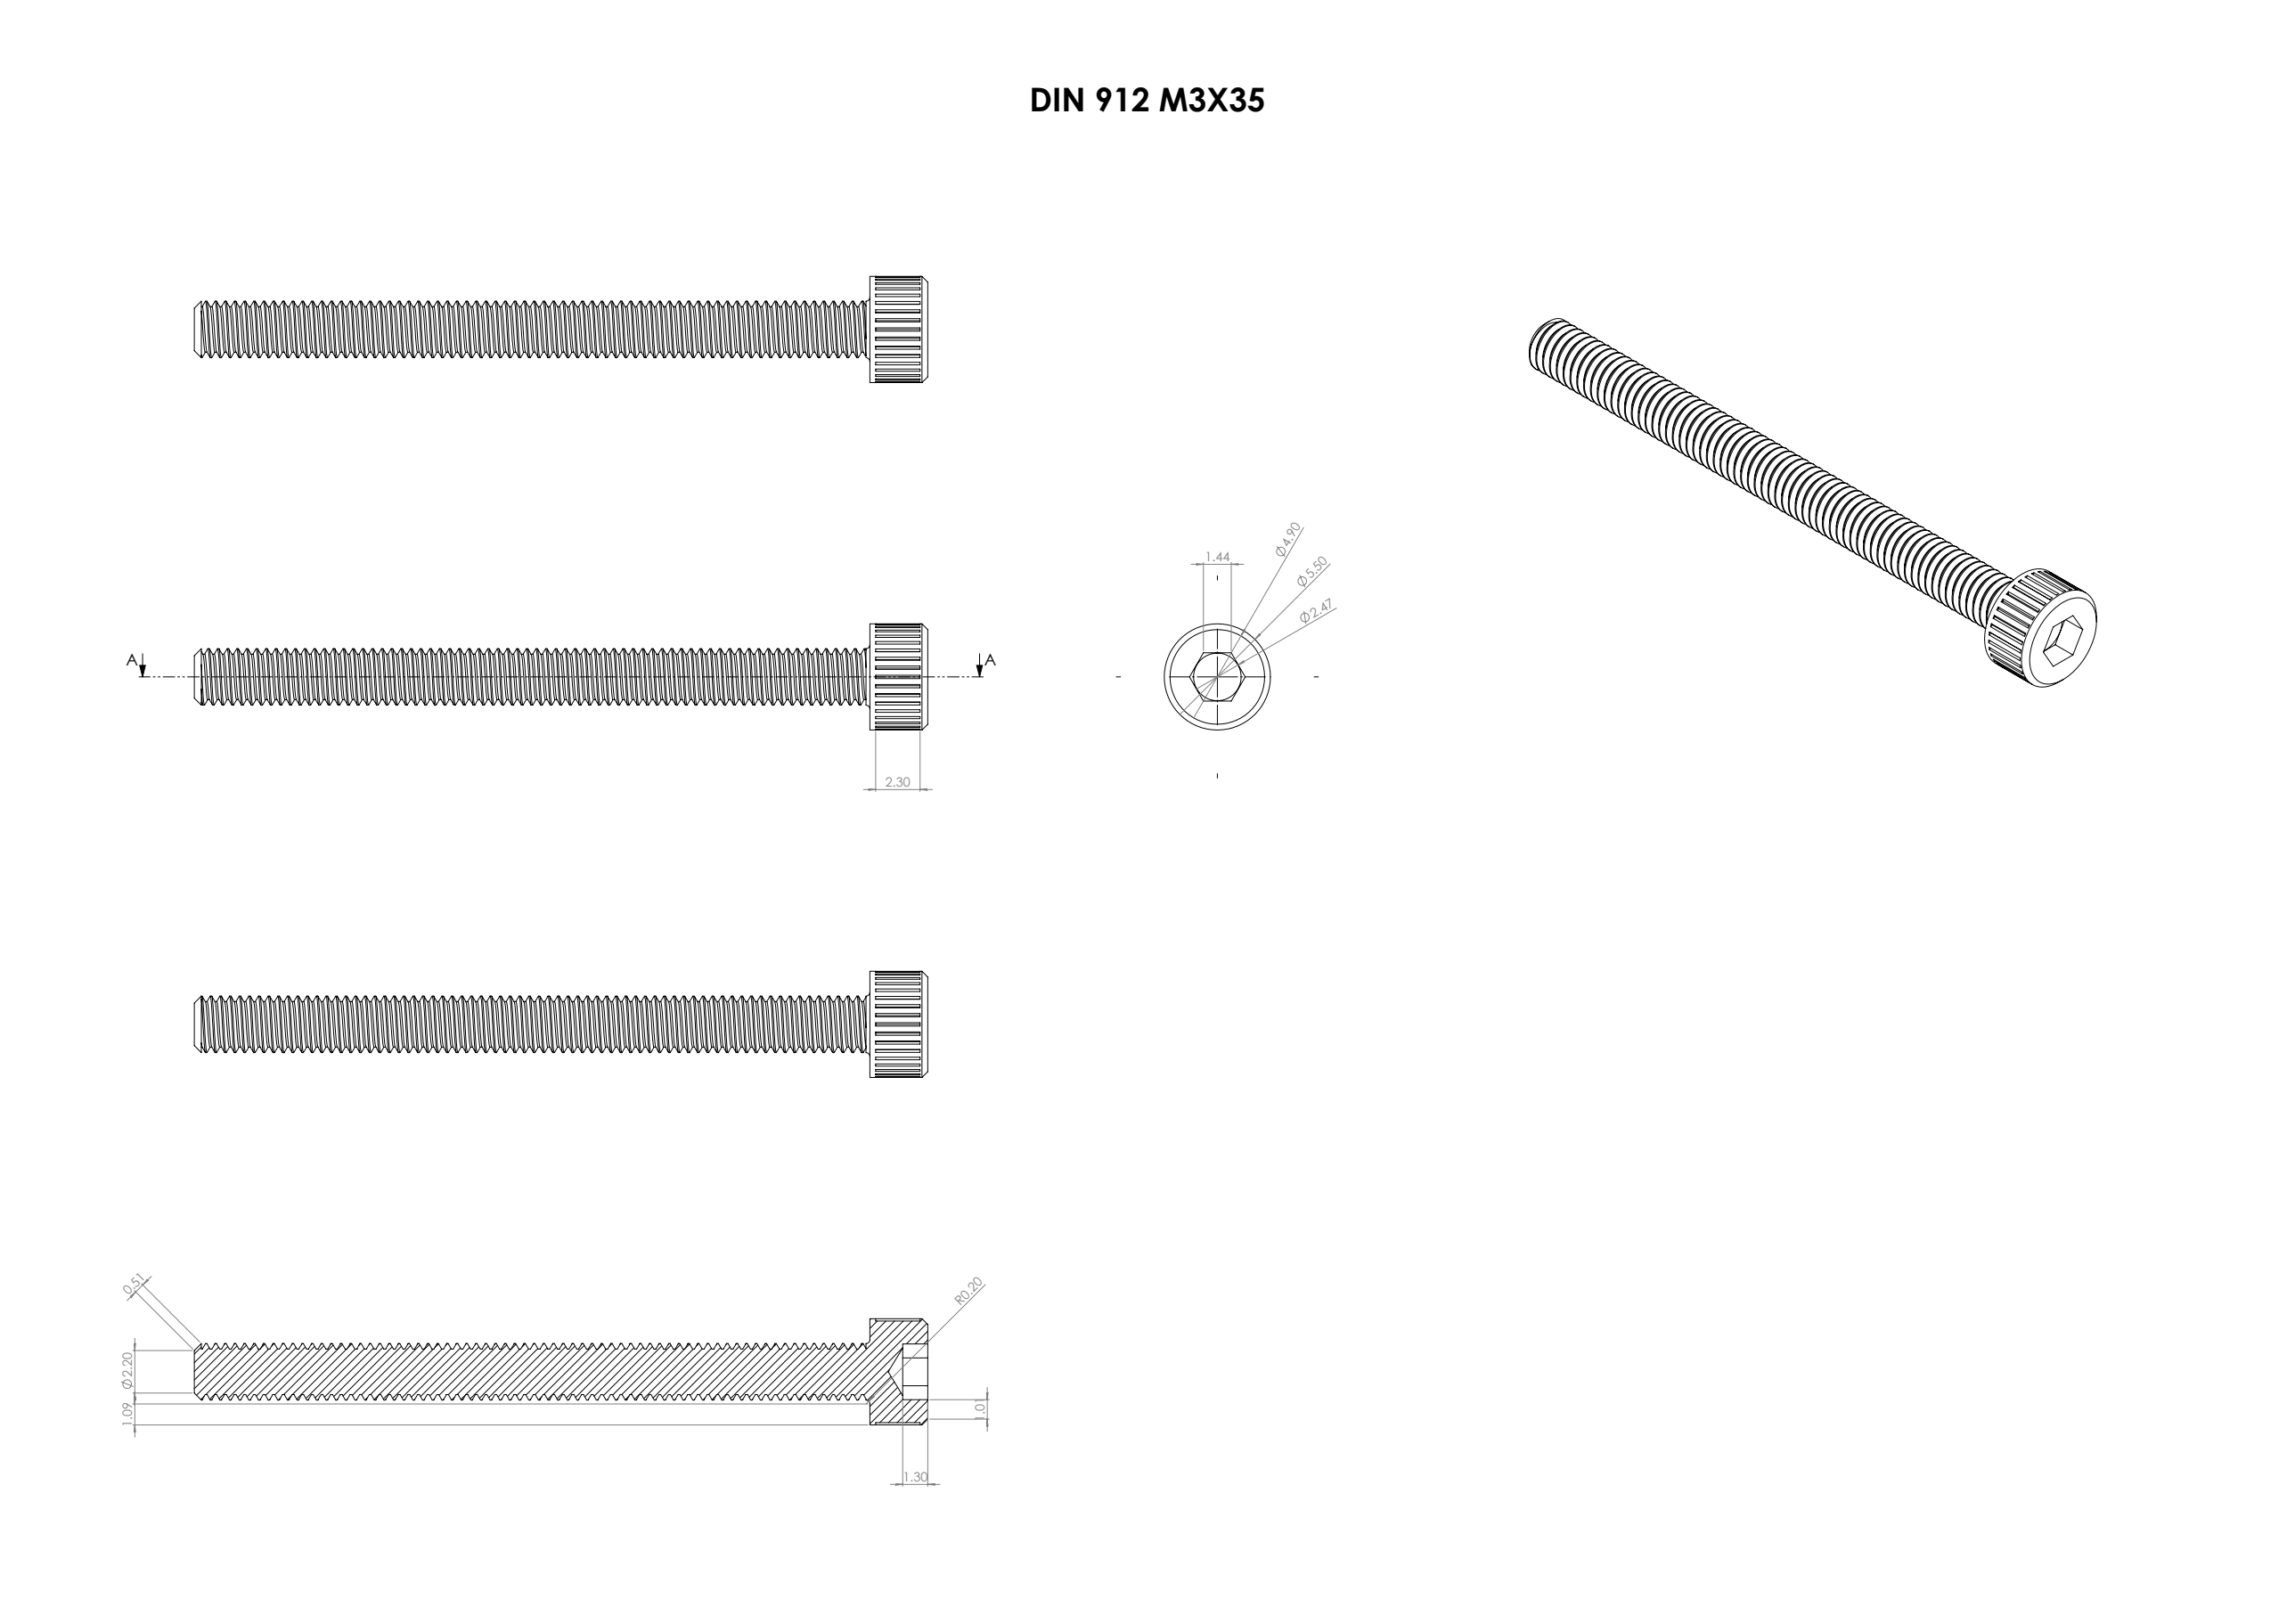
ISO-10303-21;
HEADER;
/* Generated by software containing ST-Developer
 * from STEP Tools, Inc. (www.steptools.com) 
 */

FILE_DESCRIPTION(
/* description */ (''),
/* implementation_level */ '2;1');

FILE_NAME(
/* name */ '18_DIN_912_M3x35.step',
/* time_stamp */ '2026-10-21T01:56:51-07:00',
/* author */ (''),
/* organization */ (''),
/* preprocessor_version */ 'ST-DEVELOPER v20.2',
/* originating_system */ 'Autodesk Translation Framework v15.15.0.0',
/* authorisation */ '');

FILE_SCHEMA (('AUTOMOTIVE_DESIGN { 1 0 10303 214 3 1 1 }'));
ENDSEC;

DATA;
#10=MECHANICAL_DESIGN_GEOMETRIC_PRESENTATION_REPRESENTATION('',(#283),#82384);
#161=TOROIDAL_SURFACE('',#32603,1.6635,0.2);
#245=SHAPE_REPRESENTATION_RELATIONSHIP('SRR','None',#82479,#264);
#264=ADVANCED_BREP_SHAPE_REPRESENTATION('',(#302),#82378);
#283=STYLED_ITEM('',(#82638),#302);
#302=MANIFOLD_SOLID_BREP('Body1',#30674);
#424=B_SPLINE_SURFACE_WITH_KNOTS('',3,3,((#61259,#61260,#61261,#61262,#61263,
#61264,#61265,#61266,#61267,#61268,#61269,#61270,#61271,#61272,#61273,#61274,
#61275,#61276,#61277,#61278,#61279,#61280,#61281,#61282,#61283,#61284,#61285,
#61286,#61287,#61288,#61289,#61290,#61291,#61292,#61293,#61294,#61295,#61296,
#61297,#61298,#61299,#61300,#61301,#61302,#61303,#61304,#61305,#61306,#61307,
#61308,#61309,#61310,#61311,#61312,#61313,#61314,#61315,#61316,#61317,#61318,
#61319,#61320,#61321,#61322,#61323,#61324,#61325,#61326,#61327,#61328,#61329,
#61330,#61331,#61332,#61333,#61334,#61335,#61336,#61337,#61338,#61339,#61340,
#61341,#61342,#61343,#61344,#61345,#61346,#61347,#61348,#61349,#61350,#61351,
#61352,#61353,#61354,#61355,#61356,#61357,#61358,#61359,#61360,#61361,#61362,
#61363,#61364,#61365,#61366,#61367,#61368,#61369,#61370,#61371,#61372,#61373,
#61374,#61375,#61376,#61377,#61378,#61379,#61380,#61381,#61382,#61383,#61384,
#61385,#61386,#61387,#61388,#61389,#61390,#61391,#61392,#61393,#61394,#61395,
#61396,#61397,#61398,#61399,#61400,#61401,#61402,#61403,#61404,#61405,#61406,
#61407,#61408,#61409,#61410,#61411,#61412,#61413,#61414,#61415,#61416,#61417,
#61418,#61419,#61420,#61421,#61422,#61423,#61424,#61425,#61426,#61427,#61428,
#61429,#61430,#61431,#61432,#61433,#61434,#61435,#61436,#61437,#61438,#61439,
#61440,#61441,#61442,#61443,#61444,#61445,#61446,#61447,#61448,#61449,#61450,
#61451,#61452,#61453,#61454,#61455,#61456,#61457,#61458,#61459,#61460,#61461,
#61462,#61463,#61464,#61465,#61466,#61467,#61468,#61469,#61470,#61471,#61472,
#61473,#61474,#61475,#61476,#61477,#61478,#61479,#61480,#61481,#61482,#61483,
#61484,#61485,#61486,#61487,#61488,#61489,#61490,#61491,#61492,#61493,#61494,
#61495,#61496,#61497,#61498,#61499,#61500,#61501,#61502,#61503,#61504,#61505,
#61506,#61507,#61508,#61509,#61510,#61511,#61512,#61513,#61514,#61515,#61516,
#61517,#61518,#61519,#61520,#61521,#61522,#61523,#61524,#61525,#61526,#61527,
#61528,#61529,#61530,#61531,#61532,#61533,#61534,#61535,#61536,#61537,#61538,
#61539,#61540,#61541,#61542,#61543,#61544,#61545,#61546,#61547,#61548,#61549,
#61550,#61551,#61552,#61553,#61554,#61555,#61556,#61557,#61558,#61559,#61560,
#61561,#61562,#61563,#61564,#61565,#61566,#61567,#61568,#61569,#61570,#61571,
#61572,#61573,#61574,#61575,#61576,#61577,#61578,#61579,#61580,#61581,#61582,
#61583,#61584,#61585,#61586,#61587,#61588,#61589,#61590,#61591,#61592,#61593,
#61594,#61595,#61596,#61597,#61598,#61599,#61600,#61601,#61602,#61603,#61604,
#61605,#61606,#61607,#61608,#61609,#61610,#61611,#61612,#61613,#61614,#61615,
#61616,#61617,#61618,#61619,#61620,#61621,#61622,#61623,#61624,#61625,#61626,
#61627,#61628,#61629,#61630,#61631,#61632,#61633,#61634,#61635,#61636,#61637,
#61638,#61639,#61640,#61641,#61642,#61643,#61644,#61645,#61646,#61647,#61648,
#61649,#61650,#61651,#61652,#61653,#61654,#61655,#61656,#61657,#61658,#61659,
#61660,#61661,#61662,#61663,#61664,#61665,#61666,#61667,#61668,#61669,#61670,
#61671,#61672,#61673,#61674,#61675,#61676,#61677,#61678,#61679,#61680,#61681,
#61682,#61683,#61684,#61685,#61686,#61687,#61688,#61689,#61690,#61691,#61692,
#61693,#61694,#61695,#61696),(#61697,#61698,#61699,#61700,#61701,#61702,
#61703,#61704,#61705,#61706,#61707,#61708,#61709,#61710,#61711,#61712,#61713,
#61714,#61715,#61716,#61717,#61718,#61719,#61720,#61721,#61722,#61723,#61724,
#61725,#61726,#61727,#61728,#61729,#61730,#61731,#61732,#61733,#61734,#61735,
#61736,#61737,#61738,#61739,#61740,#61741,#61742,#61743,#61744,#61745,#61746,
#61747,#61748,#61749,#61750,#61751,#61752,#61753,#61754,#61755,#61756,#61757,
#61758,#61759,#61760,#61761,#61762,#61763,#61764,#61765,#61766,#61767,#61768,
#61769,#61770,#61771,#61772,#61773,#61774,#61775,#61776,#61777,#61778,#61779,
#61780,#61781,#61782,#61783,#61784,#61785,#61786,#61787,#61788,#61789,#61790,
#61791,#61792,#61793,#61794,#61795,#61796,#61797,#61798,#61799,#61800,#61801,
#61802,#61803,#61804,#61805,#61806,#61807,#61808,#61809,#61810,#61811,#61812,
#61813,#61814,#61815,#61816,#61817,#61818,#61819,#61820,#61821,#61822,#61823,
#61824,#61825,#61826,#61827,#61828,#61829,#61830,#61831,#61832,#61833,#61834,
#61835,#61836,#61837,#61838,#61839,#61840,#61841,#61842,#61843,#61844,#61845,
#61846,#61847,#61848,#61849,#61850,#61851,#61852,#61853,#61854,#61855,#61856,
#61857,#61858,#61859,#61860,#61861,#61862,#61863,#61864,#61865,#61866,#61867,
#61868,#61869,#61870,#61871,#61872,#61873,#61874,#61875,#61876,#61877,#61878,
#61879,#61880,#61881,#61882,#61883,#61884,#61885,#61886,#61887,#61888,#61889,
#61890,#61891,#61892,#61893,#61894,#61895,#61896,#61897,#61898,#61899,#61900,
#61901,#61902,#61903,#61904,#61905,#61906,#61907,#61908,#61909,#61910,#61911,
#61912,#61913,#61914,#61915,#61916,#61917,#61918,#61919,#61920,#61921,#61922,
#61923,#61924,#61925,#61926,#61927,#61928,#61929,#61930,#61931,#61932,#61933,
#61934,#61935,#61936,#61937,#61938,#61939,#61940,#61941,#61942,#61943,#61944,
#61945,#61946,#61947,#61948,#61949,#61950,#61951,#61952,#61953,#61954,#61955,
#61956,#61957,#61958,#61959,#61960,#61961,#61962,#61963,#61964,#61965,#61966,
#61967,#61968,#61969,#61970,#61971,#61972,#61973,#61974,#61975,#61976,#61977,
#61978,#61979,#61980,#61981,#61982,#61983,#61984,#61985,#61986,#61987,#61988,
#61989,#61990,#61991,#61992,#61993,#61994,#61995,#61996,#61997,#61998,#61999,
#62000,#62001,#62002,#62003,#62004,#62005,#62006,#62007,#62008,#62009,#62010,
#62011,#62012,#62013,#62014,#62015,#62016,#62017,#62018,#62019,#62020,#62021,
#62022,#62023,#62024,#62025,#62026,#62027,#62028,#62029,#62030,#62031,#62032,
#62033,#62034,#62035,#62036,#62037,#62038,#62039,#62040,#62041,#62042,#62043,
#62044,#62045,#62046,#62047,#62048,#62049,#62050,#62051,#62052,#62053,#62054,
#62055,#62056,#62057,#62058,#62059,#62060,#62061,#62062,#62063,#62064,#62065,
#62066,#62067,#62068,#62069,#62070,#62071,#62072,#62073,#62074,#62075,#62076,
#62077,#62078,#62079,#62080,#62081,#62082,#62083,#62084,#62085,#62086,#62087,
#62088,#62089,#62090,#62091,#62092,#62093,#62094,#62095,#62096,#62097,#62098,
#62099,#62100,#62101,#62102,#62103,#62104,#62105,#62106,#62107,#62108,#62109,
#62110,#62111,#62112,#62113,#62114,#62115,#62116,#62117,#62118,#62119,#62120,
#62121,#62122,#62123,#62124,#62125,#62126,#62127,#62128,#62129,#62130,#62131,
#62132,#62133,#62134),(#62135,#62136,#62137,#62138,#62139,#62140,#62141,
#62142,#62143,#62144,#62145,#62146,#62147,#62148,#62149,#62150,#62151,#62152,
#62153,#62154,#62155,#62156,#62157,#62158,#62159,#62160,#62161,#62162,#62163,
#62164,#62165,#62166,#62167,#62168,#62169,#62170,#62171,#62172,#62173,#62174,
#62175,#62176,#62177,#62178,#62179,#62180,#62181,#62182,#62183,#62184,#62185,
#62186,#62187,#62188,#62189,#62190,#62191,#62192,#62193,#62194,#62195,#62196,
#62197,#62198,#62199,#62200,#62201,#62202,#62203,#62204,#62205,#62206,#62207,
#62208,#62209,#62210,#62211,#62212,#62213,#62214,#62215,#62216,#62217,#62218,
#62219,#62220,#62221,#62222,#62223,#62224,#62225,#62226,#62227,#62228,#62229,
#62230,#62231,#62232,#62233,#62234,#62235,#62236,#62237,#62238,#62239,#62240,
#62241,#62242,#62243,#62244,#62245,#62246,#62247,#62248,#62249,#62250,#62251,
#62252,#62253,#62254,#62255,#62256,#62257,#62258,#62259,#62260,#62261,#62262,
#62263,#62264,#62265,#62266,#62267,#62268,#62269,#62270,#62271,#62272,#62273,
#62274,#62275,#62276,#62277,#62278,#62279,#62280,#62281,#62282,#62283,#62284,
#62285,#62286,#62287,#62288,#62289,#62290,#62291,#62292,#62293,#62294,#62295,
#62296,#62297,#62298,#62299,#62300,#62301,#62302,#62303,#62304,#62305,#62306,
#62307,#62308,#62309,#62310,#62311,#62312,#62313,#62314,#62315,#62316,#62317,
#62318,#62319,#62320,#62321,#62322,#62323,#62324,#62325,#62326,#62327,#62328,
#62329,#62330,#62331,#62332,#62333,#62334,#62335,#62336,#62337,#62338,#62339,
#62340,#62341,#62342,#62343,#62344,#62345,#62346,#62347,#62348,#62349,#62350,
#62351,#62352,#62353,#62354,#62355,#62356,#62357,#62358,#62359,#62360,#62361,
#62362,#62363,#62364,#62365,#62366,#62367,#62368,#62369,#62370,#62371,#62372,
#62373,#62374,#62375,#62376,#62377,#62378,#62379,#62380,#62381,#62382,#62383,
#62384,#62385,#62386,#62387,#62388,#62389,#62390,#62391,#62392,#62393,#62394,
#62395,#62396,#62397,#62398,#62399,#62400,#62401,#62402,#62403,#62404,#62405,
#62406,#62407,#62408,#62409,#62410,#62411,#62412,#62413,#62414,#62415,#62416,
#62417,#62418,#62419,#62420,#62421,#62422,#62423,#62424,#62425,#62426,#62427,
#62428,#62429,#62430,#62431,#62432,#62433,#62434,#62435,#62436,#62437,#62438,
#62439,#62440,#62441,#62442,#62443,#62444,#62445,#62446,#62447,#62448,#62449,
#62450,#62451,#62452,#62453,#62454,#62455,#62456,#62457,#62458,#62459,#62460,
#62461,#62462,#62463,#62464,#62465,#62466,#62467,#62468,#62469,#62470,#62471,
#62472,#62473,#62474,#62475,#62476,#62477,#62478,#62479,#62480,#62481,#62482,
#62483,#62484,#62485,#62486,#62487,#62488,#62489,#62490,#62491,#62492,#62493,
#62494,#62495,#62496,#62497,#62498,#62499,#62500,#62501,#62502,#62503,#62504,
#62505,#62506,#62507,#62508,#62509,#62510,#62511,#62512,#62513,#62514,#62515,
#62516,#62517,#62518,#62519,#62520,#62521,#62522,#62523,#62524,#62525,#62526,
#62527,#62528,#62529,#62530,#62531,#62532,#62533,#62534,#62535,#62536,#62537,
#62538,#62539,#62540,#62541,#62542,#62543,#62544,#62545,#62546,#62547,#62548,
#62549,#62550,#62551,#62552,#62553,#62554,#62555,#62556,#62557,#62558,#62559,
#62560,#62561,#62562,#62563,#62564,#62565,#62566,#62567,#62568,#62569,#62570,
#62571,#62572),(#62573,#62574,#62575,#62576,#62577,#62578,#62579,#62580,
#62581,#62582,#62583,#62584,#62585,#62586,#62587,#62588,#62589,#62590,#62591,
#62592,#62593,#62594,#62595,#62596,#62597,#62598,#62599,#62600,#62601,#62602,
#62603,#62604,#62605,#62606,#62607,#62608,#62609,#62610,#62611,#62612,#62613,
#62614,#62615,#62616,#62617,#62618,#62619,#62620,#62621,#62622,#62623,#62624,
#62625,#62626,#62627,#62628,#62629,#62630,#62631,#62632,#62633,#62634,#62635,
#62636,#62637,#62638,#62639,#62640,#62641,#62642,#62643,#62644,#62645,#62646,
#62647,#62648,#62649,#62650,#62651,#62652,#62653,#62654,#62655,#62656,#62657,
#62658,#62659,#62660,#62661,#62662,#62663,#62664,#62665,#62666,#62667,#62668,
#62669,#62670,#62671,#62672,#62673,#62674,#62675,#62676,#62677,#62678,#62679,
#62680,#62681,#62682,#62683,#62684,#62685,#62686,#62687,#62688,#62689,#62690,
#62691,#62692,#62693,#62694,#62695,#62696,#62697,#62698,#62699,#62700,#62701,
#62702,#62703,#62704,#62705,#62706,#62707,#62708,#62709,#62710,#62711,#62712,
#62713,#62714,#62715,#62716,#62717,#62718,#62719,#62720,#62721,#62722,#62723,
#62724,#62725,#62726,#62727,#62728,#62729,#62730,#62731,#62732,#62733,#62734,
#62735,#62736,#62737,#62738,#62739,#62740,#62741,#62742,#62743,#62744,#62745,
#62746,#62747,#62748,#62749,#62750,#62751,#62752,#62753,#62754,#62755,#62756,
#62757,#62758,#62759,#62760,#62761,#62762,#62763,#62764,#62765,#62766,#62767,
#62768,#62769,#62770,#62771,#62772,#62773,#62774,#62775,#62776,#62777,#62778,
#62779,#62780,#62781,#62782,#62783,#62784,#62785,#62786,#62787,#62788,#62789,
#62790,#62791,#62792,#62793,#62794,#62795,#62796,#62797,#62798,#62799,#62800,
#62801,#62802,#62803,#62804,#62805,#62806,#62807,#62808,#62809,#62810,#62811,
#62812,#62813,#62814,#62815,#62816,#62817,#62818,#62819,#62820,#62821,#62822,
#62823,#62824,#62825,#62826,#62827,#62828,#62829,#62830,#62831,#62832,#62833,
#62834,#62835,#62836,#62837,#62838,#62839,#62840,#62841,#62842,#62843,#62844,
#62845,#62846,#62847,#62848,#62849,#62850,#62851,#62852,#62853,#62854,#62855,
#62856,#62857,#62858,#62859,#62860,#62861,#62862,#62863,#62864,#62865,#62866,
#62867,#62868,#62869,#62870,#62871,#62872,#62873,#62874,#62875,#62876,#62877,
#62878,#62879,#62880,#62881,#62882,#62883,#62884,#62885,#62886,#62887,#62888,
#62889,#62890,#62891,#62892,#62893,#62894,#62895,#62896,#62897,#62898,#62899,
#62900,#62901,#62902,#62903,#62904,#62905,#62906,#62907,#62908,#62909,#62910,
#62911,#62912,#62913,#62914,#62915,#62916,#62917,#62918,#62919,#62920,#62921,
#62922,#62923,#62924,#62925,#62926,#62927,#62928,#62929,#62930,#62931,#62932,
#62933,#62934,#62935,#62936,#62937,#62938,#62939,#62940,#62941,#62942,#62943,
#62944,#62945,#62946,#62947,#62948,#62949,#62950,#62951,#62952,#62953,#62954,
#62955,#62956,#62957,#62958,#62959,#62960,#62961,#62962,#62963,#62964,#62965,
#62966,#62967,#62968,#62969,#62970,#62971,#62972,#62973,#62974,#62975,#62976,
#62977,#62978,#62979,#62980,#62981,#62982,#62983,#62984,#62985,#62986,#62987,
#62988,#62989,#62990,#62991,#62992,#62993,#62994,#62995,#62996,#62997,#62998,
#62999,#63000,#63001,#63002,#63003,#63004,#63005,#63006,#63007,#63008,#63009,
#63010)),.UNSPECIFIED.,.F.,.F.,.F.,(4,4),(4,1,1,1,1,1,1,1,1,1,1,1,1,1,1,
1,1,1,1,1,1,1,1,1,1,1,1,1,1,1,1,1,1,1,1,1,1,1,1,1,1,1,1,1,1,1,1,1,1,1,1,
1,1,1,1,1,1,1,1,1,1,1,1,1,1,1,1,1,1,1,1,1,1,1,1,1,1,1,1,1,1,1,1,1,1,1,1,
1,1,1,1,1,1,1,1,1,1,1,1,1,1,1,1,1,1,1,1,1,1,1,1,1,1,1,1,1,1,1,1,1,1,1,1,
1,1,1,1,1,1,1,1,1,1,1,1,1,1,1,1,1,1,1,1,1,1,1,1,1,1,1,1,1,1,1,1,1,1,1,1,
1,1,1,1,1,1,1,1,1,1,1,1,1,1,1,1,1,1,1,1,1,1,1,1,1,1,1,1,1,1,1,1,1,1,1,1,
1,1,1,1,1,1,1,1,1,1,1,1,1,1,1,1,1,1,1,1,1,1,1,1,1,1,1,1,1,1,1,1,1,1,1,1,
1,1,1,1,1,1,1,1,1,1,1,1,1,1,1,1,1,1,1,1,1,1,1,1,1,1,1,1,1,1,1,1,1,1,1,1,
1,1,1,1,1,1,1,1,1,1,1,1,1,1,1,1,1,1,1,1,1,1,1,1,1,1,1,1,1,1,1,1,1,1,1,1,
1,1,1,1,1,1,1,1,1,1,1,1,1,1,1,1,1,1,1,1,1,1,1,1,1,1,1,1,1,1,1,1,1,1,1,1,
1,1,1,1,1,1,1,1,1,1,1,1,1,1,1,1,1,1,1,1,1,1,1,1,1,1,1,1,1,1,1,1,1,1,1,1,
1,1,1,1,1,1,1,1,1,1,1,1,1,1,1,1,1,1,1,1,1,1,1,1,1,1,1,1,1,1,1,1,1,1,1,1,
1,1,1,1,1,1,1,1,1,1,1,1,1,1,1,1,1,1,1,1,1,1,1,1,4),(0.,0.0329955678841869),
(8.30203615430915,9.30161085392915,10.3011855535492,11.3007602531692,12.3003349527892,
13.2999096524091,14.2994843520291,15.2990590516491,16.2986337512691,17.2982084508891,
18.2977831505091,19.2973578501291,20.2969325497491,21.2965072493691,22.2960819489891,
23.2956566486091,24.2952313482291,25.2948060478491,26.2943807474691,27.2939554470891,
28.2935301467091,29.2931048463291,30.2926795459491,31.2922542455691,32.2918289451891,
33.2914036448091,34.2909783444291,35.2905530440491,36.2901277436691,37.2897024432891,
38.2892771429091,39.2888518425291,40.2884265421491,41.2880012417691,42.2875759413891,
43.2871506410091,44.2867253406291,45.2863000402491,46.2858747398691,47.2854494394891,
48.2850241391091,49.2845988387291,50.2841735383491,51.2837482379691,52.2833229375891,
53.2828976372091,54.2824723368291,55.2820470364491,56.2816217360691,57.2811964356891,
58.2807711353091,59.2803458349291,60.2799205345491,61.2794952341691,62.2790699337891,
63.2786446334091,64.2782193330291,65.2777940326491,66.2773687322691,67.2769434318891,
68.2765181315091,69.2760928311291,70.2756675307491,71.2752422303691,72.2748169299891,
73.2743916296091,74.2739663292291,75.2735410288491,76.2731157284691,77.2726904280891,
78.2722651277091,79.2718398273291,80.2714145269491,81.2709892265691,82.2705639261891,
83.2701386258091,84.2697133254291,85.2692880250491,86.2688627246691,87.2684374242891,
88.2680121239091,89.2675868235291,90.2671615231491,91.2667362227691,92.2663109223891,
93.2658856220091,94.265460321629,95.265035021249,96.264609720869,97.264184420489,
98.2637591201091,99.2633338197291,100.262908519349,101.262483218969,102.262057918589,
103.261632618209,104.261207317829,105.260782017449,106.260356717069,107.259931416689,
108.259506116309,109.259080815929,110.258655515549,111.258230215169,112.257804914789,
113.257379614409,114.256954314029,115.256529013649,116.256103713269,117.255678412889,
118.255253112509,119.254827812129,120.254402511749,121.253977211369,122.253551910989,
123.253126610609,124.252701310229,125.252276009849,126.251850709469,127.251425409089,
128.251000108709,129.250574808329,130.250149507949,131.249724207569,132.249298907189,
133.248873606809,134.248448306429,135.248023006049,136.247597705669,137.247172405289,
138.246747104909,139.246321804529,140.245896504149,141.245471203769,142.245045903389,
143.244620603009,144.244195302629,145.243770002249,146.243344701869,147.242919401489,
148.242494101109,149.242068800729,150.241643500349,151.241218199969,152.240792899589,
153.240367599209,154.239942298829,155.239516998449,156.239091698069,157.238666397689,
158.238241097309,159.237815796929,160.237390496549,161.236965196169,162.236539895789,
163.236114595409,164.235689295029,165.235263994649,166.234838694269,167.234413393889,
168.233988093509,169.233562793129,170.233137492749,171.232712192369,172.232286891989,
173.231861591609,174.231436291229,175.231010990849,176.230585690469,177.230160390089,
178.229735089709,179.229309789329,180.228884488949,181.228459188569,182.228033888189,
183.227608587809,184.227183287429,185.226757987049,186.226332686669,187.225907386289,
188.225482085909,189.225056785529,190.224631485149,191.224206184769,192.223780884389,
193.223355584009,194.222930283629,195.222504983249,196.222079682869,197.221654382489,
198.221229082109,199.220803781729,200.220378481349,201.219953180969,202.219527880589,
203.219102580209,204.218677279829,205.218251979449,206.217826679069,207.217401378689,
208.216976078309,209.216550777929,210.216125477549,211.215700177169,212.215274876789,
213.214849576409,214.214424276029,215.213998975649,216.213573675269,217.213148374889,
218.212723074509,219.212297774129,220.211872473749,221.211447173369,222.211021872989,
223.210596572609,224.210171272229,225.209745971849,226.209320671469,227.208895371089,
228.208470070709,229.208044770329,230.207619469949,231.207194169569,232.206768869189,
233.206343568809,234.205918268429,235.205492968049,236.205067667669,237.204642367289,
238.204217066909,239.203791766529,240.203366466149,241.202941165769,242.202515865389,
243.202090565009,244.201665264629,245.201239964249,246.200814663869,247.200389363489,
248.199964063109,249.199538762729,250.199113462349,251.198688161969,252.198262861589,
253.197837561209,254.197412260829,255.196986960449,256.196561660069,257.196136359689,
258.195711059309,259.195285758929,260.194860458549,261.194435158169,262.194009857789,
263.193584557409,264.193159257029,265.192733956649,266.192308656269,267.191883355889,
268.191458055509,269.191032755129,270.190607454749,271.190182154369,272.189756853989,
273.189331553609,274.188906253229,275.188480952849,276.188055652469,277.187630352089,
278.187205051709,279.186779751329,280.186354450949,281.185929150569,282.185503850189,
283.185078549809,284.184653249429,285.184227949049,286.183802648669,287.183377348289,
288.182952047909,289.182526747529,290.182101447149,291.181676146769,292.181250846389,
293.180825546009,294.180400245629,295.179974945249,296.179549644869,297.179124344489,
298.178699044109,299.178273743729,300.177848443349,301.177423142969,302.176997842589,
303.176572542209,304.176147241829,305.175721941449,306.175296641069,307.174871340689,
308.174446040309,309.174020739929,310.173595439549,311.173170139169,312.172744838789,
313.172319538409,314.171894238029,315.171468937649,316.171043637269,317.170618336889,
318.170193036509,319.169767736129,320.169342435749,321.168917135369,322.168491834989,
323.168066534609,324.167641234229,325.167215933849,326.166790633469,327.166365333089,
328.165940032709,329.165514732329,330.165089431949,331.164664131569,332.164238831189,
333.163813530809,334.163388230429,335.162962930049,336.162537629669,337.162112329289,
338.161687028909,339.161261728529,340.160836428149,341.160411127769,342.159985827389,
343.159560527009,344.159135226629,345.158709926249,346.158284625869,347.157859325489,
348.157434025109,349.157008724729,350.156583424349,351.156158123969,352.155732823589,
353.155307523209,354.154882222829,355.154456922449,356.154031622069,357.153606321689,
358.153181021309,359.152755720929,360.152330420549,361.151905120169,362.151479819789,
363.151054519409,364.150629219029,365.150203918649,366.149778618269,367.149353317889,
368.148928017509,369.148502717129,370.148077416749,371.147652116369,372.147226815989,
373.146801515609,374.146376215229,375.145950914849,376.145525614469,377.145100314089,
378.144675013709,379.144249713329,380.143824412949,381.143399112569,382.142973812189,
383.142548511809,384.142123211429,385.141697911049,386.141272610669,387.140847310289,
388.140422009909,389.139996709529,390.139571409149,391.139146108769,392.138720808389,
393.138295508009,394.137870207629,395.137444907249,396.137019606869,397.136594306489,
398.136169006109,399.135743705729,400.135318405349,401.134893104969,402.134467804589,
403.134042504209,404.133617203829,405.133191903449,406.132766603069,407.132341302689,
408.131916002309,409.131490701929,410.131065401549,411.130640101169,412.130214800789,
413.129789500409,414.129364200029,415.128938899649,416.128513599269,417.128088298889,
418.127662998509,419.127237698129,420.126812397749,421.126387097369,422.125961796989,
423.125536496609,424.125111196229,425.124685895849,426.124260595469,427.123835295089,
428.123409994709,429.122984694329,430.122559393949,431.122134093569,432.121708793189,
433.121283492809,434.120858192429,435.120432892049,436.120007591669,437.119582291289,
438.119156990909,439.118731690529,440.118306390149,441.117881089769,442.117455789389,
443.117030489009),.UNSPECIFIED.);
#425=B_SPLINE_SURFACE_WITH_KNOTS('',3,3,((#63219,#63220,#63221,#63222,#63223,
#63224,#63225,#63226,#63227,#63228,#63229,#63230,#63231,#63232,#63233,#63234,
#63235,#63236,#63237,#63238,#63239,#63240,#63241,#63242,#63243,#63244,#63245,
#63246,#63247,#63248,#63249,#63250,#63251,#63252,#63253,#63254,#63255,#63256,
#63257,#63258,#63259,#63260,#63261,#63262,#63263,#63264,#63265,#63266,#63267,
#63268,#63269,#63270,#63271,#63272,#63273,#63274,#63275,#63276,#63277,#63278,
#63279,#63280,#63281,#63282,#63283,#63284,#63285,#63286,#63287,#63288,#63289,
#63290,#63291,#63292,#63293,#63294,#63295,#63296,#63297,#63298,#63299,#63300,
#63301,#63302,#63303,#63304,#63305,#63306,#63307,#63308,#63309,#63310,#63311,
#63312,#63313,#63314,#63315,#63316,#63317,#63318,#63319,#63320,#63321,#63322,
#63323,#63324,#63325,#63326,#63327,#63328,#63329,#63330,#63331,#63332,#63333,
#63334,#63335,#63336,#63337,#63338,#63339,#63340,#63341,#63342,#63343,#63344,
#63345,#63346,#63347,#63348,#63349,#63350,#63351,#63352,#63353,#63354,#63355,
#63356,#63357,#63358,#63359,#63360,#63361,#63362,#63363,#63364,#63365,#63366,
#63367,#63368,#63369,#63370,#63371,#63372,#63373,#63374,#63375,#63376,#63377,
#63378,#63379,#63380,#63381,#63382,#63383,#63384,#63385,#63386,#63387,#63388,
#63389,#63390,#63391,#63392,#63393,#63394,#63395,#63396,#63397,#63398,#63399,
#63400,#63401,#63402,#63403,#63404,#63405,#63406,#63407,#63408,#63409,#63410,
#63411,#63412,#63413,#63414,#63415,#63416,#63417,#63418,#63419,#63420,#63421,
#63422,#63423,#63424,#63425,#63426,#63427,#63428,#63429,#63430,#63431,#63432,
#63433,#63434,#63435,#63436,#63437,#63438,#63439,#63440,#63441,#63442,#63443,
#63444,#63445,#63446,#63447,#63448,#63449,#63450,#63451,#63452,#63453,#63454,
#63455,#63456,#63457,#63458,#63459,#63460,#63461,#63462,#63463,#63464,#63465,
#63466,#63467,#63468,#63469,#63470,#63471,#63472,#63473,#63474,#63475,#63476,
#63477,#63478,#63479,#63480,#63481,#63482,#63483,#63484,#63485,#63486,#63487,
#63488,#63489,#63490,#63491,#63492,#63493,#63494,#63495,#63496,#63497,#63498,
#63499,#63500,#63501,#63502,#63503,#63504,#63505,#63506,#63507,#63508,#63509,
#63510,#63511,#63512,#63513,#63514,#63515,#63516,#63517,#63518,#63519,#63520,
#63521,#63522,#63523,#63524,#63525,#63526,#63527,#63528,#63529,#63530,#63531,
#63532,#63533,#63534,#63535,#63536,#63537,#63538,#63539,#63540,#63541,#63542,
#63543,#63544,#63545,#63546,#63547,#63548,#63549,#63550,#63551,#63552,#63553,
#63554,#63555,#63556,#63557,#63558,#63559,#63560,#63561,#63562,#63563,#63564,
#63565,#63566,#63567,#63568,#63569,#63570,#63571,#63572,#63573,#63574,#63575,
#63576,#63577,#63578,#63579,#63580,#63581,#63582,#63583,#63584,#63585,#63586,
#63587,#63588,#63589,#63590,#63591,#63592,#63593,#63594,#63595,#63596,#63597,
#63598,#63599,#63600,#63601,#63602,#63603,#63604,#63605,#63606,#63607,#63608,
#63609,#63610,#63611,#63612,#63613,#63614,#63615,#63616,#63617,#63618,#63619,
#63620,#63621,#63622,#63623,#63624,#63625,#63626,#63627,#63628,#63629,#63630,
#63631,#63632,#63633,#63634,#63635,#63636,#63637,#63638,#63639,#63640,#63641,
#63642,#63643,#63644,#63645,#63646,#63647,#63648,#63649,#63650,#63651,#63652,
#63653,#63654,#63655,#63656),(#63657,#63658,#63659,#63660,#63661,#63662,
#63663,#63664,#63665,#63666,#63667,#63668,#63669,#63670,#63671,#63672,#63673,
#63674,#63675,#63676,#63677,#63678,#63679,#63680,#63681,#63682,#63683,#63684,
#63685,#63686,#63687,#63688,#63689,#63690,#63691,#63692,#63693,#63694,#63695,
#63696,#63697,#63698,#63699,#63700,#63701,#63702,#63703,#63704,#63705,#63706,
#63707,#63708,#63709,#63710,#63711,#63712,#63713,#63714,#63715,#63716,#63717,
#63718,#63719,#63720,#63721,#63722,#63723,#63724,#63725,#63726,#63727,#63728,
#63729,#63730,#63731,#63732,#63733,#63734,#63735,#63736,#63737,#63738,#63739,
#63740,#63741,#63742,#63743,#63744,#63745,#63746,#63747,#63748,#63749,#63750,
#63751,#63752,#63753,#63754,#63755,#63756,#63757,#63758,#63759,#63760,#63761,
#63762,#63763,#63764,#63765,#63766,#63767,#63768,#63769,#63770,#63771,#63772,
#63773,#63774,#63775,#63776,#63777,#63778,#63779,#63780,#63781,#63782,#63783,
#63784,#63785,#63786,#63787,#63788,#63789,#63790,#63791,#63792,#63793,#63794,
#63795,#63796,#63797,#63798,#63799,#63800,#63801,#63802,#63803,#63804,#63805,
#63806,#63807,#63808,#63809,#63810,#63811,#63812,#63813,#63814,#63815,#63816,
#63817,#63818,#63819,#63820,#63821,#63822,#63823,#63824,#63825,#63826,#63827,
#63828,#63829,#63830,#63831,#63832,#63833,#63834,#63835,#63836,#63837,#63838,
#63839,#63840,#63841,#63842,#63843,#63844,#63845,#63846,#63847,#63848,#63849,
#63850,#63851,#63852,#63853,#63854,#63855,#63856,#63857,#63858,#63859,#63860,
#63861,#63862,#63863,#63864,#63865,#63866,#63867,#63868,#63869,#63870,#63871,
#63872,#63873,#63874,#63875,#63876,#63877,#63878,#63879,#63880,#63881,#63882,
#63883,#63884,#63885,#63886,#63887,#63888,#63889,#63890,#63891,#63892,#63893,
#63894,#63895,#63896,#63897,#63898,#63899,#63900,#63901,#63902,#63903,#63904,
#63905,#63906,#63907,#63908,#63909,#63910,#63911,#63912,#63913,#63914,#63915,
#63916,#63917,#63918,#63919,#63920,#63921,#63922,#63923,#63924,#63925,#63926,
#63927,#63928,#63929,#63930,#63931,#63932,#63933,#63934,#63935,#63936,#63937,
#63938,#63939,#63940,#63941,#63942,#63943,#63944,#63945,#63946,#63947,#63948,
#63949,#63950,#63951,#63952,#63953,#63954,#63955,#63956,#63957,#63958,#63959,
#63960,#63961,#63962,#63963,#63964,#63965,#63966,#63967,#63968,#63969,#63970,
#63971,#63972,#63973,#63974,#63975,#63976,#63977,#63978,#63979,#63980,#63981,
#63982,#63983,#63984,#63985,#63986,#63987,#63988,#63989,#63990,#63991,#63992,
#63993,#63994,#63995,#63996,#63997,#63998,#63999,#64000,#64001,#64002,#64003,
#64004,#64005,#64006,#64007,#64008,#64009,#64010,#64011,#64012,#64013,#64014,
#64015,#64016,#64017,#64018,#64019,#64020,#64021,#64022,#64023,#64024,#64025,
#64026,#64027,#64028,#64029,#64030,#64031,#64032,#64033,#64034,#64035,#64036,
#64037,#64038,#64039,#64040,#64041,#64042,#64043,#64044,#64045,#64046,#64047,
#64048,#64049,#64050,#64051,#64052,#64053,#64054,#64055,#64056,#64057,#64058,
#64059,#64060,#64061,#64062,#64063,#64064,#64065,#64066,#64067,#64068,#64069,
#64070,#64071,#64072,#64073,#64074,#64075,#64076,#64077,#64078,#64079,#64080,
#64081,#64082,#64083,#64084,#64085,#64086,#64087,#64088,#64089,#64090,#64091,
#64092,#64093,#64094),(#64095,#64096,#64097,#64098,#64099,#64100,#64101,
#64102,#64103,#64104,#64105,#64106,#64107,#64108,#64109,#64110,#64111,#64112,
#64113,#64114,#64115,#64116,#64117,#64118,#64119,#64120,#64121,#64122,#64123,
#64124,#64125,#64126,#64127,#64128,#64129,#64130,#64131,#64132,#64133,#64134,
#64135,#64136,#64137,#64138,#64139,#64140,#64141,#64142,#64143,#64144,#64145,
#64146,#64147,#64148,#64149,#64150,#64151,#64152,#64153,#64154,#64155,#64156,
#64157,#64158,#64159,#64160,#64161,#64162,#64163,#64164,#64165,#64166,#64167,
#64168,#64169,#64170,#64171,#64172,#64173,#64174,#64175,#64176,#64177,#64178,
#64179,#64180,#64181,#64182,#64183,#64184,#64185,#64186,#64187,#64188,#64189,
#64190,#64191,#64192,#64193,#64194,#64195,#64196,#64197,#64198,#64199,#64200,
#64201,#64202,#64203,#64204,#64205,#64206,#64207,#64208,#64209,#64210,#64211,
#64212,#64213,#64214,#64215,#64216,#64217,#64218,#64219,#64220,#64221,#64222,
#64223,#64224,#64225,#64226,#64227,#64228,#64229,#64230,#64231,#64232,#64233,
#64234,#64235,#64236,#64237,#64238,#64239,#64240,#64241,#64242,#64243,#64244,
#64245,#64246,#64247,#64248,#64249,#64250,#64251,#64252,#64253,#64254,#64255,
#64256,#64257,#64258,#64259,#64260,#64261,#64262,#64263,#64264,#64265,#64266,
#64267,#64268,#64269,#64270,#64271,#64272,#64273,#64274,#64275,#64276,#64277,
#64278,#64279,#64280,#64281,#64282,#64283,#64284,#64285,#64286,#64287,#64288,
#64289,#64290,#64291,#64292,#64293,#64294,#64295,#64296,#64297,#64298,#64299,
#64300,#64301,#64302,#64303,#64304,#64305,#64306,#64307,#64308,#64309,#64310,
#64311,#64312,#64313,#64314,#64315,#64316,#64317,#64318,#64319,#64320,#64321,
#64322,#64323,#64324,#64325,#64326,#64327,#64328,#64329,#64330,#64331,#64332,
#64333,#64334,#64335,#64336,#64337,#64338,#64339,#64340,#64341,#64342,#64343,
#64344,#64345,#64346,#64347,#64348,#64349,#64350,#64351,#64352,#64353,#64354,
#64355,#64356,#64357,#64358,#64359,#64360,#64361,#64362,#64363,#64364,#64365,
#64366,#64367,#64368,#64369,#64370,#64371,#64372,#64373,#64374,#64375,#64376,
#64377,#64378,#64379,#64380,#64381,#64382,#64383,#64384,#64385,#64386,#64387,
#64388,#64389,#64390,#64391,#64392,#64393,#64394,#64395,#64396,#64397,#64398,
#64399,#64400,#64401,#64402,#64403,#64404,#64405,#64406,#64407,#64408,#64409,
#64410,#64411,#64412,#64413,#64414,#64415,#64416,#64417,#64418,#64419,#64420,
#64421,#64422,#64423,#64424,#64425,#64426,#64427,#64428,#64429,#64430,#64431,
#64432,#64433,#64434,#64435,#64436,#64437,#64438,#64439,#64440,#64441,#64442,
#64443,#64444,#64445,#64446,#64447,#64448,#64449,#64450,#64451,#64452,#64453,
#64454,#64455,#64456,#64457,#64458,#64459,#64460,#64461,#64462,#64463,#64464,
#64465,#64466,#64467,#64468,#64469,#64470,#64471,#64472,#64473,#64474,#64475,
#64476,#64477,#64478,#64479,#64480,#64481,#64482,#64483,#64484,#64485,#64486,
#64487,#64488,#64489,#64490,#64491,#64492,#64493,#64494,#64495,#64496,#64497,
#64498,#64499,#64500,#64501,#64502,#64503,#64504,#64505,#64506,#64507,#64508,
#64509,#64510,#64511,#64512,#64513,#64514,#64515,#64516,#64517,#64518,#64519,
#64520,#64521,#64522,#64523,#64524,#64525,#64526,#64527,#64528,#64529,#64530,
#64531,#64532),(#64533,#64534,#64535,#64536,#64537,#64538,#64539,#64540,
#64541,#64542,#64543,#64544,#64545,#64546,#64547,#64548,#64549,#64550,#64551,
#64552,#64553,#64554,#64555,#64556,#64557,#64558,#64559,#64560,#64561,#64562,
#64563,#64564,#64565,#64566,#64567,#64568,#64569,#64570,#64571,#64572,#64573,
#64574,#64575,#64576,#64577,#64578,#64579,#64580,#64581,#64582,#64583,#64584,
#64585,#64586,#64587,#64588,#64589,#64590,#64591,#64592,#64593,#64594,#64595,
#64596,#64597,#64598,#64599,#64600,#64601,#64602,#64603,#64604,#64605,#64606,
#64607,#64608,#64609,#64610,#64611,#64612,#64613,#64614,#64615,#64616,#64617,
#64618,#64619,#64620,#64621,#64622,#64623,#64624,#64625,#64626,#64627,#64628,
#64629,#64630,#64631,#64632,#64633,#64634,#64635,#64636,#64637,#64638,#64639,
#64640,#64641,#64642,#64643,#64644,#64645,#64646,#64647,#64648,#64649,#64650,
#64651,#64652,#64653,#64654,#64655,#64656,#64657,#64658,#64659,#64660,#64661,
#64662,#64663,#64664,#64665,#64666,#64667,#64668,#64669,#64670,#64671,#64672,
#64673,#64674,#64675,#64676,#64677,#64678,#64679,#64680,#64681,#64682,#64683,
#64684,#64685,#64686,#64687,#64688,#64689,#64690,#64691,#64692,#64693,#64694,
#64695,#64696,#64697,#64698,#64699,#64700,#64701,#64702,#64703,#64704,#64705,
#64706,#64707,#64708,#64709,#64710,#64711,#64712,#64713,#64714,#64715,#64716,
#64717,#64718,#64719,#64720,#64721,#64722,#64723,#64724,#64725,#64726,#64727,
#64728,#64729,#64730,#64731,#64732,#64733,#64734,#64735,#64736,#64737,#64738,
#64739,#64740,#64741,#64742,#64743,#64744,#64745,#64746,#64747,#64748,#64749,
#64750,#64751,#64752,#64753,#64754,#64755,#64756,#64757,#64758,#64759,#64760,
#64761,#64762,#64763,#64764,#64765,#64766,#64767,#64768,#64769,#64770,#64771,
#64772,#64773,#64774,#64775,#64776,#64777,#64778,#64779,#64780,#64781,#64782,
#64783,#64784,#64785,#64786,#64787,#64788,#64789,#64790,#64791,#64792,#64793,
#64794,#64795,#64796,#64797,#64798,#64799,#64800,#64801,#64802,#64803,#64804,
#64805,#64806,#64807,#64808,#64809,#64810,#64811,#64812,#64813,#64814,#64815,
#64816,#64817,#64818,#64819,#64820,#64821,#64822,#64823,#64824,#64825,#64826,
#64827,#64828,#64829,#64830,#64831,#64832,#64833,#64834,#64835,#64836,#64837,
#64838,#64839,#64840,#64841,#64842,#64843,#64844,#64845,#64846,#64847,#64848,
#64849,#64850,#64851,#64852,#64853,#64854,#64855,#64856,#64857,#64858,#64859,
#64860,#64861,#64862,#64863,#64864,#64865,#64866,#64867,#64868,#64869,#64870,
#64871,#64872,#64873,#64874,#64875,#64876,#64877,#64878,#64879,#64880,#64881,
#64882,#64883,#64884,#64885,#64886,#64887,#64888,#64889,#64890,#64891,#64892,
#64893,#64894,#64895,#64896,#64897,#64898,#64899,#64900,#64901,#64902,#64903,
#64904,#64905,#64906,#64907,#64908,#64909,#64910,#64911,#64912,#64913,#64914,
#64915,#64916,#64917,#64918,#64919,#64920,#64921,#64922,#64923,#64924,#64925,
#64926,#64927,#64928,#64929,#64930,#64931,#64932,#64933,#64934,#64935,#64936,
#64937,#64938,#64939,#64940,#64941,#64942,#64943,#64944,#64945,#64946,#64947,
#64948,#64949,#64950,#64951,#64952,#64953,#64954,#64955,#64956,#64957,#64958,
#64959,#64960,#64961,#64962,#64963,#64964,#64965,#64966,#64967,#64968,#64969,
#64970)),.UNSPECIFIED.,.F.,.F.,.F.,(4,4),(4,1,1,1,1,1,1,1,1,1,1,1,1,1,1,
1,1,1,1,1,1,1,1,1,1,1,1,1,1,1,1,1,1,1,1,1,1,1,1,1,1,1,1,1,1,1,1,1,1,1,1,
1,1,1,1,1,1,1,1,1,1,1,1,1,1,1,1,1,1,1,1,1,1,1,1,1,1,1,1,1,1,1,1,1,1,1,1,
1,1,1,1,1,1,1,1,1,1,1,1,1,1,1,1,1,1,1,1,1,1,1,1,1,1,1,1,1,1,1,1,1,1,1,1,
1,1,1,1,1,1,1,1,1,1,1,1,1,1,1,1,1,1,1,1,1,1,1,1,1,1,1,1,1,1,1,1,1,1,1,1,
1,1,1,1,1,1,1,1,1,1,1,1,1,1,1,1,1,1,1,1,1,1,1,1,1,1,1,1,1,1,1,1,1,1,1,1,
1,1,1,1,1,1,1,1,1,1,1,1,1,1,1,1,1,1,1,1,1,1,1,1,1,1,1,1,1,1,1,1,1,1,1,1,
1,1,1,1,1,1,1,1,1,1,1,1,1,1,1,1,1,1,1,1,1,1,1,1,1,1,1,1,1,1,1,1,1,1,1,1,
1,1,1,1,1,1,1,1,1,1,1,1,1,1,1,1,1,1,1,1,1,1,1,1,1,1,1,1,1,1,1,1,1,1,1,1,
1,1,1,1,1,1,1,1,1,1,1,1,1,1,1,1,1,1,1,1,1,1,1,1,1,1,1,1,1,1,1,1,1,1,1,1,
1,1,1,1,1,1,1,1,1,1,1,1,1,1,1,1,1,1,1,1,1,1,1,1,1,1,1,1,1,1,1,1,1,1,1,1,
1,1,1,1,1,1,1,1,1,1,1,1,1,1,1,1,1,1,1,1,1,1,1,1,1,1,1,1,1,1,1,1,1,1,1,1,
1,1,1,1,1,1,1,1,1,1,1,1,1,1,1,1,1,1,1,1,1,1,1,1,4),(0.,0.0329955678841869),
(11.6159397475014,12.6155144471214,13.6150891467414,14.6146638463614,15.6142385459814,
16.6138132456014,17.6133879452214,18.6129626448414,19.6125373444614,20.6121120440814,
21.6116867437014,22.6112614433214,23.6108361429414,24.6104108425614,25.6099855421814,
26.6095602418014,27.6091349414214,28.6087096410414,29.6082843406614,30.6078590402814,
31.6074337399014,32.6070084395214,33.6065831391414,34.6061578387614,35.6057325383814,
36.6053072380014,37.6048819376214,38.6044566372414,39.6040313368614,40.6036060364814,
41.6031807361014,42.6027554357214,43.6023301353414,44.6019048349614,45.6014795345814,
46.6010542342014,47.6006289338214,48.6002036334414,49.5997783330614,50.5993530326813,
51.5989277323013,52.5985024319213,53.5980771315413,54.5976518311613,55.5972265307813,
56.5968012304013,57.5963759300213,58.5959506296413,59.5955253292613,60.5951000288813,
61.5946747285013,62.5942494281213,63.5938241277413,64.5933988273613,65.5929735269813,
66.5925482266013,67.5921229262213,68.5916976258413,69.5912723254613,70.5908470250813,
71.5904217247013,72.5899964243213,73.5895711239413,74.5891458235613,75.5887205231813,
76.5882952228013,77.5878699224213,78.5874446220413,79.5870193216613,80.5865940212813,
81.5861687209013,82.5857434205213,83.5853181201413,84.5848928197613,85.5844675193813,
86.5840422190013,87.5836169186213,88.5831916182413,89.5827663178613,90.5823410174813,
91.5819157171013,92.5814904167213,93.5810651163413,94.5806398159613,95.5802145155813,
96.5797892152013,97.5793639148213,98.5789386144413,99.5785133140613,100.578088013681,
101.577662713301,102.577237412921,103.576812112541,104.576386812161,105.575961511781,
106.575536211401,107.575110911021,108.574685610641,109.574260310261,110.573835009881,
111.573409709501,112.572984409121,113.572559108741,114.572133808361,115.571708507981,
116.571283207601,117.570857907221,118.570432606841,119.570007306461,120.569582006081,
121.569156705701,122.568731405321,123.568306104941,124.567880804561,125.567455504181,
126.567030203801,127.566604903421,128.566179603041,129.565754302661,130.565329002281,
131.564903701901,132.564478401521,133.564053101141,134.563627800761,135.563202500381,
136.562777200001,137.562351899621,138.561926599241,139.561501298861,140.561075998481,
141.560650698101,142.560225397721,143.559800097341,144.559374796961,145.558949496581,
146.558524196201,147.558098895821,148.557673595441,149.557248295061,150.556822994681,
151.556397694301,152.555972393921,153.555547093541,154.555121793161,155.554696492781,
156.554271192401,157.553845892021,158.553420591641,159.552995291261,160.552569990881,
161.552144690501,162.551719390121,163.551294089741,164.550868789361,165.550443488981,
166.550018188601,167.549592888221,168.549167587841,169.548742287461,170.548316987081,
171.547891686701,172.547466386321,173.547041085941,174.546615785561,175.546190485181,
176.545765184801,177.545339884421,178.544914584041,179.544489283661,180.544063983281,
181.543638682901,182.543213382521,183.542788082141,184.542362781761,185.541937481381,
186.541512181001,187.541086880621,188.540661580241,189.540236279861,190.539810979481,
191.539385679101,192.538960378721,193.538535078341,194.538109777961,195.537684477581,
196.537259177201,197.536833876821,198.536408576441,199.535983276061,200.535557975681,
201.535132675301,202.534707374921,203.534282074541,204.533856774161,205.533431473781,
206.533006173401,207.532580873021,208.532155572641,209.531730272261,210.531304971881,
211.530879671501,212.530454371121,213.530029070741,214.529603770361,215.529178469981,
216.528753169601,217.528327869221,218.527902568841,219.527477268461,220.527051968081,
221.526626667701,222.526201367321,223.525776066941,224.525350766561,225.524925466181,
226.524500165801,227.524074865421,228.523649565041,229.523224264661,230.522798964281,
231.522373663901,232.521948363521,233.521523063141,234.521097762761,235.520672462381,
236.520247162001,237.519821861621,238.519396561241,239.518971260861,240.518545960481,
241.518120660101,242.517695359721,243.517270059341,244.516844758961,245.516419458581,
246.515994158201,247.515568857821,248.515143557441,249.514718257061,250.514292956681,
251.513867656301,252.513442355921,253.513017055541,254.512591755161,255.512166454781,
256.511741154401,257.511315854021,258.510890553641,259.510465253261,260.510039952881,
261.509614652501,262.509189352121,263.508764051741,264.508338751361,265.507913450981,
266.507488150601,267.507062850221,268.506637549841,269.506212249461,270.505786949081,
271.505361648701,272.504936348321,273.504511047941,274.504085747561,275.503660447181,
276.503235146801,277.502809846421,278.502384546041,279.501959245661,280.501533945281,
281.501108644901,282.500683344521,283.500258044141,284.499832743761,285.499407443381,
286.498982143001,287.498556842621,288.498131542241,289.497706241861,290.497280941481,
291.496855641101,292.496430340721,293.496005040341,294.495579739961,295.495154439581,
296.494729139201,297.494303838821,298.493878538441,299.493453238061,300.493027937681,
301.492602637301,302.492177336921,303.491752036541,304.491326736161,305.490901435781,
306.490476135401,307.490050835021,308.489625534641,309.489200234261,310.488774933881,
311.488349633501,312.487924333121,313.487499032741,314.487073732361,315.486648431981,
316.486223131601,317.485797831221,318.485372530841,319.484947230461,320.484521930081,
321.484096629701,322.483671329321,323.483246028941,324.482820728561,325.482395428181,
326.481970127801,327.481544827421,328.481119527041,329.480694226661,330.480268926281,
331.479843625901,332.479418325521,333.478993025141,334.478567724761,335.478142424381,
336.477717124001,337.477291823621,338.476866523241,339.476441222861,340.476015922481,
341.475590622101,342.475165321721,343.474740021341,344.474314720961,345.473889420581,
346.473464120201,347.473038819821,348.472613519441,349.472188219061,350.471762918681,
351.471337618301,352.470912317921,353.470487017541,354.470061717161,355.469636416781,
356.469211116401,357.468785816021,358.468360515641,359.467935215261,360.467509914881,
361.467084614501,362.466659314121,363.466234013741,364.465808713361,365.465383412981,
366.464958112601,367.464532812221,368.464107511841,369.463682211461,370.463256911081,
371.462831610701,372.462406310321,373.461981009941,374.461555709561,375.461130409181,
376.460705108801,377.460279808421,378.459854508041,379.459429207661,380.459003907281,
381.458578606901,382.458153306521,383.457728006141,384.457302705761,385.456877405381,
386.456452105001,387.456026804621,388.455601504241,389.455176203861,390.454750903481,
391.454325603101,392.453900302721,393.453475002341,394.453049701961,395.452624401581,
396.452199101201,397.451773800821,398.451348500441,399.450923200061,400.450497899681,
401.450072599301,402.449647298921,403.449221998541,404.448796698161,405.448371397781,
406.447946097401,407.447520797021,408.447095496641,409.446670196261,410.446244895881,
411.445819595501,412.445394295121,413.444968994741,414.444543694361,415.444118393981,
416.443693093601,417.443267793221,418.442842492841,419.442417192461,420.441991892081,
421.441566591701,422.441141291321,423.440715990941,424.440290690561,425.439865390181,
426.439440089801,427.439014789421,428.438589489041,429.438164188661,430.437738888281,
431.437313587901,432.436888287521,433.436462987141,434.436037686761,435.435612386381,
436.435187086001,437.434761785621,438.434336485241,439.433911184861,440.433485884481,
441.433060584101,442.432635283721,443.432209983341,444.431784682961,445.431359382581,
446.430934082201),.UNSPECIFIED.);
#666=CYLINDRICAL_SURFACE('',#32455,1.4635);
#667=CYLINDRICAL_SURFACE('',#32457,1.4635);
#668=CYLINDRICAL_SURFACE('',#32458,1.4635);
#669=CYLINDRICAL_SURFACE('',#32459,1.4635);
#670=CYLINDRICAL_SURFACE('',#32460,1.4635);
#671=CYLINDRICAL_SURFACE('',#32461,1.4635);
#672=CYLINDRICAL_SURFACE('',#32462,1.4635);
#673=CYLINDRICAL_SURFACE('',#32463,1.4635);
#674=CYLINDRICAL_SURFACE('',#32464,1.4635);
#675=CYLINDRICAL_SURFACE('',#32465,1.4635);
#676=CYLINDRICAL_SURFACE('',#32466,1.4635);
#677=CYLINDRICAL_SURFACE('',#32467,1.4635);
#678=CYLINDRICAL_SURFACE('',#32468,1.4635);
#679=CYLINDRICAL_SURFACE('',#32469,1.4635);
#680=CYLINDRICAL_SURFACE('',#32470,1.4635);
#681=CYLINDRICAL_SURFACE('',#32471,1.4635);
#682=CYLINDRICAL_SURFACE('',#32472,1.4635);
#683=CYLINDRICAL_SURFACE('',#32473,1.4635);
#684=CYLINDRICAL_SURFACE('',#32474,1.4635);
#685=CYLINDRICAL_SURFACE('',#32475,1.4635);
#686=CYLINDRICAL_SURFACE('',#32476,1.4635);
#687=CYLINDRICAL_SURFACE('',#32477,1.4635);
#688=CYLINDRICAL_SURFACE('',#32478,1.4635);
#689=CYLINDRICAL_SURFACE('',#32479,1.4635);
#690=CYLINDRICAL_SURFACE('',#32480,1.4635);
#691=CYLINDRICAL_SURFACE('',#32481,1.4635);
#692=CYLINDRICAL_SURFACE('',#32482,1.4635);
#693=CYLINDRICAL_SURFACE('',#32483,1.4635);
#694=CYLINDRICAL_SURFACE('',#32484,1.4635);
#695=CYLINDRICAL_SURFACE('',#32485,1.4635);
#696=CYLINDRICAL_SURFACE('',#32486,1.4635);
#697=CYLINDRICAL_SURFACE('',#32487,1.4635);
#698=CYLINDRICAL_SURFACE('',#32488,1.4635);
#699=CYLINDRICAL_SURFACE('',#32489,1.4635);
#700=CYLINDRICAL_SURFACE('',#32490,1.4635);
#701=CYLINDRICAL_SURFACE('',#32491,1.4635);
#702=CYLINDRICAL_SURFACE('',#32492,1.4635);
#703=CYLINDRICAL_SURFACE('',#32493,1.4635);
#704=CYLINDRICAL_SURFACE('',#32494,1.4635);
#705=CYLINDRICAL_SURFACE('',#32495,1.4635);
#706=CYLINDRICAL_SURFACE('',#32496,1.4635);
#707=CYLINDRICAL_SURFACE('',#32497,1.4635);
#708=CYLINDRICAL_SURFACE('',#32498,1.4635);
#709=CYLINDRICAL_SURFACE('',#32499,1.4635);
#710=CYLINDRICAL_SURFACE('',#32500,1.4635);
#711=CYLINDRICAL_SURFACE('',#32501,1.4635);
#712=CYLINDRICAL_SURFACE('',#32502,1.4635);
#713=CYLINDRICAL_SURFACE('',#32503,1.4635);
#714=CYLINDRICAL_SURFACE('',#32504,1.4635);
#715=CYLINDRICAL_SURFACE('',#32505,1.4635);
#716=CYLINDRICAL_SURFACE('',#32506,1.4635);
#717=CYLINDRICAL_SURFACE('',#32507,1.4635);
#718=CYLINDRICAL_SURFACE('',#32508,1.4635);
#719=CYLINDRICAL_SURFACE('',#32509,1.4635);
#720=CYLINDRICAL_SURFACE('',#32510,1.4635);
#721=CYLINDRICAL_SURFACE('',#32511,1.4635);
#722=CYLINDRICAL_SURFACE('',#32512,1.4635);
#723=CYLINDRICAL_SURFACE('',#32513,1.4635);
#724=CYLINDRICAL_SURFACE('',#32514,1.4635);
#725=CYLINDRICAL_SURFACE('',#32515,1.4635);
#726=CYLINDRICAL_SURFACE('',#32516,1.4635);
#727=CYLINDRICAL_SURFACE('',#32517,1.4635);
#728=CYLINDRICAL_SURFACE('',#32518,1.4635);
#729=CYLINDRICAL_SURFACE('',#32519,1.4635);
#730=CYLINDRICAL_SURFACE('',#32520,1.4635);
#731=CYLINDRICAL_SURFACE('',#32521,1.4635);
#732=CYLINDRICAL_SURFACE('',#32522,1.4635);
#733=CYLINDRICAL_SURFACE('',#32523,1.4635);
#734=CYLINDRICAL_SURFACE('',#32524,1.4635);
#735=CYLINDRICAL_SURFACE('',#32525,1.17775);
#736=CYLINDRICAL_SURFACE('',#32527,1.17775);
#737=CYLINDRICAL_SURFACE('',#32528,1.17775);
#738=CYLINDRICAL_SURFACE('',#32529,1.17775);
#739=CYLINDRICAL_SURFACE('',#32530,1.17775);
#740=CYLINDRICAL_SURFACE('',#32531,1.17775);
#741=CYLINDRICAL_SURFACE('',#32532,1.17775);
#742=CYLINDRICAL_SURFACE('',#32533,1.17775);
#743=CYLINDRICAL_SURFACE('',#32534,1.17775);
#744=CYLINDRICAL_SURFACE('',#32535,1.17775);
#745=CYLINDRICAL_SURFACE('',#32536,1.17775);
#746=CYLINDRICAL_SURFACE('',#32537,1.17775);
#747=CYLINDRICAL_SURFACE('',#32538,1.17775);
#748=CYLINDRICAL_SURFACE('',#32539,1.17775);
#749=CYLINDRICAL_SURFACE('',#32540,1.17775);
#750=CYLINDRICAL_SURFACE('',#32541,1.17775);
#751=CYLINDRICAL_SURFACE('',#32542,1.17775);
#752=CYLINDRICAL_SURFACE('',#32543,1.17775);
#753=CYLINDRICAL_SURFACE('',#32544,1.17775);
#754=CYLINDRICAL_SURFACE('',#32545,1.17775);
#755=CYLINDRICAL_SURFACE('',#32546,1.17775);
#756=CYLINDRICAL_SURFACE('',#32547,1.17775);
#757=CYLINDRICAL_SURFACE('',#32548,1.17775);
#758=CYLINDRICAL_SURFACE('',#32549,1.17775);
#759=CYLINDRICAL_SURFACE('',#32550,1.17775);
#760=CYLINDRICAL_SURFACE('',#32551,1.17775);
#761=CYLINDRICAL_SURFACE('',#32552,1.17775);
#762=CYLINDRICAL_SURFACE('',#32553,1.17775);
#763=CYLINDRICAL_SURFACE('',#32554,1.17775);
#764=CYLINDRICAL_SURFACE('',#32555,1.17775);
#765=CYLINDRICAL_SURFACE('',#32556,1.17775);
#766=CYLINDRICAL_SURFACE('',#32557,1.17775);
#767=CYLINDRICAL_SURFACE('',#32558,1.17775);
#768=CYLINDRICAL_SURFACE('',#32559,1.17775);
#769=CYLINDRICAL_SURFACE('',#32560,1.17775);
#770=CYLINDRICAL_SURFACE('',#32561,1.17775);
#771=CYLINDRICAL_SURFACE('',#32562,1.17775);
#772=CYLINDRICAL_SURFACE('',#32563,1.17775);
#773=CYLINDRICAL_SURFACE('',#32564,1.17775);
#774=CYLINDRICAL_SURFACE('',#32565,1.17775);
#775=CYLINDRICAL_SURFACE('',#32566,1.17775);
#776=CYLINDRICAL_SURFACE('',#32567,1.17775);
#777=CYLINDRICAL_SURFACE('',#32568,1.17775);
#778=CYLINDRICAL_SURFACE('',#32569,1.17775);
#779=CYLINDRICAL_SURFACE('',#32570,1.17775);
#780=CYLINDRICAL_SURFACE('',#32571,1.17775);
#781=CYLINDRICAL_SURFACE('',#32572,1.17775);
#782=CYLINDRICAL_SURFACE('',#32573,1.17775);
#783=CYLINDRICAL_SURFACE('',#32574,1.17775);
#784=CYLINDRICAL_SURFACE('',#32575,1.17775);
#785=CYLINDRICAL_SURFACE('',#32576,1.17775);
#786=CYLINDRICAL_SURFACE('',#32577,1.17775);
#787=CYLINDRICAL_SURFACE('',#32578,1.17775);
#788=CYLINDRICAL_SURFACE('',#32579,1.17775);
#789=CYLINDRICAL_SURFACE('',#32580,1.17775);
#790=CYLINDRICAL_SURFACE('',#32581,1.17775);
#791=CYLINDRICAL_SURFACE('',#32582,1.17775);
#792=CYLINDRICAL_SURFACE('',#32583,1.17775);
#793=CYLINDRICAL_SURFACE('',#32584,1.17775);
#794=CYLINDRICAL_SURFACE('',#32585,1.17775);
#795=CYLINDRICAL_SURFACE('',#32586,1.17775);
#796=CYLINDRICAL_SURFACE('',#32587,1.17775);
#797=CYLINDRICAL_SURFACE('',#32588,1.17775);
#798=CYLINDRICAL_SURFACE('',#32589,1.17775);
#799=CYLINDRICAL_SURFACE('',#32590,1.17775);
#800=CYLINDRICAL_SURFACE('',#32591,1.17775);
#801=CYLINDRICAL_SURFACE('',#32592,1.17775);
#802=CYLINDRICAL_SURFACE('',#32593,1.17775);
#803=CYLINDRICAL_SURFACE('',#32594,1.17775);
#804=CYLINDRICAL_SURFACE('',#32602,1.17775);
#805=CYLINDRICAL_SURFACE('',#32607,1.4635);
#806=CYLINDRICAL_SURFACE('',#32840,2.75);
#1635=CIRCLE('',#32456,1.4635);
#1636=CIRCLE('',#32526,1.17775);
#1637=CIRCLE('',#32596,1.4635);
#1638=CIRCLE('',#32597,1.4635);
#1639=CIRCLE('',#32599,1.4635);
#1640=CIRCLE('',#32600,1.4635);
#1641=CIRCLE('',#32601,1.17775);
#1642=CIRCLE('',#32604,0.2);
#1643=CIRCLE('',#32605,1.6635);
#1644=CIRCLE('',#32606,1.4635);
#1645=CIRCLE('',#32609,2.75);
#1646=CIRCLE('',#32612,2.75);
#1647=CIRCLE('',#32615,2.75);
#1648=CIRCLE('',#32618,2.75);
#1649=CIRCLE('',#32621,2.75);
#1650=CIRCLE('',#32624,2.75);
#1651=CIRCLE('',#32627,2.75);
#1652=CIRCLE('',#32630,2.75);
#1653=CIRCLE('',#32633,2.75);
#1654=CIRCLE('',#32636,2.75);
#1655=CIRCLE('',#32639,2.75);
#1656=CIRCLE('',#32642,2.75);
#1657=CIRCLE('',#32645,2.75);
#1658=CIRCLE('',#32648,2.75);
#1659=CIRCLE('',#32651,2.75);
#1660=CIRCLE('',#32654,2.75);
#1661=CIRCLE('',#32657,2.75);
#1662=CIRCLE('',#32660,2.75);
#1663=CIRCLE('',#32663,2.75);
#1664=CIRCLE('',#32666,2.75);
#1665=CIRCLE('',#32669,2.75);
#1666=CIRCLE('',#32672,2.75);
#1667=CIRCLE('',#32675,2.75);
#1668=CIRCLE('',#32678,2.75);
#1669=CIRCLE('',#32681,2.75);
#1670=CIRCLE('',#32684,2.75);
#1671=CIRCLE('',#32687,2.75);
#1672=CIRCLE('',#32690,2.75);
#1673=CIRCLE('',#32693,2.75);
#1674=CIRCLE('',#32696,2.75);
#1675=CIRCLE('',#32699,2.75);
#1676=CIRCLE('',#32702,2.75);
#1677=CIRCLE('',#32705,2.75);
#1678=CIRCLE('',#32708,2.75);
#1679=CIRCLE('',#32711,2.75);
#1680=CIRCLE('',#32714,2.75);
#1681=CIRCLE('',#32715,2.75);
#1682=CIRCLE('',#32718,2.75);
#1683=CIRCLE('',#32719,2.75);
#1684=CIRCLE('',#32722,2.75);
#1685=CIRCLE('',#32725,2.75);
#1686=CIRCLE('',#32728,2.75);
#1687=CIRCLE('',#32731,2.75);
#1688=CIRCLE('',#32734,2.75);
#1689=CIRCLE('',#32737,2.75);
#1690=CIRCLE('',#32740,2.75);
#1691=CIRCLE('',#32743,2.75);
#1692=CIRCLE('',#32746,2.75);
#1693=CIRCLE('',#32749,2.75);
#1694=CIRCLE('',#32752,2.75);
#1695=CIRCLE('',#32755,2.75);
#1696=CIRCLE('',#32758,2.75);
#1697=CIRCLE('',#32761,2.75);
#1698=CIRCLE('',#32764,2.75);
#1699=CIRCLE('',#32767,2.75);
#1700=CIRCLE('',#32770,2.75);
#1701=CIRCLE('',#32773,2.75);
#1702=CIRCLE('',#32776,2.75);
#1703=CIRCLE('',#32779,2.75);
#1704=CIRCLE('',#32782,2.75);
#1705=CIRCLE('',#32785,2.75);
#1706=CIRCLE('',#32788,2.75);
#1707=CIRCLE('',#32791,2.75);
#1708=CIRCLE('',#32794,2.75);
#1709=CIRCLE('',#32797,2.75);
#1710=CIRCLE('',#32800,2.75);
#1711=CIRCLE('',#32803,2.75);
#1712=CIRCLE('',#32806,2.75);
#1713=CIRCLE('',#32809,2.75);
#1714=CIRCLE('',#32812,2.75);
#1715=CIRCLE('',#32815,2.75);
#1716=CIRCLE('',#32818,2.75);
#1717=CIRCLE('',#32821,2.75);
#1718=CIRCLE('',#32824,2.75);
#1719=CIRCLE('',#32827,2.75);
#1720=CIRCLE('',#32829,1.23357587978679);
#1721=CIRCLE('',#32838,1.1);
#1722=CIRCLE('',#32841,2.75);
#1723=CIRCLE('',#32843,2.45);
#2044=CONICAL_SURFACE('',#32828,0.625,1.02388712580674);
#2045=CONICAL_SURFACE('',#32839,1.3,0.785398163397448);
#2046=CONICAL_SURFACE('',#32842,2.6,0.785398163397449);
#2551=B_SPLINE_CURVE_WITH_KNOTS('',3,(#56003,#56004,#56005,#56006,#56007,
#56008,#56009,#56010,#56011,#56012),.UNSPECIFIED.,.F.,.F.,(4,3,3,4),(-4.09202352044849,
-3.99829879847999,-2.99872409886,-2.07317267331967),.UNSPECIFIED.);
#2552=B_SPLINE_CURVE_WITH_KNOTS('',3,(#56015,#56016,#56017,#56018,#56019,
#56020,#56021),.UNSPECIFIED.,.F.,.F.,(4,3,4),(0.,0.99957469961999,1.12274180646236),
 .UNSPECIFIED.);
#2553=B_SPLINE_CURVE_WITH_KNOTS('',3,(#56026,#56027,#56028,#56029,#56030,
#56031,#56032,#56033,#56034,#56035,#56036,#56037,#56038,#56039,#56040,#56041,
#56042,#56043,#56044,#56045,#56046,#56047),.UNSPECIFIED.,.F.,.F.,(4,3,3,
3,3,3,3,4),(-10.3752088276281,-9.99574699619999,-8.99617229657999,-7.99659759695999,
-6.99702289733998,-5.99744819771999,-4.99787349809999,-4.09202352044849),
 .UNSPECIFIED.);
#2554=B_SPLINE_CURVE_WITH_KNOTS('',3,(#56048,#56049,#56050,#56051,#56052,
#56053,#56054,#56055,#56056,#56057,#56058,#56059,#56060,#56061,#56062,#56063,
#56064,#56065,#56066,#56067,#56068,#56069),.UNSPECIFIED.,.F.,.F.,(4,3,3,
3,3,3,3,4),(1.12274180646236,1.99914939923999,2.99872409886,3.99829879848,
4.9978734981,5.99744819772,6.99702289734001,7.40592711364193),
 .UNSPECIFIED.);
#2555=B_SPLINE_CURVE_WITH_KNOTS('',3,(#56074,#56075,#56076,#56077,#56078,
#56079,#56080,#56081,#56082,#56083,#56084,#56085,#56086,#56087,#56088,#56089,
#56090,#56091,#56092,#56093,#56094,#56095),.UNSPECIFIED.,.F.,.F.,(4,3,3,
3,3,3,3,4),(-16.6583941348077,-15.99319519392,-14.9936204943,-13.99404579468,
-12.99447109506,-11.99489639544,-10.99532169582,-10.3752088276281),
 .UNSPECIFIED.);
#2556=B_SPLINE_CURVE_WITH_KNOTS('',3,(#56096,#56097,#56098,#56099,#56100,
#56101,#56102,#56103,#56104,#56105,#56106,#56107,#56108,#56109,#56110,#56111,
#56112,#56113,#56114,#56115,#56116,#56117),.UNSPECIFIED.,.F.,.F.,(4,3,3,
3,3,3,3,4),(7.40592711364193,7.99659759696,8.99617229658,9.99574699619999,
10.99532169582,11.99489639544,12.99447109506,13.6891124208215),
 .UNSPECIFIED.);
#2557=B_SPLINE_CURVE_WITH_KNOTS('',3,(#56122,#56123,#56124,#56125,#56126,
#56127,#56128,#56129,#56130,#56131,#56132,#56133,#56134,#56135,#56136,#56137,
#56138,#56139,#56140,#56141,#56142,#56143),.UNSPECIFIED.,.F.,.F.,(4,3,3,
3,3,3,3,4),(-22.9415794419873,-21.99064339164,-20.99106869202,-19.9914939924,
-18.99191929278,-17.99234459316,-16.99276989354,-16.6583941348077),
 .UNSPECIFIED.);
#2558=B_SPLINE_CURVE_WITH_KNOTS('',3,(#56144,#56145,#56146,#56147,#56148,
#56149,#56150,#56151,#56152,#56153,#56154,#56155,#56156,#56157,#56158,#56159,
#56160,#56161,#56162,#56163,#56164,#56165),.UNSPECIFIED.,.F.,.F.,(4,3,3,
3,3,3,3,4),(13.6891124208215,13.99404579468,14.9936204943,15.99319519392,
16.99276989354,17.99234459316,18.99191929278,19.9722977280011),
 .UNSPECIFIED.);
#2559=B_SPLINE_CURVE_WITH_KNOTS('',3,(#56170,#56171,#56172,#56173,#56174,
#56175,#56176,#56177,#56178,#56179,#56180,#56181,#56182,#56183,#56184,#56185,
#56186,#56187,#56188,#56189,#56190,#56191,#56192,#56193,#56194),
 .UNSPECIFIED.,.F.,.F.,(4,3,3,3,3,3,3,3,4),(-29.2247647491669,-28.98766628898,
-27.98809158936,-26.98851688974,-25.98894219012,-24.9893674905,-23.98979279088,
-22.99021809126,-22.9415794419873),.UNSPECIFIED.);
#2560=B_SPLINE_CURVE_WITH_KNOTS('',3,(#56195,#56196,#56197,#56198,#56199,
#56200,#56201,#56202,#56203,#56204,#56205,#56206,#56207,#56208,#56209,#56210,
#56211,#56212,#56213,#56214,#56215,#56216,#56217,#56218,#56219),
 .UNSPECIFIED.,.F.,.F.,(4,3,3,3,3,3,3,3,4),(19.9722977280011,19.9914939924,
20.99106869202,21.99064339164,22.99021809126,23.98979279088,24.9893674905,
25.98894219012,26.2554830351807),.UNSPECIFIED.);
#2561=B_SPLINE_CURVE_WITH_KNOTS('',3,(#56224,#56225,#56226,#56227,#56228,
#56229,#56230,#56231,#56232,#56233,#56234,#56235,#56236,#56237,#56238,#56239,
#56240,#56241,#56242,#56243,#56244,#56245),.UNSPECIFIED.,.F.,.F.,(4,3,3,
3,3,3,3,4),(-35.5079500563464,-34.9851144867,-33.98553978708,-32.98596508746,
-31.9863903878399,-30.98681568822,-29.9872409886,-29.2247647491669),
 .UNSPECIFIED.);
#2562=B_SPLINE_CURVE_WITH_KNOTS('',3,(#56246,#56247,#56248,#56249,#56250,
#56251,#56252,#56253,#56254,#56255,#56256,#56257,#56258,#56259,#56260,#56261,
#56262,#56263,#56264,#56265,#56266,#56267),.UNSPECIFIED.,.F.,.F.,(4,3,3,
3,3,3,3,4),(26.2554830351807,26.98851688974,27.98809158936,28.98766628898,
29.9872409886,30.98681568822,31.98639038784,32.5386683423603),
 .UNSPECIFIED.);
#2563=B_SPLINE_CURVE_WITH_KNOTS('',3,(#56272,#56273,#56274,#56275,#56276,
#56277,#56278,#56279,#56280,#56281,#56282,#56283,#56284,#56285,#56286,#56287,
#56288,#56289,#56290,#56291,#56292,#56293),.UNSPECIFIED.,.F.,.F.,(4,3,3,
3,3,3,3,4),(-41.791135363526,-40.9825626844199,-39.9829879847999,-38.9834132851799,
-37.98383858556,-36.98426388594,-35.9846891863199,-35.5079500563464),
 .UNSPECIFIED.);
#2564=B_SPLINE_CURVE_WITH_KNOTS('',3,(#56294,#56295,#56296,#56297,#56298,
#56299,#56300,#56301,#56302,#56303,#56304,#56305,#56306,#56307,#56308,#56309,
#56310,#56311,#56312,#56313,#56314,#56315),.UNSPECIFIED.,.F.,.F.,(4,3,3,
3,3,3,3,4),(32.5386683423603,32.98596508746,33.98553978708,34.9851144867,
35.98468918632,36.98426388594,37.98383858556,38.8218536495399),
 .UNSPECIFIED.);
#2565=B_SPLINE_CURVE_WITH_KNOTS('',3,(#56320,#56321,#56322,#56323,#56324,
#56325,#56326,#56327,#56328,#56329,#56330,#56331,#56332,#56333,#56334,#56335,
#56336,#56337,#56338,#56339,#56340,#56341,#56342,#56343,#56344),
 .UNSPECIFIED.,.F.,.F.,(4,3,3,3,3,3,3,3,4),(-48.0743206707057,-47.9795855817599,
-46.9800108821399,-45.9804361825199,-44.9808614828999,-43.9812867832799,
-42.9817120836599,-41.9821373840399,-41.791135363526),.UNSPECIFIED.);
#2566=B_SPLINE_CURVE_WITH_KNOTS('',3,(#56345,#56346,#56347,#56348,#56349,
#56350,#56351,#56352,#56353,#56354,#56355,#56356,#56357,#56358,#56359,#56360,
#56361,#56362,#56363,#56364,#56365,#56366,#56367,#56368,#56369),
 .UNSPECIFIED.,.F.,.F.,(4,3,3,3,3,3,3,3,4),(38.8218536495399,38.98341328518,
39.9829879848,40.98256268442,41.98213738404,42.9817120836599,43.9812867832799,
44.9808614828999,45.1050389567195),.UNSPECIFIED.);
#2567=B_SPLINE_CURVE_WITH_KNOTS('',3,(#56374,#56375,#56376,#56377,#56378,
#56379,#56380,#56381,#56382,#56383,#56384,#56385,#56386,#56387,#56388,#56389,
#56390,#56391,#56392,#56393,#56394,#56395),.UNSPECIFIED.,.F.,.F.,(4,3,3,
3,3,3,3,4),(-54.3575059778852,-53.9770337794799,-52.9774590798599,-51.9778843802399,
-50.9783096806199,-49.9787349809999,-48.9791602813799,-48.0743206707057),
 .UNSPECIFIED.);
#2568=B_SPLINE_CURVE_WITH_KNOTS('',3,(#56396,#56397,#56398,#56399,#56400,
#56401,#56402,#56403,#56404,#56405,#56406,#56407,#56408,#56409,#56410,#56411,
#56412,#56413,#56414,#56415,#56416,#56417),.UNSPECIFIED.,.F.,.F.,(4,3,3,
3,3,3,3,4),(45.1050389567195,45.9804361825199,46.9800108821399,47.9795855817599,
48.9791602813799,49.9787349809999,50.9783096806199,51.388224263899),
 .UNSPECIFIED.);
#2569=B_SPLINE_CURVE_WITH_KNOTS('',3,(#56422,#56423,#56424,#56425,#56426,
#56427,#56428,#56429,#56430,#56431,#56432,#56433,#56434,#56435,#56436,#56437,
#56438,#56439,#56440,#56441,#56442,#56443),.UNSPECIFIED.,.F.,.F.,(4,3,3,
3,3,3,3,4),(-60.6406912850648,-59.9744819771999,-58.9749072775799,-57.9753325779599,
-56.9757578783399,-55.9761831787199,-54.9766084790999,-54.3575059778852),
 .UNSPECIFIED.);
#2570=B_SPLINE_CURVE_WITH_KNOTS('',3,(#56444,#56445,#56446,#56447,#56448,
#56449,#56450,#56451,#56452,#56453,#56454,#56455,#56456,#56457,#56458,#56459,
#56460,#56461,#56462,#56463,#56464,#56465),.UNSPECIFIED.,.F.,.F.,(4,3,3,
3,3,3,3,4),(51.388224263899,51.9778843802399,52.9774590798599,53.9770337794799,
54.9766084791,55.9761831787199,56.97575787834,57.6714095710787),
 .UNSPECIFIED.);
#2571=B_SPLINE_CURVE_WITH_KNOTS('',3,(#56470,#56471,#56472,#56473,#56474,
#56475,#56476,#56477,#56478,#56479,#56480,#56481,#56482,#56483,#56484,#56485,
#56486,#56487,#56488,#56489,#56490,#56491),.UNSPECIFIED.,.F.,.F.,(4,3,3,
3,3,3,3,4),(-66.9238765922444,-65.9719301749199,-64.9723554752999,-63.9727807756799,
-62.9732060760599,-61.9736313764399,-60.9740566768199,-60.6406912850648),
 .UNSPECIFIED.);
#2572=B_SPLINE_CURVE_WITH_KNOTS('',3,(#56492,#56493,#56494,#56495,#56496,
#56497,#56498,#56499,#56500,#56501,#56502,#56503,#56504,#56505,#56506,#56507,
#56508,#56509,#56510,#56511,#56512,#56513),.UNSPECIFIED.,.F.,.F.,(4,3,3,
3,3,3,3,4),(57.6714095710787,57.97533257796,58.97490727758,59.9744819772,
60.9740566768199,61.9736313764399,62.9732060760599,63.9545948782583),
 .UNSPECIFIED.);
#2573=B_SPLINE_CURVE_WITH_KNOTS('',3,(#56518,#56519,#56520,#56521,#56522,
#56523,#56524,#56525,#56526,#56527,#56528,#56529,#56530,#56531,#56532,#56533,
#56534,#56535,#56536,#56537,#56538,#56539,#56540,#56541,#56542),
 .UNSPECIFIED.,.F.,.F.,(4,3,3,3,3,3,3,3,4),(-73.207061899424,-72.9689530722599,
-71.9693783726399,-70.9698036730199,-69.9702289733999,-68.9706542737799,
-67.9710795741599,-66.9715048745399,-66.9238765922444),.UNSPECIFIED.);
#2574=B_SPLINE_CURVE_WITH_KNOTS('',3,(#56543,#56544,#56545,#56546,#56547,
#56548,#56549,#56550,#56551,#56552,#56553,#56554,#56555,#56556,#56557,#56558,
#56559,#56560,#56561,#56562,#56563,#56564,#56565,#56566,#56567),
 .UNSPECIFIED.,.F.,.F.,(4,3,3,3,3,3,3,3,4),(63.9545948782583,63.9727807756799,
64.9723554752999,65.9719301749199,66.9715048745399,67.9710795741599,68.9706542737799,
69.9702289733999,70.2377801854378),.UNSPECIFIED.);
#2575=B_SPLINE_CURVE_WITH_KNOTS('',3,(#56572,#56573,#56574,#56575,#56576,
#56577,#56578,#56579,#56580,#56581,#56582,#56583,#56584,#56585,#56586,#56587,
#56588,#56589,#56590,#56591,#56592,#56593),.UNSPECIFIED.,.F.,.F.,(4,3,3,
3,3,3,3,4),(-79.4902472066036,-78.9664012699799,-77.9668265703599,-76.9672518707399,
-75.9676771711199,-74.9681024714999,-73.9685277718799,-73.207061899424),
 .UNSPECIFIED.);
#2576=B_SPLINE_CURVE_WITH_KNOTS('',3,(#56594,#56595,#56596,#56597,#56598,
#56599,#56600,#56601,#56602,#56603,#56604,#56605,#56606,#56607,#56608,#56609,
#56610,#56611,#56612,#56613,#56614,#56615),.UNSPECIFIED.,.F.,.F.,(4,3,3,
3,3,3,3,4),(70.2377801854378,70.9698036730199,71.9693783726399,72.9689530722599,
73.9685277718799,74.9681024714999,75.9676771711199,76.5209654926174),
 .UNSPECIFIED.);
#2577=B_SPLINE_CURVE_WITH_KNOTS('',3,(#56620,#56621,#56622,#56623,#56624,
#56625,#56626,#56627,#56628,#56629,#56630,#56631,#56632,#56633,#56634,#56635,
#56636,#56637,#56638,#56639,#56640,#56641),.UNSPECIFIED.,.F.,.F.,(4,3,3,
3,3,3,3,4),(-85.7734325137832,-84.9638494676999,-83.9642747680799,-82.9647000684599,
-81.9651253688399,-80.9655506692199,-79.9659759695999,-79.4902472066036),
 .UNSPECIFIED.);
#2578=B_SPLINE_CURVE_WITH_KNOTS('',3,(#56642,#56643,#56644,#56645,#56646,
#56647,#56648,#56649,#56650,#56651,#56652,#56653,#56654,#56655,#56656,#56657,
#56658,#56659,#56660,#56661,#56662,#56663),.UNSPECIFIED.,.F.,.F.,(4,3,3,
3,3,3,3,4),(76.5209654926174,76.9672518707399,77.9668265703599,78.9664012699799,
79.9659759695999,80.9655506692199,81.9651253688399,82.804150799797),
 .UNSPECIFIED.);
#2579=B_SPLINE_CURVE_WITH_KNOTS('',3,(#56668,#56669,#56670,#56671,#56672,
#56673,#56674,#56675,#56676,#56677,#56678,#56679,#56680,#56681,#56682,#56683,
#56684,#56685,#56686,#56687,#56688,#56689,#56690,#56691,#56692),
 .UNSPECIFIED.,.F.,.F.,(4,3,3,3,3,3,3,3,4),(-92.0566178209628,-91.9608723650399,
-90.9612976654198,-89.9617229657999,-88.9621482661799,-87.9625735665599,
-86.9629988669399,-85.9634241673199,-85.7734325137832),.UNSPECIFIED.);
#2580=B_SPLINE_CURVE_WITH_KNOTS('',3,(#56693,#56694,#56695,#56696,#56697,
#56698,#56699,#56700,#56701,#56702,#56703,#56704,#56705,#56706,#56707,#56708,
#56709,#56710,#56711,#56712,#56713,#56714,#56715,#56716,#56717),
 .UNSPECIFIED.,.F.,.F.,(4,3,3,3,3,3,3,3,4),(82.804150799797,82.9647000684599,
83.9642747680799,84.9638494676999,85.9634241673199,86.9629988669399,87.9625735665599,
88.9621482661799,89.0873361069767),.UNSPECIFIED.);
#2581=B_SPLINE_CURVE_WITH_KNOTS('',3,(#56722,#56723,#56724,#56725,#56726,
#56727,#56728,#56729,#56730,#56731,#56732,#56733,#56734,#56735,#56736,#56737,
#56738,#56739,#56740,#56741,#56742,#56743),.UNSPECIFIED.,.F.,.F.,(4,3,3,
3,3,3,3,4),(-98.3398031281424,-97.9583205627599,-96.9587458631399,-95.9591711635199,
-94.9595964638998,-93.9600217642799,-92.9604470646599,-92.0566178209628),
 .UNSPECIFIED.);
#2582=B_SPLINE_CURVE_WITH_KNOTS('',3,(#56744,#56745,#56746,#56747,#56748,
#56749,#56750,#56751,#56752,#56753,#56754,#56755,#56756,#56757,#56758,#56759,
#56760,#56761,#56762,#56763,#56764,#56765),.UNSPECIFIED.,.F.,.F.,(4,3,3,
3,3,3,3,4),(89.0873361069767,89.9617229657999,90.9612976654199,91.9608723650399,
92.9604470646599,93.9600217642799,94.9595964638998,95.3705214141562),
 .UNSPECIFIED.);
#2583=B_SPLINE_CURVE_WITH_KNOTS('',3,(#56770,#56771,#56772,#56773,#56774,
#56775,#56776,#56777,#56778,#56779,#56780,#56781,#56782,#56783,#56784,#56785,
#56786,#56787,#56788,#56789,#56790,#56791),.UNSPECIFIED.,.F.,.F.,(4,3,3,
3,3,3,3,4),(-104.622988435322,-103.95576876048,-102.95619406086,-101.95661936124,
-100.95704466162,-99.9574699619998,-98.9578952623799,-98.3398031281424),
 .UNSPECIFIED.);
#2584=B_SPLINE_CURVE_WITH_KNOTS('',3,(#56792,#56793,#56794,#56795,#56796,
#56797,#56798,#56799,#56800,#56801,#56802,#56803,#56804,#56805,#56806,#56807,
#56808,#56809,#56810,#56811,#56812,#56813),.UNSPECIFIED.,.F.,.F.,(4,3,3,
3,3,3,3,4),(95.3705214141562,95.9591711635198,96.9587458631399,97.9583205627599,
98.9578952623799,99.9574699619999,100.95704466162,101.653706721336),
 .UNSPECIFIED.);
#2585=B_SPLINE_CURVE_WITH_KNOTS('',3,(#56818,#56819,#56820,#56821,#56822,
#56823,#56824,#56825,#56826,#56827,#56828,#56829,#56830,#56831,#56832,#56833,
#56834,#56835,#56836,#56837,#56838,#56839),.UNSPECIFIED.,.F.,.F.,(4,3,3,
3,3,3,3,4),(-110.906173742502,-109.9532169582,-108.95364225858,-107.95406755896,
-106.95449285934,-105.95491815972,-104.9553434601,-104.622988435322),
 .UNSPECIFIED.);
#2586=B_SPLINE_CURVE_WITH_KNOTS('',3,(#56840,#56841,#56842,#56843,#56844,
#56845,#56846,#56847,#56848,#56849,#56850,#56851,#56852,#56853,#56854,#56855,
#56856,#56857,#56858,#56859,#56860,#56861),.UNSPECIFIED.,.F.,.F.,(4,3,3,
3,3,3,3,4),(101.653706721336,101.95661936124,102.95619406086,103.95576876048,
104.9553434601,105.95491815972,106.95449285934,107.936892028515),
 .UNSPECIFIED.);
#2587=B_SPLINE_CURVE_WITH_KNOTS('',3,(#56866,#56867,#56868,#56869,#56870,
#56871,#56872,#56873,#56874,#56875,#56876,#56877,#56878,#56879,#56880,#56881,
#56882,#56883,#56884,#56885,#56886,#56887,#56888,#56889,#56890),
 .UNSPECIFIED.,.F.,.F.,(4,3,3,3,3,3,3,3,4),(-117.189359049681,-116.95023985554,
-115.95066515592,-114.9510904563,-113.95151575668,-112.95194105706,-111.95236635744,
-110.95279165782,-110.906173742502),.UNSPECIFIED.);
#2588=B_SPLINE_CURVE_WITH_KNOTS('',3,(#56891,#56892,#56893,#56894,#56895,
#56896,#56897,#56898,#56899,#56900,#56901,#56902,#56903,#56904,#56905,#56906,
#56907,#56908,#56909,#56910,#56911,#56912,#56913,#56914,#56915),
 .UNSPECIFIED.,.F.,.F.,(4,3,3,3,3,3,3,3,4),(107.936892028515,107.95406755896,
108.95364225858,109.9532169582,110.95279165782,111.95236635744,112.95194105706,
113.95151575668,114.220077335695),.UNSPECIFIED.);
#2589=B_SPLINE_CURVE_WITH_KNOTS('',3,(#56920,#56921,#56922,#56923,#56924,
#56925,#56926,#56927,#56928,#56929,#56930,#56931,#56932,#56933,#56934,#56935,
#56936,#56937,#56938,#56939,#56940,#56941),.UNSPECIFIED.,.F.,.F.,(4,3,3,
3,3,3,3,4),(-123.472544356861,-122.94768805326,-121.94811335364,-120.94853865402,
-119.9489639544,-118.94938925478,-117.94981455516,-117.189359049681),
 .UNSPECIFIED.);
#2590=B_SPLINE_CURVE_WITH_KNOTS('',3,(#56942,#56943,#56944,#56945,#56946,
#56947,#56948,#56949,#56950,#56951,#56952,#56953,#56954,#56955,#56956,#56957,
#56958,#56959,#56960,#56961,#56962,#56963),.UNSPECIFIED.,.F.,.F.,(4,3,3,
3,3,3,3,4),(114.220077335695,114.9510904563,115.95066515592,116.95023985554,
117.94981455516,118.94938925478,119.9489639544,120.503262642875),
 .UNSPECIFIED.);
#2591=B_SPLINE_CURVE_WITH_KNOTS('',3,(#56968,#56969,#56970,#56971,#56972,
#56973,#56974,#56975,#56976,#56977,#56978,#56979,#56980,#56981,#56982,#56983,
#56984,#56985,#56986,#56987,#56988,#56989),.UNSPECIFIED.,.F.,.F.,(4,3,3,
3,3,3,3,4),(-129.75572966404,-128.94513625098,-127.94556155136,-126.94598685174,
-125.94641215212,-124.9468374525,-123.94726275288,-123.472544356861),
 .UNSPECIFIED.);
#2592=B_SPLINE_CURVE_WITH_KNOTS('',3,(#56990,#56991,#56992,#56993,#56994,
#56995,#56996,#56997,#56998,#56999,#57000,#57001,#57002,#57003,#57004,#57005,
#57006,#57007,#57008,#57009,#57010,#57011),.UNSPECIFIED.,.F.,.F.,(4,3,3,
3,3,3,3,4),(120.503262642875,120.94853865402,121.94811335364,122.94768805326,
123.94726275288,124.9468374525,125.94641215212,126.786447950054),
 .UNSPECIFIED.);
#2593=B_SPLINE_CURVE_WITH_KNOTS('',3,(#57016,#57017,#57018,#57019,#57020,
#57021,#57022,#57023,#57024,#57025,#57026,#57027,#57028,#57029,#57030,#57031,
#57032,#57033,#57034,#57035,#57036,#57037,#57038,#57039,#57040),
 .UNSPECIFIED.,.F.,.F.,(4,3,3,3,3,3,3,3,4),(-136.03891497122,-135.94215914832,
-134.9425844487,-133.94300974908,-132.94343504946,-131.94386034984,-130.94428565022,
-129.9447109506,-129.75572966404),.UNSPECIFIED.);
#2594=B_SPLINE_CURVE_WITH_KNOTS('',3,(#57041,#57042,#57043,#57044,#57045,
#57046,#57047,#57048,#57049,#57050,#57051,#57052,#57053,#57054,#57055,#57056,
#57057,#57058,#57059,#57060,#57061,#57062,#57063,#57064,#57065),
 .UNSPECIFIED.,.F.,.F.,(4,3,3,3,3,3,3,3,4),(126.786447950054,126.94598685174,
127.94556155136,128.94513625098,129.9447109506,130.94428565022,131.94386034984,
132.94343504946,133.069633257234),.UNSPECIFIED.);
#2595=B_SPLINE_CURVE_WITH_KNOTS('',3,(#57070,#57071,#57072,#57073,#57074,
#57075,#57076,#57077,#57078,#57079,#57080,#57081,#57082,#57083,#57084,#57085,
#57086,#57087,#57088,#57089,#57090,#57091),.UNSPECIFIED.,.F.,.F.,(4,3,3,
3,3,3,3,4),(-142.322100278399,-141.93960734604,-140.94003264642,-139.9404579468,
-138.94088324718,-137.94130854756,-136.94173384794,-136.03891497122),
 .UNSPECIFIED.);
#2596=B_SPLINE_CURVE_WITH_KNOTS('',3,(#57092,#57093,#57094,#57095,#57096,
#57097,#57098,#57099,#57100,#57101,#57102,#57103,#57104,#57105,#57106,#57107,
#57108,#57109,#57110,#57111,#57112,#57113),.UNSPECIFIED.,.F.,.F.,(4,3,3,
3,3,3,3,4),(133.069633257234,133.94300974908,134.9425844487,135.94215914832,
136.94173384794,137.94130854756,138.94088324718,139.352818564413),
 .UNSPECIFIED.);
#2597=B_SPLINE_CURVE_WITH_KNOTS('',3,(#57118,#57119,#57120,#57121,#57122,
#57123,#57124,#57125,#57126,#57127,#57128,#57129,#57130,#57131,#57132,#57133,
#57134,#57135,#57136,#57137,#57138,#57139),.UNSPECIFIED.,.F.,.F.,(4,3,3,
3,3,3,3,4),(-148.605285585579,-147.93705554376,-146.93748084414,-145.93790614452,
-144.9383314449,-143.93875674528,-142.93918204566,-142.322100278399),
 .UNSPECIFIED.);
#2598=B_SPLINE_CURVE_WITH_KNOTS('',3,(#57140,#57141,#57142,#57143,#57144,
#57145,#57146,#57147,#57148,#57149,#57150,#57151,#57152,#57153,#57154,#57155,
#57156,#57157,#57158,#57159,#57160,#57161),.UNSPECIFIED.,.F.,.F.,(4,3,3,
3,3,3,3,4),(139.352818564413,139.9404579468,140.94003264642,141.93960734604,
142.93918204566,143.93875674528,144.9383314449,145.636003871593),
 .UNSPECIFIED.);
#2599=B_SPLINE_CURVE_WITH_KNOTS('',3,(#57166,#57167,#57168,#57169,#57170,
#57171,#57172,#57173,#57174,#57175,#57176,#57177,#57178,#57179,#57180,#57181,
#57182,#57183,#57184,#57185,#57186,#57187),.UNSPECIFIED.,.F.,.F.,(4,3,3,
3,3,3,3,4),(-154.888470892759,-153.93450374148,-152.93492904186,-151.93535434224,
-150.93577964262,-149.936204943,-148.93663024338,-148.605285585579),
 .UNSPECIFIED.);
#2600=B_SPLINE_CURVE_WITH_KNOTS('',3,(#57188,#57189,#57190,#57191,#57192,
#57193,#57194,#57195,#57196,#57197,#57198,#57199,#57200,#57201,#57202,#57203,
#57204,#57205,#57206,#57207,#57208,#57209),.UNSPECIFIED.,.F.,.F.,(4,3,3,
3,3,3,3,4),(145.636003871593,145.93790614452,146.93748084414,147.93705554376,
148.93663024338,149.936204943,150.93577964262,151.919189178772),
 .UNSPECIFIED.);
#2601=B_SPLINE_CURVE_WITH_KNOTS('',3,(#57214,#57215,#57216,#57217,#57218,
#57219,#57220,#57221,#57222,#57223,#57224,#57225,#57226,#57227,#57228,#57229,
#57230,#57231,#57232,#57233,#57234,#57235,#57236,#57237,#57238),
 .UNSPECIFIED.,.F.,.F.,(4,3,3,3,3,3,3,3,4),(-161.171656199938,-160.93152663882,
-159.9319519392,-158.93237723958,-157.93280253996,-156.93322784034,-155.93365314072,
-154.9340784411,-154.888470892759),.UNSPECIFIED.);
#2602=B_SPLINE_CURVE_WITH_KNOTS('',3,(#57239,#57240,#57241,#57242,#57243,
#57244,#57245,#57246,#57247,#57248,#57249,#57250,#57251,#57252,#57253,#57254,
#57255,#57256,#57257,#57258,#57259,#57260,#57261,#57262,#57263),
 .UNSPECIFIED.,.F.,.F.,(4,3,3,3,3,3,3,3,4),(151.919189178772,151.93535434224,
152.93492904186,153.93450374148,154.9340784411,155.93365314072,156.93322784034,
157.93280253996,158.202374485952),.UNSPECIFIED.);
#2603=B_SPLINE_CURVE_WITH_KNOTS('',3,(#57268,#57269,#57270,#57271,#57272,
#57273,#57274,#57275,#57276,#57277,#57278,#57279,#57280,#57281,#57282,#57283,
#57284,#57285,#57286,#57287,#57288,#57289),.UNSPECIFIED.,.F.,.F.,(4,3,3,
3,3,3,3,4),(-167.454841507118,-166.92897483654,-165.92940013692,-164.9298254373,
-163.93025073768,-162.93067603806,-161.93110133844,-161.171656199938),
 .UNSPECIFIED.);
#2604=B_SPLINE_CURVE_WITH_KNOTS('',3,(#57290,#57291,#57292,#57293,#57294,
#57295,#57296,#57297,#57298,#57299,#57300,#57301,#57302,#57303,#57304,#57305,
#57306,#57307,#57308,#57309,#57310,#57311),.UNSPECIFIED.,.F.,.F.,(4,3,3,
3,3,3,3,4),(158.202374485952,158.93237723958,159.9319519392,160.93152663882,
161.93110133844,162.93067603806,163.93025073768,164.485559793132),
 .UNSPECIFIED.);
#2605=B_SPLINE_CURVE_WITH_KNOTS('',3,(#57316,#57317,#57318,#57319,#57320,
#57321,#57322,#57323,#57324,#57325,#57326,#57327,#57328,#57329,#57330,#57331,
#57332,#57333,#57334,#57335,#57336,#57337),.UNSPECIFIED.,.F.,.F.,(4,3,3,
3,3,3,3,4),(-173.738026814297,-172.92642303426,-171.92684833464,-170.92727363502,
-169.9276989354,-168.92812423578,-167.92854953616,-167.454841507118),
 .UNSPECIFIED.);
#2606=B_SPLINE_CURVE_WITH_KNOTS('',3,(#57338,#57339,#57340,#57341,#57342,
#57343,#57344,#57345,#57346,#57347,#57348,#57349,#57350,#57351,#57352,#57353,
#57354,#57355,#57356,#57357,#57358,#57359),.UNSPECIFIED.,.F.,.F.,(4,3,3,
3,3,3,3,4),(164.485559793132,164.9298254373,165.92940013692,166.92897483654,
167.92854953616,168.92812423578,169.9276989354,170.768745100311),
 .UNSPECIFIED.);
#2607=B_SPLINE_CURVE_WITH_KNOTS('',3,(#57364,#57365,#57366,#57367,#57368,
#57369,#57370,#57371,#57372,#57373,#57374,#57375,#57376,#57377,#57378,#57379,
#57380,#57381,#57382,#57383,#57384,#57385,#57386,#57387,#57388),
 .UNSPECIFIED.,.F.,.F.,(4,3,3,3,3,3,3,3,4),(-180.021212121477,-179.9234459316,
-178.92387123198,-177.92429653236,-176.92472183274,-175.92514713312,-174.9255724335,
-173.92599773388,-173.738026814297),.UNSPECIFIED.);
#2608=B_SPLINE_CURVE_WITH_KNOTS('',3,(#57389,#57390,#57391,#57392,#57393,
#57394,#57395,#57396,#57397,#57398,#57399,#57400,#57401,#57402,#57403,#57404,
#57405,#57406,#57407,#57408,#57409,#57410,#57411,#57412,#57413),
 .UNSPECIFIED.,.F.,.F.,(4,3,3,3,3,3,3,3,4),(170.768745100311,170.92727363502,
171.92684833464,172.92642303426,173.92599773388,174.9255724335,175.92514713312,
176.92472183274,177.051930407491),.UNSPECIFIED.);
#2609=B_SPLINE_CURVE_WITH_KNOTS('',3,(#57418,#57419,#57420,#57421,#57422,
#57423,#57424,#57425,#57426,#57427,#57428,#57429,#57430,#57431,#57432,#57433,
#57434,#57435,#57436,#57437,#57438,#57439),.UNSPECIFIED.,.F.,.F.,(4,3,3,
3,3,3,3,4),(-186.304397428656,-185.92089412932,-184.9213194297,-183.92174473008,
-182.92217003046,-181.92259533084,-180.92302063122,-180.021212121477),
 .UNSPECIFIED.);
#2610=B_SPLINE_CURVE_WITH_KNOTS('',3,(#57440,#57441,#57442,#57443,#57444,
#57445,#57446,#57447,#57448,#57449,#57450,#57451,#57452,#57453,#57454,#57455,
#57456,#57457,#57458,#57459,#57460,#57461),.UNSPECIFIED.,.F.,.F.,(4,3,3,
3,3,3,3,4),(177.051930407491,177.92429653236,178.92387123198,179.9234459316,
180.92302063122,181.92259533084,182.92217003046,183.33511571467),
 .UNSPECIFIED.);
#2611=B_SPLINE_CURVE_WITH_KNOTS('',3,(#57466,#57467,#57468,#57469,#57470,
#57471,#57472,#57473,#57474,#57475,#57476,#57477,#57478,#57479,#57480,#57481,
#57482,#57483,#57484,#57485,#57486,#57487),.UNSPECIFIED.,.F.,.F.,(4,3,3,
3,3,3,3,4),(-192.587582735836,-191.91834232704,-190.91876762742,-189.9191929278,
-188.91961822818,-187.92004352856,-186.92046882894,-186.304397428656),
 .UNSPECIFIED.);
#2612=B_SPLINE_CURVE_WITH_KNOTS('',3,(#57488,#57489,#57490,#57491,#57492,
#57493,#57494,#57495,#57496,#57497,#57498,#57499,#57500,#57501,#57502,#57503,
#57504,#57505,#57506,#57507,#57508,#57509),.UNSPECIFIED.,.F.,.F.,(4,3,3,
3,3,3,3,4),(183.33511571467,183.92174473008,184.9213194297,185.92089412932,
186.92046882894,187.92004352856,188.91961822818,189.61830102185),
 .UNSPECIFIED.);
#2613=B_SPLINE_CURVE_WITH_KNOTS('',3,(#57514,#57515,#57516,#57517,#57518,
#57519,#57520,#57521,#57522,#57523,#57524,#57525,#57526,#57527,#57528,#57529,
#57530,#57531,#57532,#57533,#57534,#57535),.UNSPECIFIED.,.F.,.F.,(4,3,3,
3,3,3,3,4),(-198.870768043016,-197.91579052476,-196.91621582514,-195.91664112552,
-194.9170664259,-193.91749172628,-192.91791702666,-192.587582735836),
 .UNSPECIFIED.);
#2614=B_SPLINE_CURVE_WITH_KNOTS('',3,(#57536,#57537,#57538,#57539,#57540,
#57541,#57542,#57543,#57544,#57545,#57546,#57547,#57548,#57549,#57550,#57551,
#57552,#57553,#57554,#57555,#57556,#57557),.UNSPECIFIED.,.F.,.F.,(4,3,3,
3,3,3,3,4),(189.61830102185,189.9191929278,190.91876762742,191.91834232704,
192.91791702666,193.91749172628,194.9170664259,195.901486329029),
 .UNSPECIFIED.);
#2615=B_SPLINE_CURVE_WITH_KNOTS('',3,(#57562,#57563,#57564,#57565,#57566,
#57567,#57568,#57569,#57570,#57571,#57572,#57573,#57574,#57575,#57576,#57577,
#57578,#57579,#57580,#57581,#57582,#57583,#57584,#57585,#57586),
 .UNSPECIFIED.,.F.,.F.,(4,3,3,3,3,3,3,3,4),(-205.153953350195,-204.9128134221,
-203.91323872248,-202.91366402286,-201.91408932324,-200.91451462362,-199.914939924,
-198.91536522438,-198.870768043016),.UNSPECIFIED.);
#2616=B_SPLINE_CURVE_WITH_KNOTS('',3,(#57587,#57588,#57589,#57590,#57591,
#57592,#57593,#57594,#57595,#57596,#57597,#57598,#57599,#57600,#57601,#57602,
#57603,#57604,#57605,#57606,#57607,#57608,#57609,#57610,#57611),
 .UNSPECIFIED.,.F.,.F.,(4,3,3,3,3,3,3,3,4),(195.901486329029,195.91664112552,
196.91621582514,197.91579052476,198.91536522438,199.914939924,200.91451462362,
201.91408932324,202.184671636209),.UNSPECIFIED.);
#2617=B_SPLINE_CURVE_WITH_KNOTS('',3,(#57616,#57617,#57618,#57619,#57620,
#57621,#57622,#57623,#57624,#57625,#57626,#57627,#57628,#57629,#57630,#57631,
#57632,#57633,#57634,#57635,#57636,#57637),.UNSPECIFIED.,.F.,.F.,(4,3,3,
3,3,3,3,4),(-211.437138657375,-210.91026161982,-209.9106869202,-208.91111222058,
-207.91153752096,-206.91196282134,-205.91238812172,-205.153953350195),
 .UNSPECIFIED.);
#2618=B_SPLINE_CURVE_WITH_KNOTS('',3,(#57638,#57639,#57640,#57641,#57642,
#57643,#57644,#57645,#57646,#57647,#57648,#57649,#57650,#57651,#57652,#57653,
#57654,#57655,#57656,#57657,#57658,#57659),.UNSPECIFIED.,.F.,.F.,(4,3,3,
3,3,3,3,4),(202.184671636209,202.91366402286,203.91323872248,204.9128134221,
205.91238812172,206.91196282134,207.91153752096,208.467856943389),
 .UNSPECIFIED.);
#2619=B_SPLINE_CURVE_WITH_KNOTS('',3,(#57664,#57665,#57666,#57667,#57668,
#57669,#57670,#57671,#57672,#57673,#57674,#57675,#57676,#57677,#57678,#57679,
#57680,#57681,#57682,#57683,#57684,#57685),.UNSPECIFIED.,.F.,.F.,(4,3,3,
3,3,3,3,4),(-217.720323964554,-216.90770981754,-215.90813511792,-214.9085604183,
-213.90898571868,-212.90941101906,-211.90983631944,-211.437138657375),
 .UNSPECIFIED.);
#2620=B_SPLINE_CURVE_WITH_KNOTS('',3,(#57686,#57687,#57688,#57689,#57690,
#57691,#57692,#57693,#57694,#57695,#57696,#57697,#57698,#57699,#57700,#57701,
#57702,#57703,#57704,#57705,#57706,#57707),.UNSPECIFIED.,.F.,.F.,(4,3,3,
3,3,3,3,4),(208.467856943389,208.91111222058,209.9106869202,210.91026161982,
211.90983631944,212.90941101906,213.90898571868,214.751042250568),
 .UNSPECIFIED.);
#2621=B_SPLINE_CURVE_WITH_KNOTS('',3,(#57712,#57713,#57714,#57715,#57716,
#57717,#57718,#57719,#57720,#57721,#57722,#57723,#57724,#57725,#57726,#57727,
#57728,#57729,#57730,#57731,#57732,#57733,#57734,#57735,#57736),
 .UNSPECIFIED.,.F.,.F.,(4,3,3,3,3,3,3,3,4),(-224.003509271734,-223.90473271488,
-222.90515801526,-221.90558331564,-220.90600861602,-219.9064339164,-218.90685921678,
-217.90728451716,-217.720323964554),.UNSPECIFIED.);
#2622=B_SPLINE_CURVE_WITH_KNOTS('',3,(#57737,#57738,#57739,#57740,#57741,
#57742,#57743,#57744,#57745,#57746,#57747,#57748,#57749,#57750,#57751,#57752,
#57753,#57754,#57755,#57756,#57757,#57758,#57759,#57760,#57761),
 .UNSPECIFIED.,.F.,.F.,(4,3,3,3,3,3,3,3,4),(214.751042250568,214.9085604183,
215.90813511792,216.90770981754,217.90728451716,218.90685921678,219.9064339164,
220.90600861602,221.034227557748),.UNSPECIFIED.);
#2623=B_SPLINE_CURVE_WITH_KNOTS('',3,(#57766,#57767,#57768,#57769,#57770,
#57771,#57772,#57773,#57774,#57775,#57776,#57777,#57778,#57779,#57780,#57781,
#57782,#57783,#57784,#57785,#57786,#57787),.UNSPECIFIED.,.F.,.F.,(4,3,3,
3,3,3,3,4),(-230.286694578913,-229.9021809126,-228.90260621298,-227.90303151336,
-226.90345681374,-225.90388211412,-224.9043074145,-224.003509271734),
 .UNSPECIFIED.);
#2624=B_SPLINE_CURVE_WITH_KNOTS('',3,(#57788,#57789,#57790,#57791,#57792,
#57793,#57794,#57795,#57796,#57797,#57798,#57799,#57800,#57801,#57802,#57803,
#57804,#57805,#57806,#57807,#57808,#57809),.UNSPECIFIED.,.F.,.F.,(4,3,3,
3,3,3,3,4),(221.034227557748,221.90558331564,222.90515801526,223.90473271488,
224.9043074145,225.90388211412,226.90345681374,227.317412864927),
 .UNSPECIFIED.);
#2625=B_SPLINE_CURVE_WITH_KNOTS('',3,(#57814,#57815,#57816,#57817,#57818,
#57819,#57820,#57821,#57822,#57823,#57824,#57825,#57826,#57827,#57828,#57829,
#57830,#57831,#57832,#57833,#57834,#57835),.UNSPECIFIED.,.F.,.F.,(4,3,3,
3,3,3,3,4),(-236.569879886093,-235.89962911032,-234.9000544107,-233.90047971108,
-232.90090501146,-231.90133031184,-230.90175561222,-230.286694578913),
 .UNSPECIFIED.);
#2626=B_SPLINE_CURVE_WITH_KNOTS('',3,(#57836,#57837,#57838,#57839,#57840,
#57841,#57842,#57843,#57844,#57845,#57846,#57847,#57848,#57849,#57850,#57851,
#57852,#57853,#57854,#57855,#57856,#57857),.UNSPECIFIED.,.F.,.F.,(4,3,3,
3,3,3,3,4),(227.317412864927,227.90303151336,228.90260621298,229.9021809126,
230.90175561222,231.90133031184,232.90090501146,233.600598172107),
 .UNSPECIFIED.);
#2627=B_SPLINE_CURVE_WITH_KNOTS('',3,(#57862,#57863,#57864,#57865,#57866,
#57867,#57868,#57869,#57870,#57871,#57872,#57873,#57874,#57875,#57876,#57877,
#57878,#57879,#57880,#57881,#57882,#57883),.UNSPECIFIED.,.F.,.F.,(4,3,3,
3,3,3,3,4),(-242.853065193272,-241.89707730804,-240.89750260842,-239.8979279088,
-238.89835320918,-237.89877850956,-236.89920380994,-236.569879886093),
 .UNSPECIFIED.);
#2628=B_SPLINE_CURVE_WITH_KNOTS('',3,(#57884,#57885,#57886,#57887,#57888,
#57889,#57890,#57891,#57892,#57893,#57894,#57895,#57896,#57897,#57898,#57899,
#57900,#57901,#57902,#57903,#57904,#57905),.UNSPECIFIED.,.F.,.F.,(4,3,3,
3,3,3,3,4),(233.600598172107,233.90047971108,234.9000544107,235.89962911032,
236.89920380994,237.89877850956,238.89835320918,239.883783479286),
 .UNSPECIFIED.);
#2629=B_SPLINE_CURVE_WITH_KNOTS('',3,(#57910,#57911,#57912,#57913,#57914,
#57915,#57916,#57917,#57918,#57919,#57920,#57921,#57922,#57923,#57924,#57925,
#57926,#57927,#57928,#57929,#57930,#57931,#57932,#57933,#57934),
 .UNSPECIFIED.,.F.,.F.,(4,3,3,3,3,3,3,3,4),(-249.136250500452,-248.89410020538,
-247.89452550576,-246.89495080614,-245.89537610652,-244.8958014069,-243.89622670728,
-242.89665200766,-242.853065193272),.UNSPECIFIED.);
#2630=B_SPLINE_CURVE_WITH_KNOTS('',3,(#57935,#57936,#57937,#57938,#57939,
#57940,#57941,#57942,#57943,#57944,#57945,#57946,#57947,#57948,#57949,#57950,
#57951,#57952,#57953,#57954,#57955,#57956,#57957,#57958,#57959),
 .UNSPECIFIED.,.F.,.F.,(4,3,3,3,3,3,3,3,4),(239.883783479286,239.8979279088,
240.89750260842,241.89707730804,242.89665200766,243.89622670728,244.8958014069,
245.89537610652,246.166968786466),.UNSPECIFIED.);
#2631=B_SPLINE_CURVE_WITH_KNOTS('',3,(#57964,#57965,#57966,#57967,#57968,
#57969,#57970,#57971,#57972,#57973,#57974,#57975,#57976,#57977,#57978,#57979,
#57980,#57981,#57982,#57983,#57984,#57985),.UNSPECIFIED.,.F.,.F.,(4,3,3,
3,3,3,3,4),(-255.419435807632,-254.8915484031,-253.89197370348,-252.89239900386,
-251.89282430424,-250.89324960462,-249.893674905,-249.136250500452),
 .UNSPECIFIED.);
#2632=B_SPLINE_CURVE_WITH_KNOTS('',3,(#57986,#57987,#57988,#57989,#57990,
#57991,#57992,#57993,#57994,#57995,#57996,#57997,#57998,#57999,#58000,#58001,
#58002,#58003,#58004,#58005,#58006,#58007),.UNSPECIFIED.,.F.,.F.,(4,3,3,
3,3,3,3,4),(246.166968786466,246.89495080614,247.89452550576,248.89410020538,
249.893674905,250.89324960462,251.89282430424,252.450154093645),
 .UNSPECIFIED.);
#2633=B_SPLINE_CURVE_WITH_KNOTS('',3,(#58012,#58013,#58014,#58015,#58016,
#58017,#58018,#58019,#58020,#58021,#58022,#58023,#58024,#58025,#58026,#58027,
#58028,#58029,#58030,#58031,#58032,#58033),.UNSPECIFIED.,.F.,.F.,(4,3,3,
3,3,3,3,4),(-261.702621114811,-260.88899660082,-259.8894219012,-258.88984720158,
-257.89027250196,-256.89069780234,-255.89112310272,-255.419435807632),
 .UNSPECIFIED.);
#2634=B_SPLINE_CURVE_WITH_KNOTS('',3,(#58034,#58035,#58036,#58037,#58038,
#58039,#58040,#58041,#58042,#58043,#58044,#58045,#58046,#58047,#58048,#58049,
#58050,#58051,#58052,#58053,#58054,#58055),.UNSPECIFIED.,.F.,.F.,(4,3,3,
3,3,3,3,4),(252.450154093645,252.89239900386,253.89197370348,254.8915484031,
255.89112310272,256.89069780234,257.89027250196,258.733339400825),
 .UNSPECIFIED.);
#2635=B_SPLINE_CURVE_WITH_KNOTS('',3,(#58060,#58061,#58062,#58063,#58064,
#58065,#58066,#58067,#58068,#58069,#58070,#58071,#58072,#58073,#58074,#58075,
#58076,#58077,#58078,#58079,#58080,#58081,#58082,#58083,#58084),
 .UNSPECIFIED.,.F.,.F.,(4,3,3,3,3,3,3,3,4),(-267.985806421991,-267.88601949816,
-266.88644479854,-265.88687009892,-264.8872953993,-263.88772069968,-262.88814600006,
-261.88857130044,-261.702621114811),.UNSPECIFIED.);
#2636=B_SPLINE_CURVE_WITH_KNOTS('',3,(#58085,#58086,#58087,#58088,#58089,
#58090,#58091,#58092,#58093,#58094,#58095,#58096,#58097,#58098,#58099,#58100,
#58101,#58102,#58103,#58104,#58105,#58106,#58107,#58108,#58109),
 .UNSPECIFIED.,.F.,.F.,(4,3,3,3,3,3,3,3,4),(258.733339400825,258.88984720158,
259.8894219012,260.88899660082,261.88857130044,262.88814600006,263.88772069968,
264.8872953993,265.016524708005),.UNSPECIFIED.);
#2637=B_SPLINE_CURVE_WITH_KNOTS('',3,(#58114,#58115,#58116,#58117,#58118,
#58119,#58120,#58121,#58122,#58123,#58124,#58125,#58126,#58127,#58128,#58129,
#58130,#58131,#58132,#58133,#58134,#58135),.UNSPECIFIED.,.F.,.F.,(4,3,3,
3,3,3,3,4),(-274.26899172917,-273.88346769588,-272.88389299626,-271.88431829664,
-270.88474359702,-269.8851688974,-268.88559419778,-267.985806421991),
 .UNSPECIFIED.);
#2638=B_SPLINE_CURVE_WITH_KNOTS('',3,(#58136,#58137,#58138,#58139,#58140,
#58141,#58142,#58143,#58144,#58145,#58146,#58147,#58148,#58149,#58150,#58151,
#58152,#58153,#58154,#58155,#58156,#58157),.UNSPECIFIED.,.F.,.F.,(4,3,3,
3,3,3,3,4),(265.016524708005,265.88687009892,266.88644479854,267.88601949816,
268.88559419778,269.8851688974,270.88474359702,271.299710015184),
 .UNSPECIFIED.);
#2639=B_SPLINE_CURVE_WITH_KNOTS('',3,(#58162,#58163,#58164,#58165,#58166,
#58167,#58168,#58169,#58170,#58171,#58172,#58173,#58174,#58175,#58176,#58177,
#58178,#58179,#58180,#58181,#58182,#58183),.UNSPECIFIED.,.F.,.F.,(4,3,3,
3,3,3,3,4),(-280.55217703635,-279.8809158936,-278.88134119398,-277.88176649436,
-276.88219179474,-275.88261709512,-274.8830423955,-274.26899172917),
 .UNSPECIFIED.);
#2640=B_SPLINE_CURVE_WITH_KNOTS('',3,(#58184,#58185,#58186,#58187,#58188,
#58189,#58190,#58191,#58192,#58193,#58194,#58195,#58196,#58197,#58198,#58199,
#58200,#58201,#58202,#58203,#58204,#58205),.UNSPECIFIED.,.F.,.F.,(4,3,3,
3,3,3,3,4),(271.299710015184,271.88431829664,272.88389299626,273.88346769588,
274.8830423955,275.88261709512,276.88219179474,277.582895322364),
 .UNSPECIFIED.);
#2641=B_SPLINE_CURVE_WITH_KNOTS('',3,(#58210,#58211,#58212,#58213,#58214,
#58215,#58216,#58217,#58218,#58219,#58220,#58221,#58222,#58223,#58224,#58225,
#58226,#58227,#58228,#58229,#58230,#58231),.UNSPECIFIED.,.F.,.F.,(4,3,3,
3,3,3,3,4),(-286.835362343529,-285.87836409132,-284.8787893917,-283.87921469208,
-282.87963999246,-281.88006529284,-280.88049059322,-280.55217703635),
 .UNSPECIFIED.);
#2642=B_SPLINE_CURVE_WITH_KNOTS('',3,(#58232,#58233,#58234,#58235,#58236,
#58237,#58238,#58239,#58240,#58241,#58242,#58243,#58244,#58245,#58246,#58247,
#58248,#58249,#58250,#58251,#58252,#58253),.UNSPECIFIED.,.F.,.F.,(4,3,3,
3,3,3,3,4),(277.582895322364,277.88176649436,278.88134119398,279.8809158936,
280.88049059322,281.88006529284,282.87963999246,283.866080629543),
 .UNSPECIFIED.);
#2643=B_SPLINE_CURVE_WITH_KNOTS('',3,(#58258,#58259,#58260,#58261,#58262,
#58263,#58264,#58265,#58266,#58267,#58268,#58269,#58270,#58271,#58272,#58273,
#58274,#58275,#58276,#58277,#58278,#58279,#58280,#58281,#58282),
 .UNSPECIFIED.,.F.,.F.,(4,3,3,3,3,3,3,3,4),(-293.118547650709,-292.87538698866,
-291.87581228904,-290.87623758942,-289.8766628898,-288.87708819018,-287.87751349056,
-286.87793879094,-286.835362343529),.UNSPECIFIED.);
#2644=B_SPLINE_CURVE_WITH_KNOTS('',3,(#58283,#58284,#58285,#58286,#58287,
#58288,#58289,#58290,#58291,#58292,#58293,#58294,#58295,#58296,#58297,#58298,
#58299,#58300,#58301,#58302,#58303,#58304,#58305,#58306,#58307),
 .UNSPECIFIED.,.F.,.F.,(4,3,3,3,3,3,3,3,4),(283.866080629543,283.87921469208,
284.8787893917,285.87836409132,286.87793879094,287.87751349056,288.87708819018,
289.8766628898,290.149265936723),.UNSPECIFIED.);
#2645=B_SPLINE_CURVE_WITH_KNOTS('',3,(#58312,#58313,#58314,#58315,#58316,
#58317,#58318,#58319,#58320,#58321,#58322,#58323,#58324,#58325,#58326,#58327,
#58328,#58329,#58330,#58331,#58332,#58333),.UNSPECIFIED.,.F.,.F.,(4,3,3,
3,3,3,3,4),(-299.401732957889,-298.87283518638,-297.87326048676,-296.87368578714,
-295.87411108752,-294.8745363879,-293.87496168828,-293.118547650709),
 .UNSPECIFIED.);
#2646=B_SPLINE_CURVE_WITH_KNOTS('',3,(#58334,#58335,#58336,#58337,#58338,
#58339,#58340,#58341,#58342,#58343,#58344,#58345,#58346,#58347,#58348,#58349,
#58350,#58351,#58352,#58353,#58354,#58355),.UNSPECIFIED.,.F.,.F.,(4,3,3,
3,3,3,3,4),(290.149265936723,290.87623758942,291.87581228904,292.87538698866,
293.87496168828,294.8745363879,295.87411108752,296.432451243902),
 .UNSPECIFIED.);
#2647=B_SPLINE_CURVE_WITH_KNOTS('',3,(#58360,#58361,#58362,#58363,#58364,
#58365,#58366,#58367,#58368,#58369,#58370,#58371,#58372,#58373,#58374,#58375,
#58376,#58377,#58378,#58379,#58380,#58381),.UNSPECIFIED.,.F.,.F.,(4,3,3,
3,3,3,3,4),(-305.684918265068,-304.8702833841,-303.87070868448,-302.87113398486,
-301.87155928524,-300.87198458562,-299.872409886,-299.401732957889),
 .UNSPECIFIED.);
#2648=B_SPLINE_CURVE_WITH_KNOTS('',3,(#58382,#58383,#58384,#58385,#58386,
#58387,#58388,#58389,#58390,#58391,#58392,#58393,#58394,#58395,#58396,#58397,
#58398,#58399,#58400,#58401,#58402,#58403),.UNSPECIFIED.,.F.,.F.,(4,3,3,
3,3,3,3,4),(296.432451243902,296.87368578714,297.87326048676,298.87283518638,
299.872409886,300.87198458562,301.87155928524,302.715636551082),
 .UNSPECIFIED.);
#2649=B_SPLINE_CURVE_WITH_KNOTS('',3,(#58408,#58409,#58410,#58411,#58412,
#58413,#58414,#58415,#58416,#58417,#58418,#58419,#58420,#58421,#58422,#58423,
#58424,#58425,#58426,#58427,#58428,#58429,#58430,#58431,#58432),
 .UNSPECIFIED.,.F.,.F.,(4,3,3,3,3,3,3,3,4),(-311.968103572248,-311.86730628144,
-310.867731581819,-309.868156882199,-308.868582182579,-307.86900748296,
-306.869432783339,-305.86985808372,-305.684918265068),.UNSPECIFIED.);
#2650=B_SPLINE_CURVE_WITH_KNOTS('',3,(#58433,#58434,#58435,#58436,#58437,
#58438,#58439,#58440,#58441,#58442,#58443,#58444,#58445,#58446,#58447,#58448,
#58449,#58450,#58451,#58452,#58453,#58454,#58455,#58456,#58457),
 .UNSPECIFIED.,.F.,.F.,(4,3,3,3,3,3,3,3,4),(302.715636551082,302.87113398486,
303.87070868448,304.8702833841,305.86985808372,306.86943278334,307.86900748296,
308.86858218258,308.998821858262),.UNSPECIFIED.);
#2651=B_SPLINE_CURVE_WITH_KNOTS('',3,(#58462,#58463,#58464,#58465,#58466,
#58467,#58468,#58469,#58470,#58471,#58472,#58473,#58474,#58475,#58476,#58477,
#58478,#58479,#58480,#58481,#58482,#58483),.UNSPECIFIED.,.F.,.F.,(4,3,3,
3,3,3,3,4),(-318.251288879427,-317.86475447916,-316.86517977954,-315.865605079919,
-314.866030380299,-313.86645568068,-312.866880981059,-311.968103572248),
 .UNSPECIFIED.);
#2652=B_SPLINE_CURVE_WITH_KNOTS('',3,(#58484,#58485,#58486,#58487,#58488,
#58489,#58490,#58491,#58492,#58493,#58494,#58495,#58496,#58497,#58498,#58499,
#58500,#58501,#58502,#58503,#58504,#58505),.UNSPECIFIED.,.F.,.F.,(4,3,3,
3,3,3,3,4),(308.998821858262,309.8681568822,310.86773158182,311.86730628144,
312.86688098106,313.86645568068,314.8660303803,315.282007165441),
 .UNSPECIFIED.);
#2653=B_SPLINE_CURVE_WITH_KNOTS('',3,(#58510,#58511,#58512,#58513,#58514,
#58515,#58516,#58517,#58518,#58519,#58520,#58521,#58522,#58523,#58524,#58525,
#58526,#58527,#58528,#58529,#58530,#58531),.UNSPECIFIED.,.F.,.F.,(4,3,3,
3,3,3,3,4),(-324.534474186607,-323.86220267688,-322.862627977259,-321.863053277639,
-320.86347857802,-319.8639038784,-318.864329178779,-318.251288879427),
 .UNSPECIFIED.);
#2654=B_SPLINE_CURVE_WITH_KNOTS('',3,(#58532,#58533,#58534,#58535,#58536,
#58537,#58538,#58539,#58540,#58541,#58542,#58543,#58544,#58545,#58546,#58547,
#58548,#58549,#58550,#58551,#58552,#58553),.UNSPECIFIED.,.F.,.F.,(4,3,3,
3,3,3,3,4),(315.282007165441,315.86560507992,316.86517977954,317.86475447916,
318.86432917878,319.8639038784,320.86347857802,321.565192472621),
 .UNSPECIFIED.);
#2655=B_SPLINE_CURVE_WITH_KNOTS('',3,(#58558,#58559,#58560,#58561,#58562,
#58563,#58564,#58565,#58566,#58567,#58568,#58569,#58570,#58571,#58572,#58573,
#58574,#58575,#58576,#58577,#58578,#58579),.UNSPECIFIED.,.F.,.F.,(4,3,3,
3,3,3,3,4),(-330.817659493786,-329.859650874599,-328.860076174979,-327.86050147536,
-326.860926775739,-325.861352076119,-324.8617773765,-324.534474186607),
 .UNSPECIFIED.);
#2656=B_SPLINE_CURVE_WITH_KNOTS('',3,(#58580,#58581,#58582,#58583,#58584,
#58585,#58586,#58587,#58588,#58589,#58590,#58591,#58592,#58593,#58594,#58595,
#58596,#58597,#58598,#58599,#58600,#58601),.UNSPECIFIED.,.F.,.F.,(4,3,3,
3,3,3,3,4),(321.565192472621,321.86305327764,322.86262797726,323.86220267688,
324.8617773765,325.86135207612,326.86092677574,327.8483777798),
 .UNSPECIFIED.);
#2657=B_SPLINE_CURVE_WITH_KNOTS('',3,(#58606,#58607,#58608,#58609,#58610,
#58611,#58612,#58613,#58614,#58615,#58616,#58617,#58618,#58619,#58620,#58621,
#58622,#58623,#58624,#58625,#58626,#58627,#58628,#58629,#58630),
 .UNSPECIFIED.,.F.,.F.,(4,3,3,3,3,3,3,3,4),(-337.100844800966,-336.85667377194,
-335.857099072319,-334.857524372699,-333.857949673079,-332.858374973459,
-331.858800273839,-330.859225574219,-330.817659493786),.UNSPECIFIED.);
#2658=B_SPLINE_CURVE_WITH_KNOTS('',3,(#58631,#58632,#58633,#58634,#58635,
#58636,#58637,#58638,#58639,#58640,#58641,#58642,#58643,#58644,#58645,#58646,
#58647,#58648,#58649,#58650,#58651,#58652,#58653,#58654,#58655),
 .UNSPECIFIED.,.F.,.F.,(4,3,3,3,3,3,3,3,4),(327.8483777798,327.86050147536,
328.86007617498,329.8596508746,330.85922557422,331.85880027384,332.85837497346,
333.85794967308,334.13156308698),.UNSPECIFIED.);
#2659=B_SPLINE_CURVE_WITH_KNOTS('',3,(#58660,#58661,#58662,#58663,#58664,
#58665,#58666,#58667,#58668,#58669,#58670,#58671,#58672,#58673,#58674,#58675,
#58676,#58677,#58678,#58679,#58680,#58681),.UNSPECIFIED.,.F.,.F.,(4,3,3,
3,3,3,3,4),(-343.384030108146,-342.854121969659,-341.85454727004,-340.854972570419,
-339.855397870799,-338.855823171179,-337.856248471559,-337.100844800966),
 .UNSPECIFIED.);
#2660=B_SPLINE_CURVE_WITH_KNOTS('',3,(#58682,#58683,#58684,#58685,#58686,
#58687,#58688,#58689,#58690,#58691,#58692,#58693,#58694,#58695,#58696,#58697,
#58698,#58699,#58700,#58701,#58702,#58703),.UNSPECIFIED.,.F.,.F.,(4,3,3,
3,3,3,3,4),(334.13156308698,334.8575243727,335.85709907232,336.85667377194,
337.85624847156,338.85582317118,339.8553978708,340.414748394159),
 .UNSPECIFIED.);
#2661=B_SPLINE_CURVE_WITH_KNOTS('',3,(#58708,#58709,#58710,#58711,#58712,
#58713,#58714,#58715,#58716,#58717,#58718,#58719,#58720,#58721,#58722,#58723,
#58724,#58725,#58726,#58727,#58728,#58729),.UNSPECIFIED.,.F.,.F.,(4,3,3,
3,3,3,3,4),(-349.667215415325,-348.851570167379,-347.851995467759,-346.852420768139,
-345.852846068519,-344.853271368899,-343.853696669279,-343.384030108146),
 .UNSPECIFIED.);
#2662=B_SPLINE_CURVE_WITH_KNOTS('',3,(#58730,#58731,#58732,#58733,#58734,
#58735,#58736,#58737,#58738,#58739,#58740,#58741,#58742,#58743,#58744,#58745,
#58746,#58747,#58748,#58749,#58750,#58751),.UNSPECIFIED.,.F.,.F.,(4,3,3,
3,3,3,3,4),(340.414748394159,340.85497257042,341.85454727004,342.85412196966,
343.85369666928,344.8532713689,345.85284606852,346.697933701339),
 .UNSPECIFIED.);
#2663=B_SPLINE_CURVE_WITH_KNOTS('',3,(#58756,#58757,#58758,#58759,#58760,
#58761,#58762,#58763,#58764,#58765,#58766,#58767,#58768,#58769,#58770,#58771,
#58772,#58773,#58774,#58775,#58776,#58777,#58778,#58779,#58780),
 .UNSPECIFIED.,.F.,.F.,(4,3,3,3,3,3,3,3,4),(-355.950400722505,-355.848593064719,
-354.849018365099,-353.849443665479,-352.849868965859,-351.850294266239,
-350.850719566619,-349.851144866999,-349.667215415325),.UNSPECIFIED.);
#2664=B_SPLINE_CURVE_WITH_KNOTS('',3,(#58781,#58782,#58783,#58784,#58785,
#58786,#58787,#58788,#58789,#58790,#58791,#58792,#58793,#58794,#58795,#58796,
#58797,#58798,#58799,#58800,#58801,#58802,#58803,#58804,#58805),
 .UNSPECIFIED.,.F.,.F.,(4,3,3,3,3,3,3,3,4),(346.697933701339,346.85242076814,
347.85199546776,348.85157016738,349.851144867,350.85071956662,351.85029426624,
352.84986896586,352.981119008518),.UNSPECIFIED.);
#2665=B_SPLINE_CURVE_WITH_KNOTS('',3,(#58810,#58811,#58812,#58813,#58814,
#58815,#58816,#58817,#58818,#58819,#58820,#58821,#58822,#58823,#58824,#58825,
#58826,#58827,#58828,#58829,#58830,#58831),.UNSPECIFIED.,.F.,.F.,(4,3,3,
3,3,3,3,4),(-362.233586029684,-361.846041262439,-360.846466562819,-359.846891863199,
-358.847317163579,-357.847742463959,-356.848167764339,-355.950400722505),
 .UNSPECIFIED.);
#2666=B_SPLINE_CURVE_WITH_KNOTS('',3,(#58832,#58833,#58834,#58835,#58836,
#58837,#58838,#58839,#58840,#58841,#58842,#58843,#58844,#58845,#58846,#58847,
#58848,#58849,#58850,#58851,#58852,#58853),.UNSPECIFIED.,.F.,.F.,(4,3,3,
3,3,3,3,4),(352.981119008518,353.84944366548,354.8490183651,355.84859306472,
356.84816776434,357.84774246396,358.84731716358,359.264304315698),
 .UNSPECIFIED.);
#2667=B_SPLINE_CURVE_WITH_KNOTS('',3,(#58858,#58859,#58860,#58861,#58862,
#58863,#58864,#58865,#58866,#58867,#58868,#58869,#58870,#58871,#58872,#58873,
#58874,#58875,#58876,#58877,#58878,#58879),.UNSPECIFIED.,.F.,.F.,(4,3,3,
3,3,3,3,4),(-368.516771336864,-367.843489460159,-366.843914760539,-365.844340060919,
-364.844765361299,-363.845190661679,-362.845615962059,-362.233586029684),
 .UNSPECIFIED.);
#2668=B_SPLINE_CURVE_WITH_KNOTS('',3,(#58880,#58881,#58882,#58883,#58884,
#58885,#58886,#58887,#58888,#58889,#58890,#58891,#58892,#58893,#58894,#58895,
#58896,#58897,#58898,#58899,#58900,#58901),.UNSPECIFIED.,.F.,.F.,(4,3,3,
3,3,3,3,4),(359.264304315698,359.8468918632,360.84646656282,361.84604126244,
362.84561596206,363.84519066168,364.8447653613,365.547489622878),
 .UNSPECIFIED.);
#2669=B_SPLINE_CURVE_WITH_KNOTS('',3,(#58906,#58907,#58908,#58909,#58910,
#58911,#58912,#58913,#58914,#58915,#58916,#58917,#58918,#58919,#58920,#58921,
#58922,#58923,#58924,#58925,#58926,#58927),.UNSPECIFIED.,.F.,.F.,(4,3,3,
3,3,3,3,4),(-374.799956644043,-373.840937657879,-372.841362958259,-371.841788258639,
-370.842213559019,-369.842638859399,-368.843064159779,-368.516771336864),
 .UNSPECIFIED.);
#2670=B_SPLINE_CURVE_WITH_KNOTS('',3,(#58928,#58929,#58930,#58931,#58932,
#58933,#58934,#58935,#58936,#58937,#58938,#58939,#58940,#58941,#58942,#58943,
#58944,#58945,#58946,#58947,#58948,#58949),.UNSPECIFIED.,.F.,.F.,(4,3,3,
3,3,3,3,4),(365.547489622878,365.84434006092,366.84391476054,367.84348946016,
368.84306415978,369.8426388594,370.84221355902,371.830674930057),
 .UNSPECIFIED.);
#2671=B_SPLINE_CURVE_WITH_KNOTS('',3,(#58954,#58955,#58956,#58957,#58958,
#58959,#58960,#58961,#58962,#58963,#58964,#58965,#58966,#58967,#58968,#58969,
#58970,#58971,#58972,#58973,#58974,#58975,#58976,#58977,#58978),
 .UNSPECIFIED.,.F.,.F.,(4,3,3,3,3,3,3,3,4),(-381.083141951223,-380.837960555219,
-379.838385855599,-378.838811155979,-377.839236456359,-376.839661756739,
-375.840087057119,-374.840512357499,-374.799956644043),.UNSPECIFIED.);
#2672=B_SPLINE_CURVE_WITH_KNOTS('',3,(#58979,#58980,#58981,#58982,#58983,
#58984,#58985,#58986,#58987,#58988,#58989,#58990,#58991,#58992,#58993,#58994,
#58995,#58996,#58997,#58998,#58999,#59000,#59001,#59002,#59003),
 .UNSPECIFIED.,.F.,.F.,(4,3,3,3,3,3,3,3,4),(371.830674930057,371.84178825864,
372.84136295826,373.84093765788,374.8405123575,375.84008705712,376.83966175674,
377.83923645636,378.113860237237),.UNSPECIFIED.);
#2673=B_SPLINE_CURVE_WITH_KNOTS('',3,(#59008,#59009,#59010,#59011,#59012,
#59013,#59014,#59015,#59016,#59017,#59018,#59019,#59020,#59021,#59022,#59023,
#59024,#59025,#59026,#59027,#59028,#59029),.UNSPECIFIED.,.F.,.F.,(4,3,3,
3,3,3,3,4),(-387.366327258402,-386.835408752939,-385.835834053319,-384.836259353699,
-383.836684654079,-382.837109954459,-381.837535254839,-381.083141951223),
 .UNSPECIFIED.);
#2674=B_SPLINE_CURVE_WITH_KNOTS('',3,(#59030,#59031,#59032,#59033,#59034,
#59035,#59036,#59037,#59038,#59039,#59040,#59041,#59042,#59043,#59044,#59045,
#59046,#59047,#59048,#59049,#59050,#59051),.UNSPECIFIED.,.F.,.F.,(4,3,3,
3,3,3,3,4),(378.113860237237,378.83881115598,379.8383858556,380.83796055522,
381.83753525484,382.83710995446,383.83668465408,384.397045544416),
 .UNSPECIFIED.);
#2675=B_SPLINE_CURVE_WITH_KNOTS('',3,(#59056,#59057,#59058,#59059,#59060,
#59061,#59062,#59063,#59064,#59065,#59066,#59067,#59068,#59069,#59070,#59071,
#59072,#59073,#59074,#59075,#59076,#59077),.UNSPECIFIED.,.F.,.F.,(4,3,3,
3,3,3,3,4),(-393.649512565582,-392.832856950659,-391.833282251039,-390.833707551419,
-389.834132851799,-388.834558152179,-387.834983452559,-387.366327258402),
 .UNSPECIFIED.);
#2676=B_SPLINE_CURVE_WITH_KNOTS('',3,(#59078,#59079,#59080,#59081,#59082,
#59083,#59084,#59085,#59086,#59087,#59088,#59089,#59090,#59091,#59092,#59093,
#59094,#59095,#59096,#59097,#59098,#59099),.UNSPECIFIED.,.F.,.F.,(4,3,3,
3,3,3,3,4),(384.397045544416,384.8362593537,385.83583405332,386.83540875294,
387.83498345256,388.83455815218,389.8341328518,390.680230851596),
 .UNSPECIFIED.);
#2677=B_SPLINE_CURVE_WITH_KNOTS('',3,(#59104,#59105,#59106,#59107,#59108,
#59109,#59110,#59111,#59112,#59113,#59114,#59115,#59116,#59117,#59118,#59119,
#59120,#59121,#59122,#59123,#59124,#59125,#59126,#59127,#59128),
 .UNSPECIFIED.,.F.,.F.,(4,3,3,3,3,3,3,3,4),(-399.932697872762,-399.829879847999,
-398.830305148379,-397.830730448759,-396.831155749139,-395.831581049519,
-394.832006349899,-393.832431650279,-393.649512565582),.UNSPECIFIED.);
#2678=B_SPLINE_CURVE_WITH_KNOTS('',3,(#59129,#59130,#59131,#59132,#59133,
#59134,#59135,#59136,#59137,#59138,#59139,#59140,#59141,#59142,#59143,#59144,
#59145,#59146,#59147,#59148,#59149,#59150,#59151,#59152,#59153),
 .UNSPECIFIED.,.F.,.F.,(4,3,3,3,3,3,3,3,4),(390.680230851596,390.83370755142,
391.83328225104,392.83285695066,393.83243165028,394.8320063499,395.83158104952,
396.83115574914,396.963416158775),.UNSPECIFIED.);
#2679=B_SPLINE_CURVE_WITH_KNOTS('',3,(#59158,#59159,#59160,#59161,#59162,
#59163,#59164,#59165,#59166,#59167,#59168,#59169,#59170,#59171,#59172,#59173,
#59174,#59175,#59176,#59177,#59178,#59179),.UNSPECIFIED.,.F.,.F.,(4,3,3,
3,3,3,3,4),(-406.215883179941,-405.827328045719,-404.827753346099,-403.828178646479,
-402.828603946859,-401.829029247239,-400.829454547619,-399.932697872762),
 .UNSPECIFIED.);
#2680=B_SPLINE_CURVE_WITH_KNOTS('',3,(#59180,#59181,#59182,#59183,#59184,
#59185,#59186,#59187,#59188,#59189,#59190,#59191,#59192,#59193,#59194,#59195,
#59196,#59197,#59198,#59199,#59200,#59201),.UNSPECIFIED.,.F.,.F.,(4,3,3,
3,3,3,3,4),(396.963416158775,397.83073044876,398.83030514838,399.829879848,
400.82945454762,401.82902924724,402.82860394686,403.246601465955),
 .UNSPECIFIED.);
#2681=B_SPLINE_CURVE_WITH_KNOTS('',3,(#59206,#59207,#59208,#59209,#59210,
#59211,#59212,#59213,#59214,#59215,#59216,#59217,#59218,#59219,#59220,#59221,
#59222,#59223,#59224,#59225,#59226,#59227),.UNSPECIFIED.,.F.,.F.,(4,3,3,
3,3,3,3,4),(-412.499068487121,-411.824776243439,-410.825201543819,-409.825626844199,
-408.826052144579,-407.826477444959,-406.826902745339,-406.215883179941),
 .UNSPECIFIED.);
#2682=B_SPLINE_CURVE_WITH_KNOTS('',3,(#59228,#59229,#59230,#59231,#59232,
#59233,#59234,#59235,#59236,#59237,#59238,#59239,#59240,#59241,#59242,#59243,
#59244,#59245,#59246,#59247,#59248,#59249),.UNSPECIFIED.,.F.,.F.,(4,3,3,
3,3,3,3,4),(403.246601465955,403.82817864648,404.8277533461,405.82732804572,
406.82690274534,407.82647744496,408.82605214458,409.529786773135),
 .UNSPECIFIED.);
#2683=B_SPLINE_CURVE_WITH_KNOTS('',3,(#59254,#59255,#59256,#59257,#59258,
#59259,#59260,#59261,#59262,#59263,#59264,#59265,#59266,#59267,#59268,#59269,
#59270,#59271,#59272,#59273,#59274,#59275),.UNSPECIFIED.,.F.,.F.,(4,3,3,
3,3,3,3,4),(-418.7822537943,-417.822224441159,-416.822649741539,-415.823075041919,
-414.823500342299,-413.823925642679,-412.824350943059,-412.499068487121),
 .UNSPECIFIED.);
#2684=B_SPLINE_CURVE_WITH_KNOTS('',3,(#59276,#59277,#59278,#59279,#59280,
#59281,#59282,#59283,#59284,#59285,#59286,#59287,#59288,#59289,#59290,#59291,
#59292,#59293,#59294,#59295,#59296,#59297),.UNSPECIFIED.,.F.,.F.,(4,3,3,
3,3,3,3,4),(409.529786773135,409.8256268442,410.82520154382,411.82477624344,
412.82435094306,413.82392564268,414.8235003423,415.812972080314),
 .UNSPECIFIED.);
#2685=B_SPLINE_CURVE_WITH_KNOTS('',3,(#59302,#59303,#59304,#59305,#59306,
#59307,#59308,#59309,#59310,#59311,#59312,#59313,#59314,#59315,#59316,#59317,
#59318,#59319,#59320,#59321,#59322,#59323,#59324,#59325,#59326),
 .UNSPECIFIED.,.F.,.F.,(4,3,3,3,3,3,3,3,4),(-425.06543910148,-424.819247338499,
-423.819672638879,-422.820097939259,-421.820523239639,-420.820948540019,
-419.821373840399,-418.821799140779,-418.7822537943),.UNSPECIFIED.);
#2686=B_SPLINE_CURVE_WITH_KNOTS('',3,(#59327,#59328,#59329,#59330,#59331,
#59332,#59333,#59334,#59335,#59336,#59337,#59338,#59339,#59340,#59341,#59342,
#59343,#59344,#59345,#59346,#59347,#59348,#59349,#59350,#59351),
 .UNSPECIFIED.,.F.,.F.,(4,3,3,3,3,3,3,3,4),(415.812972080314,415.82307504192,
416.82264974154,417.82222444116,418.82179914078,419.8213738404,420.82094854002,
421.82052323964,422.096157387494),.UNSPECIFIED.);
#2687=B_SPLINE_CURVE_WITH_KNOTS('',3,(#59356,#59357,#59358,#59359,#59360,
#59361,#59362,#59363,#59364,#59365,#59366,#59367,#59368,#59369,#59370,#59371,
#59372,#59373,#59374,#59375,#59376,#59377),.UNSPECIFIED.,.F.,.F.,(4,3,3,
3,3,3,3,4),(-431.348624408659,-430.816695536219,-429.817120836599,-428.817546136979,
-427.817971437359,-426.818396737739,-425.818822038119,-425.06543910148),
 .UNSPECIFIED.);
#2688=B_SPLINE_CURVE_WITH_KNOTS('',3,(#59378,#59379,#59380,#59381,#59382,
#59383,#59384,#59385,#59386,#59387,#59388,#59389,#59390,#59391,#59392,#59393,
#59394,#59395,#59396,#59397,#59398,#59399),.UNSPECIFIED.,.F.,.F.,(4,3,3,
3,3,3,3,4),(422.096157387494,422.82009793926,423.81967263888,424.8192473385,
425.81882203812,426.81839673774,427.81797143736,428.379342694673),
 .UNSPECIFIED.);
#2689=B_SPLINE_CURVE_WITH_KNOTS('',3,(#59405,#59406,#59407,#59408,#59409),
 .UNSPECIFIED.,.F.,.F.,(4,1,4),(442.964564156161,443.432209983341,444.357761408881),
 .UNSPECIFIED.);
#2690=B_SPLINE_CURVE_WITH_KNOTS('',3,(#59412,#59413,#59414,#59415),
 .UNSPECIFIED.,.F.,.F.,(4,4),(442.964564156161,443.117030489009),
 .UNSPECIFIED.);
#2691=B_SPLINE_CURVE_WITH_KNOTS('',3,(#59420,#59421,#59422,#59423,#59424,
#59425,#59426,#59427,#59428,#59429),.UNSPECIFIED.,.F.,.F.,(4,1,1,1,1,1,
1,4),(436.681378848981,437.434761785621,438.434336485241,439.433911184861,
440.433485884481,441.433060584101,442.432635283721,442.964564156161),
 .UNSPECIFIED.);
#2692=B_SPLINE_CURVE_WITH_KNOTS('',3,(#59430,#59431,#59432,#59433,#59434,
#59435,#59436,#59437,#59438,#59439),.UNSPECIFIED.,.F.,.F.,(4,1,1,1,1,1,
1,4),(436.681378848981,437.119582291289,438.119156990909,439.118731690529,
440.118306390149,441.117881089769,442.117455789389,442.964564156161),
 .UNSPECIFIED.);
#2693=B_SPLINE_CURVE_WITH_KNOTS('',3,(#59444,#59445,#59446,#59447,#59448,
#59449,#59450,#59451,#59452,#59453,#59454),.UNSPECIFIED.,.F.,.F.,(4,1,1,
1,1,1,1,1,4),(430.398193541801,430.437738888281,431.437313587901,432.436888287521,
433.436462987141,434.436037686761,435.435612386381,436.435187086001,436.681378848981),
 .UNSPECIFIED.);
#2694=B_SPLINE_CURVE_WITH_KNOTS('',3,(#59455,#59456,#59457,#59458,#59459,
#59460,#59461,#59462,#59463,#59464),.UNSPECIFIED.,.F.,.F.,(4,1,1,1,1,1,
1,4),(430.398193541802,431.122134093569,432.121708793189,433.121283492809,
434.120858192429,435.120432892049,436.120007591669,436.681378848981),
 .UNSPECIFIED.);
#2695=B_SPLINE_CURVE_WITH_KNOTS('',3,(#59469,#59470,#59471,#59472,#59473,
#59474,#59475,#59476,#59477,#59478),.UNSPECIFIED.,.F.,.F.,(4,1,1,1,1,1,
1,4),(424.115008234622,424.440290690561,425.439865390181,426.439440089801,
427.439014789421,428.438589489041,429.438164188661,430.398193541801),
 .UNSPECIFIED.);
#2696=B_SPLINE_CURVE_WITH_KNOTS('',3,(#59479,#59480,#59481,#59482,#59483,
#59484,#59485,#59486,#59487,#59488,#59489),.UNSPECIFIED.,.F.,.F.,(4,1,1,
1,1,1,1,1,4),(424.115008234622,424.125111196229,425.124685895849,426.124260595469,
427.123835295089,428.123409994709,429.122984694329,430.122559393949,430.398193541802),
 .UNSPECIFIED.);
#2697=B_SPLINE_CURVE_WITH_KNOTS('',3,(#59494,#59495,#59496,#59497,#59498,
#59499,#59500,#59501,#59502,#59503),.UNSPECIFIED.,.F.,.F.,(4,1,1,1,1,1,
1,4),(417.831822927442,418.442842492841,419.442417192461,420.441991892081,
421.441566591701,422.441141291321,423.440715990941,424.115008234622),
 .UNSPECIFIED.);
#2698=B_SPLINE_CURVE_WITH_KNOTS('',3,(#59504,#59505,#59506,#59507,#59508,
#59509,#59510,#59511,#59512,#59513),.UNSPECIFIED.,.F.,.F.,(4,1,1,1,1,1,
1,4),(417.831822927443,418.127662998509,419.127237698129,420.126812397749,
421.126387097369,422.125961796989,423.125536496609,424.115008234622),
 .UNSPECIFIED.);
#2699=B_SPLINE_CURVE_WITH_KNOTS('',3,(#59518,#59519,#59520,#59521,#59522,
#59523,#59524,#59525,#59526,#59527),.UNSPECIFIED.,.F.,.F.,(4,1,1,1,1,1,
1,4),(411.548637620263,412.445394295121,413.444968994741,414.444543694361,
415.444118393981,416.443693093601,417.443267793221,417.831822927442),
 .UNSPECIFIED.);
#2700=B_SPLINE_CURVE_WITH_KNOTS('',3,(#59528,#59529,#59530,#59531,#59532,
#59533,#59534,#59535,#59536,#59537),.UNSPECIFIED.,.F.,.F.,(4,1,1,1,1,1,
1,4),(411.548637620263,412.130214800789,413.129789500409,414.129364200029,
415.128938899649,416.128513599269,417.128088298889,417.831822927443),
 .UNSPECIFIED.);
#2701=B_SPLINE_CURVE_WITH_KNOTS('',3,(#59542,#59543,#59544,#59545,#59546,
#59547,#59548,#59549,#59550,#59551,#59552),.UNSPECIFIED.,.F.,.F.,(4,1,1,
1,1,1,1,1,4),(405.265452313083,405.448371397781,406.447946097401,407.447520797021,
408.447095496641,409.446670196261,410.446244895881,411.445819595501,411.548637620263),
 .UNSPECIFIED.);
#2702=B_SPLINE_CURVE_WITH_KNOTS('',3,(#59553,#59554,#59555,#59556,#59557,
#59558,#59559,#59560,#59561,#59562),.UNSPECIFIED.,.F.,.F.,(4,1,1,1,1,1,
1,4),(405.265452313083,406.132766603069,407.132341302689,408.131916002309,
409.131490701929,410.131065401549,411.130640101169,411.548637620263),
 .UNSPECIFIED.);
#2703=B_SPLINE_CURVE_WITH_KNOTS('',3,(#59567,#59568,#59569,#59570,#59571,
#59572,#59573,#59574,#59575,#59576),.UNSPECIFIED.,.F.,.F.,(4,1,1,1,1,1,
1,4),(398.982267005904,399.450923200061,400.450497899681,401.450072599301,
402.449647298921,403.449221998541,404.448796698161,405.265452313083),
 .UNSPECIFIED.);
#2704=B_SPLINE_CURVE_WITH_KNOTS('',3,(#59577,#59578,#59579,#59580,#59581,
#59582,#59583,#59584,#59585,#59586,#59587),.UNSPECIFIED.,.F.,.F.,(4,1,1,
1,1,1,1,1,4),(398.982267005904,399.135743705729,400.135318405349,401.134893104969,
402.134467804589,403.134042504209,404.133617203829,405.133191903449,405.265452313083),
 .UNSPECIFIED.);
#2705=B_SPLINE_CURVE_WITH_KNOTS('',3,(#59592,#59593,#59594,#59595,#59596,
#59597,#59598,#59599,#59600,#59601),.UNSPECIFIED.,.F.,.F.,(4,1,1,1,1,1,
1,4),(392.699081698724,393.453475002341,394.453049701961,395.452624401581,
396.452199101201,397.451773800821,398.451348500441,398.982267005904),
 .UNSPECIFIED.);
#2706=B_SPLINE_CURVE_WITH_KNOTS('',3,(#59602,#59603,#59604,#59605,#59606,
#59607,#59608,#59609,#59610,#59611),.UNSPECIFIED.,.F.,.F.,(4,1,1,1,1,1,
1,4),(392.699081698724,393.138295508009,394.137870207629,395.137444907249,
396.137019606869,397.136594306489,398.136169006109,398.982267005904),
 .UNSPECIFIED.);
#2707=B_SPLINE_CURVE_WITH_KNOTS('',3,(#59616,#59617,#59618,#59619,#59620,
#59621,#59622,#59623,#59624,#59625,#59626),.UNSPECIFIED.,.F.,.F.,(4,1,1,
1,1,1,1,1,4),(386.415896391544,386.456452105001,387.456026804621,388.455601504241,
389.455176203861,390.454750903481,391.454325603101,392.453900302721,392.699081698724),
 .UNSPECIFIED.);
#2708=B_SPLINE_CURVE_WITH_KNOTS('',3,(#59627,#59628,#59629,#59630,#59631,
#59632,#59633,#59634,#59635,#59636),.UNSPECIFIED.,.F.,.F.,(4,1,1,1,1,1,
1,4),(386.415896391545,387.140847310289,388.140422009909,389.139996709529,
390.139571409149,391.139146108769,392.138720808389,392.699081698724),
 .UNSPECIFIED.);
#2709=B_SPLINE_CURVE_WITH_KNOTS('',3,(#59641,#59642,#59643,#59644,#59645,
#59646,#59647,#59648,#59649,#59650),.UNSPECIFIED.,.F.,.F.,(4,1,1,1,1,1,
1,4),(380.132711084365,380.459003907281,381.458578606901,382.458153306521,
383.457728006141,384.457302705761,385.456877405381,386.415896391544),
 .UNSPECIFIED.);
#2710=B_SPLINE_CURVE_WITH_KNOTS('',3,(#59651,#59652,#59653,#59654,#59655,
#59656,#59657,#59658,#59659,#59660,#59661),.UNSPECIFIED.,.F.,.F.,(4,1,1,
1,1,1,1,1,4),(380.132711084365,380.143824412949,381.143399112569,382.142973812189,
383.142548511809,384.142123211429,385.141697911049,386.141272610669,386.415896391545),
 .UNSPECIFIED.);
#2711=B_SPLINE_CURVE_WITH_KNOTS('',3,(#59666,#59667,#59668,#59669,#59670,
#59671,#59672,#59673,#59674,#59675),.UNSPECIFIED.,.F.,.F.,(4,1,1,1,1,1,
1,4),(373.849525777185,374.461555709561,375.461130409181,376.460705108801,
377.460279808421,378.459854508041,379.459429207661,380.132711084365),
 .UNSPECIFIED.);
#2712=B_SPLINE_CURVE_WITH_KNOTS('',3,(#59676,#59677,#59678,#59679,#59680,
#59681,#59682,#59683,#59684,#59685),.UNSPECIFIED.,.F.,.F.,(4,1,1,1,1,1,
1,4),(373.849525777185,374.146376215229,375.145950914849,376.145525614469,
377.145100314089,378.144675013709,379.144249713329,380.132711084365),
 .UNSPECIFIED.);
#2713=B_SPLINE_CURVE_WITH_KNOTS('',3,(#59690,#59691,#59692,#59693,#59694,
#59695,#59696,#59697,#59698,#59699),.UNSPECIFIED.,.F.,.F.,(4,1,1,1,1,1,
1,4),(367.566340470006,368.464107511841,369.463682211461,370.463256911081,
371.462831610701,372.462406310321,373.461981009941,373.849525777185),
 .UNSPECIFIED.);
#2714=B_SPLINE_CURVE_WITH_KNOTS('',3,(#59700,#59701,#59702,#59703,#59704,
#59705,#59706,#59707,#59708,#59709),.UNSPECIFIED.,.F.,.F.,(4,1,1,1,1,1,
1,4),(367.566340470006,368.148928017509,369.148502717129,370.148077416749,
371.147652116369,372.147226815989,373.146801515609,373.849525777185),
 .UNSPECIFIED.);
#2715=B_SPLINE_CURVE_WITH_KNOTS('',3,(#59714,#59715,#59716,#59717,#59718,
#59719,#59720,#59721,#59722,#59723,#59724),.UNSPECIFIED.,.F.,.F.,(4,1,1,
1,1,1,1,1,4),(361.283155162826,361.467084614501,362.466659314121,363.466234013741,
364.465808713361,365.465383412981,366.464958112601,367.464532812221,367.566340470006),
 .UNSPECIFIED.);
#2716=B_SPLINE_CURVE_WITH_KNOTS('',3,(#59725,#59726,#59727,#59728,#59729,
#59730,#59731,#59732,#59733,#59734),.UNSPECIFIED.,.F.,.F.,(4,1,1,1,1,1,
1,4),(361.283155162826,362.151479819789,363.151054519409,364.150629219029,
365.150203918649,366.149778618269,367.149353317889,367.566340470006),
 .UNSPECIFIED.);
#2717=B_SPLINE_CURVE_WITH_KNOTS('',3,(#59739,#59740,#59741,#59742,#59743,
#59744,#59745,#59746,#59747,#59748),.UNSPECIFIED.,.F.,.F.,(4,1,1,1,1,1,
1,4),(354.999969855647,355.469636416781,356.469211116401,357.468785816021,
358.468360515641,359.467935215261,360.467509914881,361.283155162826),
 .UNSPECIFIED.);
#2718=B_SPLINE_CURVE_WITH_KNOTS('',3,(#59749,#59750,#59751,#59752,#59753,
#59754,#59755,#59756,#59757,#59758,#59759),.UNSPECIFIED.,.F.,.F.,(4,1,1,
1,1,1,1,1,4),(354.999969855647,355.154456922449,356.154031622069,357.153606321689,
358.153181021309,359.152755720929,360.152330420549,361.151905120169,361.283155162826),
 .UNSPECIFIED.);
#2719=B_SPLINE_CURVE_WITH_KNOTS('',3,(#59764,#59765,#59766,#59767,#59768,
#59769,#59770,#59771,#59772,#59773),.UNSPECIFIED.,.F.,.F.,(4,1,1,1,1,1,
1,4),(348.716784548467,349.472188219061,350.471762918681,351.471337618301,
352.470912317921,353.470487017541,354.470061717161,354.999969855647),
 .UNSPECIFIED.);
#2720=B_SPLINE_CURVE_WITH_KNOTS('',3,(#59774,#59775,#59776,#59777,#59778,
#59779,#59780,#59781,#59782,#59783),.UNSPECIFIED.,.F.,.F.,(4,1,1,1,1,1,
1,4),(348.716784548467,349.157008724729,350.156583424349,351.156158123969,
352.155732823589,353.155307523209,354.154882222829,354.999969855647),
 .UNSPECIFIED.);
#2721=B_SPLINE_CURVE_WITH_KNOTS('',3,(#59788,#59789,#59790,#59791,#59792,
#59793,#59794,#59795,#59796,#59797,#59798),.UNSPECIFIED.,.F.,.F.,(4,1,1,
1,1,1,1,1,4),(342.433599241287,342.475165321721,343.474740021341,344.474314720961,
345.473889420581,346.473464120201,347.473038819821,348.472613519441,348.716784548467),
 .UNSPECIFIED.);
#2722=B_SPLINE_CURVE_WITH_KNOTS('',3,(#59799,#59800,#59801,#59802,#59803,
#59804,#59805,#59806,#59807,#59808),.UNSPECIFIED.,.F.,.F.,(4,1,1,1,1,1,
1,4),(342.433599241288,343.159560527009,344.159135226629,345.158709926249,
346.158284625869,347.157859325489,348.157434025109,348.716784548467),
 .UNSPECIFIED.);
#2723=B_SPLINE_CURVE_WITH_KNOTS('',3,(#59813,#59814,#59815,#59816,#59817,
#59818,#59819,#59820,#59821,#59822),.UNSPECIFIED.,.F.,.F.,(4,1,1,1,1,1,
1,4),(336.150413934108,336.477717124001,337.477291823621,338.476866523241,
339.476441222861,340.476015922481,341.475590622101,342.433599241287),
 .UNSPECIFIED.);
#2724=B_SPLINE_CURVE_WITH_KNOTS('',3,(#59823,#59824,#59825,#59826,#59827,
#59828,#59829,#59830,#59831,#59832,#59833),.UNSPECIFIED.,.F.,.F.,(4,1,1,
1,1,1,1,1,4),(336.150413934108,336.162537629669,337.162112329289,338.161687028909,
339.161261728529,340.160836428149,341.160411127769,342.159985827389,342.433599241288),
 .UNSPECIFIED.);
#2725=B_SPLINE_CURVE_WITH_KNOTS('',3,(#59838,#59839,#59840,#59841,#59842,
#59843,#59844,#59845,#59846,#59847),.UNSPECIFIED.,.F.,.F.,(4,1,1,1,1,1,
1,4),(329.867228626928,330.480268926281,331.479843625901,332.479418325521,
333.478993025141,334.478567724761,335.478142424381,336.150413934108),
 .UNSPECIFIED.);
#2726=B_SPLINE_CURVE_WITH_KNOTS('',3,(#59848,#59849,#59850,#59851,#59852,
#59853,#59854,#59855,#59856,#59857),.UNSPECIFIED.,.F.,.F.,(4,1,1,1,1,1,
1,4),(329.867228626929,330.165089431949,331.164664131569,332.164238831189,
333.163813530809,334.163388230429,335.162962930049,336.150413934108),
 .UNSPECIFIED.);
#2727=B_SPLINE_CURVE_WITH_KNOTS('',3,(#59862,#59863,#59864,#59865,#59866,
#59867,#59868,#59869,#59870,#59871),.UNSPECIFIED.,.F.,.F.,(4,1,1,1,1,1,
1,4),(323.584043319749,324.482820728561,325.482395428181,326.481970127801,
327.481544827421,328.481119527041,329.480694226661,329.867228626928),
 .UNSPECIFIED.);
#2728=B_SPLINE_CURVE_WITH_KNOTS('',3,(#59872,#59873,#59874,#59875,#59876,
#59877,#59878,#59879,#59880,#59881),.UNSPECIFIED.,.F.,.F.,(4,1,1,1,1,1,
1,4),(323.584043319749,324.167641234229,325.167215933849,326.166790633469,
327.166365333089,328.165940032709,329.165514732329,329.867228626929),
 .UNSPECIFIED.);
#2729=B_SPLINE_CURVE_WITH_KNOTS('',3,(#59886,#59887,#59888,#59889,#59890,
#59891,#59892,#59893,#59894,#59895,#59896),.UNSPECIFIED.,.F.,.F.,(4,1,1,
1,1,1,1,1,4),(317.300858012569,317.485797831221,318.485372530841,319.484947230461,
320.484521930081,321.484096629701,322.483671329321,323.483246028941,323.584043319749),
 .UNSPECIFIED.);
#2730=B_SPLINE_CURVE_WITH_KNOTS('',3,(#59897,#59898,#59899,#59900,#59901,
#59902,#59903,#59904,#59905,#59906),.UNSPECIFIED.,.F.,.F.,(4,1,1,1,1,1,
1,4),(317.300858012569,318.170193036509,319.169767736129,320.169342435749,
321.168917135369,322.168491834989,323.168066534609,323.584043319749),
 .UNSPECIFIED.);
#2731=B_SPLINE_CURVE_WITH_KNOTS('',3,(#59911,#59912,#59913,#59914,#59915,
#59916,#59917,#59918,#59919,#59920),.UNSPECIFIED.,.F.,.F.,(4,1,1,1,1,1,
1,4),(311.01767270539,311.488349633501,312.487924333121,313.487499032741,
314.487073732361,315.486648431981,316.486223131601,317.300858012569),
 .UNSPECIFIED.);
#2732=B_SPLINE_CURVE_WITH_KNOTS('',3,(#59921,#59922,#59923,#59924,#59925,
#59926,#59927,#59928,#59929,#59930,#59931),.UNSPECIFIED.,.F.,.F.,(4,1,1,
1,1,1,1,1,4),(311.01767270539,311.173170139169,312.172744838789,313.172319538409,
314.171894238029,315.171468937649,316.171043637269,317.170618336889,317.300858012569),
 .UNSPECIFIED.);
#2733=B_SPLINE_CURVE_WITH_KNOTS('',3,(#59936,#59937,#59938,#59939,#59940,
#59941,#59942,#59943,#59944,#59945),.UNSPECIFIED.,.F.,.F.,(4,1,1,1,1,1,
1,4),(304.73448739821,305.490901435781,306.490476135401,307.490050835021,
308.489625534641,309.489200234261,310.488774933881,311.01767270539),
 .UNSPECIFIED.);
#2734=B_SPLINE_CURVE_WITH_KNOTS('',3,(#59946,#59947,#59948,#59949,#59950,
#59951,#59952,#59953,#59954,#59955),.UNSPECIFIED.,.F.,.F.,(4,1,1,1,1,1,
1,4),(304.73448739821,305.175721941449,306.175296641069,307.174871340689,
308.174446040309,309.174020739929,310.173595439549,311.01767270539),
 .UNSPECIFIED.);
#2735=B_SPLINE_CURVE_WITH_KNOTS('',3,(#59960,#59961,#59962,#59963,#59964,
#59965,#59966,#59967,#59968,#59969,#59970),.UNSPECIFIED.,.F.,.F.,(4,1,1,
1,1,1,1,1,4),(298.451302091031,298.493878538441,299.493453238061,300.493027937681,
301.492602637301,302.492177336921,303.491752036541,304.491326736161,304.73448739821),
 .UNSPECIFIED.);
#2736=B_SPLINE_CURVE_WITH_KNOTS('',3,(#59971,#59972,#59973,#59974,#59975,
#59976,#59977,#59978,#59979,#59980),.UNSPECIFIED.,.F.,.F.,(4,1,1,1,1,1,
1,4),(298.451302091031,299.178273743729,300.177848443349,301.177423142969,
302.176997842589,303.176572542209,304.176147241829,304.73448739821),
 .UNSPECIFIED.);
#2737=B_SPLINE_CURVE_WITH_KNOTS('',3,(#59985,#59986,#59987,#59988,#59989,
#59990,#59991,#59992,#59993,#59994),.UNSPECIFIED.,.F.,.F.,(4,1,1,1,1,1,
1,4),(292.168116783851,292.496430340721,293.496005040341,294.495579739961,
295.495154439581,296.494729139201,297.494303838821,298.451302091031),
 .UNSPECIFIED.);
#2738=B_SPLINE_CURVE_WITH_KNOTS('',3,(#59995,#59996,#59997,#59998,#59999,
#60000,#60001,#60002,#60003,#60004,#60005),.UNSPECIFIED.,.F.,.F.,(4,1,1,
1,1,1,1,1,4),(292.168116783851,292.181250846389,293.180825546009,294.180400245629,
295.179974945249,296.179549644869,297.179124344489,298.178699044109,298.451302091031),
 .UNSPECIFIED.);
#2739=B_SPLINE_CURVE_WITH_KNOTS('',3,(#60010,#60011,#60012,#60013,#60014,
#60015,#60016,#60017,#60018,#60019),.UNSPECIFIED.,.F.,.F.,(4,1,1,1,1,1,
1,4),(285.884931476671,286.498982143001,287.498556842621,288.498131542241,
289.497706241861,290.497280941481,291.496855641101,292.168116783851),
 .UNSPECIFIED.);
#2740=B_SPLINE_CURVE_WITH_KNOTS('',3,(#60020,#60021,#60022,#60023,#60024,
#60025,#60026,#60027,#60028,#60029),.UNSPECIFIED.,.F.,.F.,(4,1,1,1,1,1,
1,4),(285.884931476672,286.183802648669,287.183377348289,288.182952047909,
289.182526747529,290.182101447149,291.181676146769,292.168116783851),
 .UNSPECIFIED.);
#2741=B_SPLINE_CURVE_WITH_KNOTS('',3,(#60034,#60035,#60036,#60037,#60038,
#60039,#60040,#60041,#60042,#60043),.UNSPECIFIED.,.F.,.F.,(4,1,1,1,1,1,
1,4),(279.601746169492,280.501533945281,281.501108644901,282.500683344521,
283.500258044141,284.499832743761,285.499407443381,285.884931476671),
 .UNSPECIFIED.);
#2742=B_SPLINE_CURVE_WITH_KNOTS('',3,(#60044,#60045,#60046,#60047,#60048,
#60049,#60050,#60051,#60052,#60053),.UNSPECIFIED.,.F.,.F.,(4,1,1,1,1,1,
1,4),(279.601746169492,280.186354450949,281.185929150569,282.185503850189,
283.185078549809,284.184653249429,285.184227949049,285.884931476672),
 .UNSPECIFIED.);
#2743=B_SPLINE_CURVE_WITH_KNOTS('',3,(#60058,#60059,#60060,#60061,#60062,
#60063,#60064,#60065,#60066,#60067,#60068),.UNSPECIFIED.,.F.,.F.,(4,1,1,
1,1,1,1,1,4),(273.318560862312,273.504511047941,274.504085747561,275.503660447181,
276.503235146801,277.502809846421,278.502384546041,279.501959245661,279.601746169492),
 .UNSPECIFIED.);
#2744=B_SPLINE_CURVE_WITH_KNOTS('',3,(#60069,#60070,#60071,#60072,#60073,
#60074,#60075,#60076,#60077,#60078),.UNSPECIFIED.,.F.,.F.,(4,1,1,1,1,1,
1,4),(273.318560862312,274.188906253229,275.188480952849,276.188055652469,
277.187630352089,278.187205051709,279.186779751329,279.601746169492),
 .UNSPECIFIED.);
#2745=B_SPLINE_CURVE_WITH_KNOTS('',3,(#60083,#60084,#60085,#60086,#60087,
#60088,#60089,#60090,#60091,#60092),.UNSPECIFIED.,.F.,.F.,(4,1,1,1,1,1,
1,4),(267.035375555133,267.507062850221,268.506637549841,269.506212249461,
270.505786949081,271.505361648701,272.504936348321,273.318560862312),
 .UNSPECIFIED.);
#2746=B_SPLINE_CURVE_WITH_KNOTS('',3,(#60093,#60094,#60095,#60096,#60097,
#60098,#60099,#60100,#60101,#60102,#60103),.UNSPECIFIED.,.F.,.F.,(4,1,1,
1,1,1,1,1,4),(267.035375555133,267.191883355889,268.191458055509,269.191032755129,
270.190607454749,271.190182154369,272.189756853989,273.189331553609,273.318560862312),
 .UNSPECIFIED.);
#2747=B_SPLINE_CURVE_WITH_KNOTS('',3,(#60108,#60109,#60110,#60111,#60112,
#60113,#60114,#60115,#60116,#60117),.UNSPECIFIED.,.F.,.F.,(4,1,1,1,1,1,
1,4),(260.752190247953,261.509614652501,262.509189352121,263.508764051741,
264.508338751361,265.507913450981,266.507488150601,267.035375555133),
 .UNSPECIFIED.);
#2748=B_SPLINE_CURVE_WITH_KNOTS('',3,(#60118,#60119,#60120,#60121,#60122,
#60123,#60124,#60125,#60126,#60127),.UNSPECIFIED.,.F.,.F.,(4,1,1,1,1,1,
1,4),(260.752190247953,261.194435158169,262.194009857789,263.193584557409,
264.193159257029,265.192733956649,266.192308656269,267.035375555133),
 .UNSPECIFIED.);
#2749=B_SPLINE_CURVE_WITH_KNOTS('',3,(#60132,#60133,#60134,#60135,#60136,
#60137,#60138,#60139,#60140,#60141,#60142),.UNSPECIFIED.,.F.,.F.,(4,1,1,
1,1,1,1,1,4),(254.469004940774,254.512591755161,255.512166454781,256.511741154401,
257.511315854021,258.510890553641,259.510465253261,260.510039952881,260.752190247953),
 .UNSPECIFIED.);
#2750=B_SPLINE_CURVE_WITH_KNOTS('',3,(#60143,#60144,#60145,#60146,#60147,
#60148,#60149,#60150,#60151,#60152),.UNSPECIFIED.,.F.,.F.,(4,1,1,1,1,1,
1,4),(254.469004940774,255.196986960449,256.196561660069,257.196136359689,
258.195711059309,259.195285758929,260.194860458549,260.752190247953),
 .UNSPECIFIED.);
#2751=B_SPLINE_CURVE_WITH_KNOTS('',3,(#60157,#60158,#60159,#60160,#60161,
#60162,#60163,#60164,#60165,#60166),.UNSPECIFIED.,.F.,.F.,(4,1,1,1,1,1,
1,4),(248.185819633594,248.515143557441,249.514718257061,250.514292956681,
251.513867656301,252.513442355921,253.513017055541,254.469004940774),
 .UNSPECIFIED.);
#2752=B_SPLINE_CURVE_WITH_KNOTS('',3,(#60167,#60168,#60169,#60170,#60171,
#60172,#60173,#60174,#60175,#60176,#60177),.UNSPECIFIED.,.F.,.F.,(4,1,1,
1,1,1,1,1,4),(248.185819633594,248.199964063109,249.199538762729,250.199113462349,
251.198688161969,252.198262861589,253.197837561209,254.197412260829,254.469004940774),
 .UNSPECIFIED.);
#2753=B_SPLINE_CURVE_WITH_KNOTS('',3,(#60182,#60183,#60184,#60185,#60186,
#60187,#60188,#60189,#60190,#60191),.UNSPECIFIED.,.F.,.F.,(4,1,1,1,1,1,
1,4),(241.902634326414,242.517695359721,243.517270059341,244.516844758961,
245.516419458581,246.515994158201,247.515568857821,248.185819633594),
 .UNSPECIFIED.);
#2754=B_SPLINE_CURVE_WITH_KNOTS('',3,(#60192,#60193,#60194,#60195,#60196,
#60197,#60198,#60199,#60200,#60201),.UNSPECIFIED.,.F.,.F.,(4,1,1,1,1,1,
1,4),(241.902634326415,242.202515865389,243.202090565009,244.201665264629,
245.201239964249,246.200814663869,247.200389363489,248.185819633594),
 .UNSPECIFIED.);
#2755=B_SPLINE_CURVE_WITH_KNOTS('',3,(#60206,#60207,#60208,#60209,#60210,
#60211,#60212,#60213,#60214,#60215),.UNSPECIFIED.,.F.,.F.,(4,1,1,1,1,1,
1,4),(235.619449019235,236.520247162001,237.519821861621,238.519396561241,
239.518971260861,240.518545960481,241.518120660101,241.902634326414),
 .UNSPECIFIED.);
#2756=B_SPLINE_CURVE_WITH_KNOTS('',3,(#60216,#60217,#60218,#60219,#60220,
#60221,#60222,#60223,#60224,#60225),.UNSPECIFIED.,.F.,.F.,(4,1,1,1,1,1,
1,4),(235.619449019235,236.205067667669,237.204642367289,238.204217066909,
239.203791766529,240.203366466149,241.202941165769,241.902634326415),
 .UNSPECIFIED.);
#2757=B_SPLINE_CURVE_WITH_KNOTS('',3,(#60230,#60231,#60232,#60233,#60234,
#60235,#60236,#60237,#60238,#60239,#60240),.UNSPECIFIED.,.F.,.F.,(4,1,1,
1,1,1,1,1,4),(229.336263712055,229.523224264661,230.522798964281,231.522373663901,
232.521948363521,233.521523063141,234.521097762761,235.520672462381,235.619449019235),
 .UNSPECIFIED.);
#2758=B_SPLINE_CURVE_WITH_KNOTS('',3,(#60241,#60242,#60243,#60244,#60245,
#60246,#60247,#60248,#60249,#60250),.UNSPECIFIED.,.F.,.F.,(4,1,1,1,1,1,
1,4),(229.336263712056,230.207619469949,231.207194169569,232.206768869189,
233.206343568809,234.205918268429,235.205492968049,235.619449019235),
 .UNSPECIFIED.);
#2759=B_SPLINE_CURVE_WITH_KNOTS('',3,(#60255,#60256,#60257,#60258,#60259,
#60260,#60261,#60262,#60263,#60264),.UNSPECIFIED.,.F.,.F.,(4,1,1,1,1,1,
1,4),(223.053078404876,223.525776066941,224.525350766561,225.524925466181,
226.524500165801,227.524074865421,228.523649565041,229.336263712055),
 .UNSPECIFIED.);
#2760=B_SPLINE_CURVE_WITH_KNOTS('',3,(#60265,#60266,#60267,#60268,#60269,
#60270,#60271,#60272,#60273,#60274,#60275),.UNSPECIFIED.,.F.,.F.,(4,1,1,
1,1,1,1,1,4),(223.053078404876,223.210596572609,224.210171272229,225.209745971849,
226.209320671469,227.208895371089,228.208470070709,229.208044770329,229.336263712056),
 .UNSPECIFIED.);
#2761=B_SPLINE_CURVE_WITH_KNOTS('',3,(#60280,#60281,#60282,#60283,#60284,
#60285,#60286,#60287,#60288,#60289),.UNSPECIFIED.,.F.,.F.,(4,1,1,1,1,1,
1,4),(216.769893097696,217.528327869221,218.527902568841,219.527477268461,
220.527051968081,221.526626667701,222.526201367321,223.053078404876),
 .UNSPECIFIED.);
#2762=B_SPLINE_CURVE_WITH_KNOTS('',3,(#60290,#60291,#60292,#60293,#60294,
#60295,#60296,#60297,#60298,#60299),.UNSPECIFIED.,.F.,.F.,(4,1,1,1,1,1,
1,4),(216.769893097696,217.213148374889,218.212723074509,219.212297774129,
220.211872473749,221.211447173369,222.211021872989,223.053078404876),
 .UNSPECIFIED.);
#2763=B_SPLINE_CURVE_WITH_KNOTS('',3,(#60304,#60305,#60306,#60307,#60308,
#60309,#60310,#60311,#60312,#60313,#60314),.UNSPECIFIED.,.F.,.F.,(4,1,1,
1,1,1,1,1,4),(210.486707790517,210.531304971881,211.530879671501,212.530454371121,
213.530029070741,214.529603770361,215.529178469981,216.528753169601,216.769893097696),
 .UNSPECIFIED.);
#2764=B_SPLINE_CURVE_WITH_KNOTS('',3,(#60315,#60316,#60317,#60318,#60319,
#60320,#60321,#60322,#60323,#60324),.UNSPECIFIED.,.F.,.F.,(4,1,1,1,1,1,
1,4),(210.486707790517,211.215700177169,212.215274876789,213.214849576409,
214.214424276029,215.213998975649,216.213573675269,216.769893097696),
 .UNSPECIFIED.);
#2765=B_SPLINE_CURVE_WITH_KNOTS('',3,(#60329,#60330,#60331,#60332,#60333,
#60334,#60335,#60336,#60337,#60338),.UNSPECIFIED.,.F.,.F.,(4,1,1,1,1,1,
1,4),(204.203522483337,204.533856774161,205.533431473781,206.533006173401,
207.532580873021,208.532155572641,209.531730272261,210.486707790517),
 .UNSPECIFIED.);
#2766=B_SPLINE_CURVE_WITH_KNOTS('',3,(#60339,#60340,#60341,#60342,#60343,
#60344,#60345,#60346,#60347,#60348,#60349),.UNSPECIFIED.,.F.,.F.,(4,1,1,
1,1,1,1,1,4),(204.203522483337,204.218677279829,205.218251979449,206.217826679069,
207.217401378689,208.216976078309,209.216550777929,210.216125477549,210.486707790517),
 .UNSPECIFIED.);
#2767=B_SPLINE_CURVE_WITH_KNOTS('',3,(#60354,#60355,#60356,#60357,#60358,
#60359,#60360,#60361,#60362,#60363),.UNSPECIFIED.,.F.,.F.,(4,1,1,1,1,1,
1,4),(197.920337176158,198.536408576441,199.535983276061,200.535557975681,
201.535132675301,202.534707374921,203.534282074541,204.203522483337),
 .UNSPECIFIED.);
#2768=B_SPLINE_CURVE_WITH_KNOTS('',3,(#60364,#60365,#60366,#60367,#60368,
#60369,#60370,#60371,#60372,#60373),.UNSPECIFIED.,.F.,.F.,(4,1,1,1,1,1,
1,4),(197.920337176158,198.221229082109,199.220803781729,200.220378481349,
201.219953180969,202.219527880589,203.219102580209,204.203522483337),
 .UNSPECIFIED.);
#2769=B_SPLINE_CURVE_WITH_KNOTS('',3,(#60378,#60379,#60380,#60381,#60382,
#60383,#60384,#60385,#60386,#60387),.UNSPECIFIED.,.F.,.F.,(4,1,1,1,1,1,
1,4),(191.637151868978,192.538960378721,193.538535078341,194.538109777961,
195.537684477581,196.537259177201,197.536833876821,197.920337176158),
 .UNSPECIFIED.);
#2770=B_SPLINE_CURVE_WITH_KNOTS('',3,(#60388,#60389,#60390,#60391,#60392,
#60393,#60394,#60395,#60396,#60397),.UNSPECIFIED.,.F.,.F.,(4,1,1,1,1,1,
1,4),(191.637151868978,192.223780884389,193.223355584009,194.222930283629,
195.222504983249,196.222079682869,197.221654382489,197.920337176158),
 .UNSPECIFIED.);
#2771=B_SPLINE_CURVE_WITH_KNOTS('',3,(#60402,#60403,#60404,#60405,#60406,
#60407,#60408,#60409,#60410,#60411,#60412),.UNSPECIFIED.,.F.,.F.,(4,1,1,
1,1,1,1,1,4),(185.353966561798,185.541937481381,186.541512181001,187.541086880621,
188.540661580241,189.540236279861,190.539810979481,191.539385679101,191.637151868978),
 .UNSPECIFIED.);
#2772=B_SPLINE_CURVE_WITH_KNOTS('',3,(#60413,#60414,#60415,#60416,#60417,
#60418,#60419,#60420,#60421,#60422),.UNSPECIFIED.,.F.,.F.,(4,1,1,1,1,1,
1,4),(185.353966561799,186.226332686669,187.225907386289,188.225482085909,
189.225056785529,190.224631485149,191.224206184769,191.637151868978),
 .UNSPECIFIED.);
#2773=B_SPLINE_CURVE_WITH_KNOTS('',3,(#60427,#60428,#60429,#60430,#60431,
#60432,#60433,#60434,#60435,#60436),.UNSPECIFIED.,.F.,.F.,(4,1,1,1,1,1,
1,4),(179.070781254619,179.544489283661,180.544063983281,181.543638682901,
182.543213382521,183.542788082141,184.542362781761,185.353966561798),
 .UNSPECIFIED.);
#2774=B_SPLINE_CURVE_WITH_KNOTS('',3,(#60437,#60438,#60439,#60440,#60441,
#60442,#60443,#60444,#60445,#60446,#60447),.UNSPECIFIED.,.F.,.F.,(4,1,1,
1,1,1,1,1,4),(179.070781254619,179.229309789329,180.228884488949,181.228459188569,
182.228033888189,183.227608587809,184.227183287429,185.226757987049,185.353966561799),
 .UNSPECIFIED.);
#2775=B_SPLINE_CURVE_WITH_KNOTS('',3,(#60452,#60453,#60454,#60455,#60456,
#60457,#60458,#60459,#60460,#60461),.UNSPECIFIED.,.F.,.F.,(4,1,1,1,1,1,
1,4),(172.787595947439,173.547041085941,174.546615785561,175.546190485181,
176.545765184801,177.545339884421,178.544914584041,179.070781254619),
 .UNSPECIFIED.);
#2776=B_SPLINE_CURVE_WITH_KNOTS('',3,(#60462,#60463,#60464,#60465,#60466,
#60467,#60468,#60469,#60470,#60471),.UNSPECIFIED.,.F.,.F.,(4,1,1,1,1,1,
1,4),(172.78759594744,173.231861591609,174.231436291229,175.231010990849,
176.230585690469,177.230160390089,178.229735089709,179.070781254619),
 .UNSPECIFIED.);
#2777=B_SPLINE_CURVE_WITH_KNOTS('',3,(#60476,#60477,#60478,#60479,#60480,
#60481,#60482,#60483,#60484,#60485,#60486),.UNSPECIFIED.,.F.,.F.,(4,1,1,
1,1,1,1,1,4),(166.50441064026,166.550018188601,167.549592888221,168.549167587841,
169.548742287461,170.548316987081,171.547891686701,172.547466386321,172.787595947439),
 .UNSPECIFIED.);
#2778=B_SPLINE_CURVE_WITH_KNOTS('',3,(#60487,#60488,#60489,#60490,#60491,
#60492,#60493,#60494,#60495,#60496),.UNSPECIFIED.,.F.,.F.,(4,1,1,1,1,1,
1,4),(166.50441064026,167.234413393889,168.233988093509,169.233562793129,
170.233137492749,171.232712192369,172.232286891989,172.78759594744),
 .UNSPECIFIED.);
#2779=B_SPLINE_CURVE_WITH_KNOTS('',3,(#60501,#60502,#60503,#60504,#60505,
#60506,#60507,#60508,#60509,#60510),.UNSPECIFIED.,.F.,.F.,(4,1,1,1,1,1,
1,4),(160.22122533308,160.552569990881,161.552144690501,162.551719390121,
163.551294089741,164.550868789361,165.550443488981,166.50441064026),
 .UNSPECIFIED.);
#2780=B_SPLINE_CURVE_WITH_KNOTS('',3,(#60511,#60512,#60513,#60514,#60515,
#60516,#60517,#60518,#60519,#60520,#60521),.UNSPECIFIED.,.F.,.F.,(4,1,1,
1,1,1,1,1,4),(160.22122533308,160.237390496549,161.236965196169,162.236539895789,
163.236114595409,164.235689295029,165.235263994649,166.234838694269,166.50441064026),
 .UNSPECIFIED.);
#2781=B_SPLINE_CURVE_WITH_KNOTS('',3,(#60526,#60527,#60528,#60529,#60530,
#60531,#60532,#60533,#60534,#60535),.UNSPECIFIED.,.F.,.F.,(4,1,1,1,1,1,
1,4),(153.938040025901,154.555121793161,155.554696492781,156.554271192401,
157.553845892021,158.553420591641,159.552995291261,160.22122533308),
 .UNSPECIFIED.);
#2782=B_SPLINE_CURVE_WITH_KNOTS('',3,(#60536,#60537,#60538,#60539,#60540,
#60541,#60542,#60543,#60544,#60545),.UNSPECIFIED.,.F.,.F.,(4,1,1,1,1,1,
1,4),(153.938040025901,154.239942298829,155.239516998449,156.239091698069,
157.238666397689,158.238241097309,159.237815796929,160.22122533308),
 .UNSPECIFIED.);
#2783=B_SPLINE_CURVE_WITH_KNOTS('',3,(#60550,#60551,#60552,#60553,#60554,
#60555,#60556,#60557,#60558,#60559),.UNSPECIFIED.,.F.,.F.,(4,1,1,1,1,1,
1,4),(147.654854718721,148.557673595441,149.557248295061,150.556822994681,
151.556397694301,152.555972393921,153.555547093541,153.938040025901),
 .UNSPECIFIED.);
#2784=B_SPLINE_CURVE_WITH_KNOTS('',3,(#60560,#60561,#60562,#60563,#60564,
#60565,#60566,#60567,#60568,#60569),.UNSPECIFIED.,.F.,.F.,(4,1,1,1,1,1,
1,4),(147.654854718721,148.242494101109,149.242068800729,150.241643500349,
151.241218199969,152.240792899589,153.240367599209,153.938040025901),
 .UNSPECIFIED.);
#2785=B_SPLINE_CURVE_WITH_KNOTS('',3,(#60574,#60575,#60576,#60577,#60578,
#60579,#60580,#60581,#60582,#60583,#60584),.UNSPECIFIED.,.F.,.F.,(4,1,1,
1,1,1,1,1,4),(141.371669411541,141.560650698101,142.560225397721,143.559800097341,
144.559374796961,145.558949496581,146.558524196201,147.558098895821,147.654854718721),
 .UNSPECIFIED.);
#2786=B_SPLINE_CURVE_WITH_KNOTS('',3,(#60585,#60586,#60587,#60588,#60589,
#60590,#60591,#60592,#60593,#60594),.UNSPECIFIED.,.F.,.F.,(4,1,1,1,1,1,
1,4),(141.371669411542,142.245045903389,143.244620603009,144.244195302629,
145.243770002249,146.243344701869,147.242919401489,147.654854718721),
 .UNSPECIFIED.);
#2787=B_SPLINE_CURVE_WITH_KNOTS('',3,(#60599,#60600,#60601,#60602,#60603,
#60604,#60605,#60606,#60607,#60608),.UNSPECIFIED.,.F.,.F.,(4,1,1,1,1,1,
1,4),(135.088484104362,135.563202500381,136.562777200001,137.562351899621,
138.561926599241,139.561501298861,140.561075998481,141.371669411541),
 .UNSPECIFIED.);
#2788=B_SPLINE_CURVE_WITH_KNOTS('',3,(#60609,#60610,#60611,#60612,#60613,
#60614,#60615,#60616,#60617,#60618,#60619),.UNSPECIFIED.,.F.,.F.,(4,1,1,
1,1,1,1,1,4),(135.088484104362,135.248023006049,136.247597705669,137.247172405289,
138.246747104909,139.246321804529,140.245896504149,141.245471203769,141.371669411542),
 .UNSPECIFIED.);
#2789=B_SPLINE_CURVE_WITH_KNOTS('',3,(#60624,#60625,#60626,#60627,#60628,
#60629,#60630,#60631,#60632,#60633),.UNSPECIFIED.,.F.,.F.,(4,1,1,1,1,1,
1,4),(128.805298797182,129.565754302661,130.565329002281,131.564903701901,
132.564478401521,133.564053101141,134.563627800761,135.088484104362),
 .UNSPECIFIED.);
#2790=B_SPLINE_CURVE_WITH_KNOTS('',3,(#60634,#60635,#60636,#60637,#60638,
#60639,#60640,#60641,#60642,#60643),.UNSPECIFIED.,.F.,.F.,(4,1,1,1,1,1,
1,4),(128.805298797183,129.250574808329,130.250149507949,131.249724207569,
132.249298907189,133.248873606809,134.248448306429,135.088484104362),
 .UNSPECIFIED.);
#2791=B_SPLINE_CURVE_WITH_KNOTS('',3,(#60648,#60649,#60650,#60651,#60652,
#60653,#60654,#60655,#60656,#60657,#60658),.UNSPECIFIED.,.F.,.F.,(4,1,1,
1,1,1,1,1,4),(122.522113490003,122.568731405321,123.568306104941,124.567880804561,
125.567455504181,126.567030203801,127.566604903421,128.566179603041,128.805298797182),
 .UNSPECIFIED.);
#2792=B_SPLINE_CURVE_WITH_KNOTS('',3,(#60659,#60660,#60661,#60662,#60663,
#60664,#60665,#60666,#60667,#60668),.UNSPECIFIED.,.F.,.F.,(4,1,1,1,1,1,
1,4),(122.522113490003,123.253126610609,124.252701310229,125.252276009849,
126.251850709469,127.251425409089,128.251000108709,128.805298797183),
 .UNSPECIFIED.);
#2793=B_SPLINE_CURVE_WITH_KNOTS('',3,(#60673,#60674,#60675,#60676,#60677,
#60678,#60679,#60680,#60681,#60682),.UNSPECIFIED.,.F.,.F.,(4,1,1,1,1,1,
1,4),(116.238928182823,116.571283207601,117.570857907221,118.570432606841,
119.570007306461,120.569582006081,121.569156705701,122.522113490003),
 .UNSPECIFIED.);
#2794=B_SPLINE_CURVE_WITH_KNOTS('',3,(#60683,#60684,#60685,#60686,#60687,
#60688,#60689,#60690,#60691,#60692,#60693),.UNSPECIFIED.,.F.,.F.,(4,1,1,
1,1,1,1,1,4),(116.238928182823,116.256103713269,117.255678412889,118.255253112509,
119.254827812129,120.254402511749,121.253977211369,122.253551910989,122.522113490003),
 .UNSPECIFIED.);
#2795=B_SPLINE_CURVE_WITH_KNOTS('',3,(#60698,#60699,#60700,#60701,#60702,
#60703,#60704,#60705,#60706,#60707),.UNSPECIFIED.,.F.,.F.,(4,1,1,1,1,1,
1,4),(109.955742875644,110.573835009881,111.573409709501,112.572984409121,
113.572559108741,114.572133808361,115.571708507981,116.238928182823),
 .UNSPECIFIED.);
#2796=B_SPLINE_CURVE_WITH_KNOTS('',3,(#60708,#60709,#60710,#60711,#60712,
#60713,#60714,#60715,#60716,#60717),.UNSPECIFIED.,.F.,.F.,(4,1,1,1,1,1,
1,4),(109.955742875644,110.258655515549,111.258230215169,112.257804914789,
113.257379614409,114.256954314029,115.256529013649,116.238928182823),
 .UNSPECIFIED.);
#2797=B_SPLINE_CURVE_WITH_KNOTS('',3,(#60722,#60723,#60724,#60725,#60726,
#60727,#60728,#60729,#60730,#60731),.UNSPECIFIED.,.F.,.F.,(4,1,1,1,1,1,
1,4),(103.672557568464,104.576386812161,105.575961511781,106.575536211401,
107.575110911021,108.574685610641,109.574260310261,109.955742875644),
 .UNSPECIFIED.);
#2798=B_SPLINE_CURVE_WITH_KNOTS('',3,(#60732,#60733,#60734,#60735,#60736,
#60737,#60738,#60739,#60740,#60741),.UNSPECIFIED.,.F.,.F.,(4,1,1,1,1,1,
1,4),(103.672557568464,104.261207317829,105.260782017449,106.260356717069,
107.259931416689,108.259506116309,109.259080815929,109.955742875644),
 .UNSPECIFIED.);
#2799=B_SPLINE_CURVE_WITH_KNOTS('',3,(#60746,#60747,#60748,#60749,#60750,
#60751,#60752,#60753,#60754,#60755,#60756),.UNSPECIFIED.,.F.,.F.,(4,1,1,
1,1,1,1,1,4),(97.3893722612844,97.5793639148213,98.5789386144413,99.5785133140613,
100.578088013681,101.577662713301,102.577237412921,103.576812112541,103.672557568464),
 .UNSPECIFIED.);
#2800=B_SPLINE_CURVE_WITH_KNOTS('',3,(#60757,#60758,#60759,#60760,#60761,
#60762,#60763,#60764,#60765,#60766),.UNSPECIFIED.,.F.,.F.,(4,1,1,1,1,1,
1,4),(97.3893722612846,98.2637591201091,99.2633338197291,100.262908519349,
101.262483218969,102.262057918589,103.261632618209,103.672557568464),
 .UNSPECIFIED.);
#2801=B_SPLINE_CURVE_WITH_KNOTS('',3,(#60771,#60772,#60773,#60774,#60775,
#60776,#60777,#60778,#60779,#60780),.UNSPECIFIED.,.F.,.F.,(4,1,1,1,1,1,
1,4),(91.1061869541047,91.5819157171013,92.5814904167213,93.5810651163413,
94.5806398159613,95.5802145155813,96.5797892152013,97.3893722612844),
 .UNSPECIFIED.);
#2802=B_SPLINE_CURVE_WITH_KNOTS('',3,(#60781,#60782,#60783,#60784,#60785,
#60786,#60787,#60788,#60789,#60790,#60791),.UNSPECIFIED.,.F.,.F.,(4,1,1,
1,1,1,1,1,4),(91.106186954105,91.2667362227691,92.2663109223891,93.2658856220091,
94.265460321629,95.265035021249,96.264609720869,97.264184420489,97.3893722612846),
 .UNSPECIFIED.);
#2803=B_SPLINE_CURVE_WITH_KNOTS('',3,(#60796,#60797,#60798,#60799,#60800,
#60801,#60802,#60803,#60804,#60805),.UNSPECIFIED.,.F.,.F.,(4,1,1,1,1,1,
1,4),(84.8230016469252,85.5844675193813,86.5840422190013,87.5836169186213,
88.5831916182413,89.5827663178613,90.5823410174813,91.1061869541047),
 .UNSPECIFIED.);
#2804=B_SPLINE_CURVE_WITH_KNOTS('',3,(#60806,#60807,#60808,#60809,#60810,
#60811,#60812,#60813,#60814,#60815),.UNSPECIFIED.,.F.,.F.,(4,1,1,1,1,1,
1,4),(84.8230016469254,85.2692880250491,86.2688627246691,87.2684374242891,
88.2680121239091,89.2675868235291,90.2671615231491,91.106186954105),
 .UNSPECIFIED.);
#2805=B_SPLINE_CURVE_WITH_KNOTS('',3,(#60820,#60821,#60822,#60823,#60824,
#60825,#60826,#60827,#60828,#60829,#60830),.UNSPECIFIED.,.F.,.F.,(4,1,1,
1,1,1,1,1,4),(78.5398163397456,78.5874446220413,79.5870193216613,80.5865940212813,
81.5861687209013,82.5857434205213,83.5853181201413,84.5848928197613,84.8230016469252),
 .UNSPECIFIED.);
#2806=B_SPLINE_CURVE_WITH_KNOTS('',3,(#60831,#60832,#60833,#60834,#60835,
#60836,#60837,#60838,#60839,#60840),.UNSPECIFIED.,.F.,.F.,(4,1,1,1,1,1,
1,4),(78.5398163397458,79.2718398273291,80.2714145269491,81.2709892265691,
82.2705639261891,83.2701386258091,84.2697133254291,84.8230016469254),
 .UNSPECIFIED.);
#2807=B_SPLINE_CURVE_WITH_KNOTS('',3,(#60845,#60846,#60847,#60848,#60849,
#60850,#60851,#60852,#60853,#60854),.UNSPECIFIED.,.F.,.F.,(4,1,1,1,1,1,
1,4),(72.256631032566,72.5899964243213,73.5895711239413,74.5891458235613,
75.5887205231813,76.5882952228013,77.5878699224213,78.5398163397456),
 .UNSPECIFIED.);
#2808=B_SPLINE_CURVE_WITH_KNOTS('',3,(#60855,#60856,#60857,#60858,#60859,
#60860,#60861,#60862,#60863,#60864,#60865),.UNSPECIFIED.,.F.,.F.,(4,1,1,
1,1,1,1,1,4),(72.2566310325662,72.2748169299891,73.2743916296091,74.2739663292291,
75.2735410288491,76.2731157284691,77.2726904280891,78.2722651277091,78.5398163397458),
 .UNSPECIFIED.);
#2809=B_SPLINE_CURVE_WITH_KNOTS('',3,(#60870,#60871,#60872,#60873,#60874,
#60875,#60876,#60877,#60878,#60879),.UNSPECIFIED.,.F.,.F.,(4,1,1,1,1,1,
1,4),(65.9734457253864,66.5925482266013,67.5921229262213,68.5916976258413,
69.5912723254613,70.5908470250813,71.5904217247013,72.256631032566),
 .UNSPECIFIED.);
#2810=B_SPLINE_CURVE_WITH_KNOTS('',3,(#60880,#60881,#60882,#60883,#60884,
#60885,#60886,#60887,#60888,#60889),.UNSPECIFIED.,.F.,.F.,(4,1,1,1,1,1,
1,4),(65.9734457253866,66.2773687322691,67.2769434318891,68.2765181315091,
69.2760928311291,70.2756675307491,71.2752422303691,72.2566310325662),
 .UNSPECIFIED.);
#2811=B_SPLINE_CURVE_WITH_KNOTS('',3,(#60894,#60895,#60896,#60897,#60898,
#60899,#60900,#60901,#60902,#60903),.UNSPECIFIED.,.F.,.F.,(4,1,1,1,1,1,
1,4),(59.6902604182068,60.5951000288813,61.5946747285013,62.5942494281213,
63.5938241277413,64.5933988273613,65.5929735269813,65.9734457253864),
 .UNSPECIFIED.);
#2812=B_SPLINE_CURVE_WITH_KNOTS('',3,(#60904,#60905,#60906,#60907,#60908,
#60909,#60910,#60911,#60912,#60913),.UNSPECIFIED.,.F.,.F.,(4,1,1,1,1,1,
1,4),(59.690260418207,60.2799205345491,61.2794952341691,62.2790699337891,
63.2786446334091,64.2782193330291,65.2777940326491,65.9734457253866),
 .UNSPECIFIED.);
#2813=B_SPLINE_CURVE_WITH_KNOTS('',3,(#60918,#60919,#60920,#60921,#60922,
#60923,#60924,#60925,#60926,#60927,#60928),.UNSPECIFIED.,.F.,.F.,(4,1,1,
1,1,1,1,1,4),(53.4070751110272,53.5980771315413,54.5976518311613,55.5972265307813,
56.5968012304013,57.5963759300213,58.5959506296413,59.5955253292613,59.6902604182068),
 .UNSPECIFIED.);
#2814=B_SPLINE_CURVE_WITH_KNOTS('',3,(#60929,#60930,#60931,#60932,#60933,
#60934,#60935,#60936,#60937,#60938),.UNSPECIFIED.,.F.,.F.,(4,1,1,1,1,1,
1,4),(53.4070751110274,54.2824723368291,55.2820470364491,56.2816217360691,
57.2811964356891,58.2807711353091,59.2803458349291,59.690260418207),
 .UNSPECIFIED.);
#2815=B_SPLINE_CURVE_WITH_KNOTS('',3,(#60943,#60944,#60945,#60946,#60947,
#60948,#60949,#60950,#60951,#60952),.UNSPECIFIED.,.F.,.F.,(4,1,1,1,1,1,
1,4),(47.1238898038476,47.6006289338214,48.6002036334414,49.5997783330614,
50.5993530326813,51.5989277323013,52.5985024319213,53.4070751110272),
 .UNSPECIFIED.);
#2816=B_SPLINE_CURVE_WITH_KNOTS('',3,(#60953,#60954,#60955,#60956,#60957,
#60958,#60959,#60960,#60961,#60962,#60963),.UNSPECIFIED.,.F.,.F.,(4,1,1,
1,1,1,1,1,4),(47.1238898038478,47.2854494394891,48.2850241391091,49.2845988387291,
50.2841735383491,51.2837482379691,52.2833229375891,53.2828976372091,53.4070751110274),
 .UNSPECIFIED.);
#2817=B_SPLINE_CURVE_WITH_KNOTS('',3,(#60968,#60969,#60970,#60971,#60972,
#60973,#60974,#60975,#60976,#60977),.UNSPECIFIED.,.F.,.F.,(4,1,1,1,1,1,
1,4),(40.840704496668,41.6031807361014,42.6027554357214,43.6023301353414,
44.6019048349614,45.6014795345814,46.6010542342014,47.1238898038476),
 .UNSPECIFIED.);
#2818=B_SPLINE_CURVE_WITH_KNOTS('',3,(#60978,#60979,#60980,#60981,#60982,
#60983,#60984,#60985,#60986,#60987),.UNSPECIFIED.,.F.,.F.,(4,1,1,1,1,1,
1,4),(40.8407044966683,41.2880012417691,42.2875759413891,43.2871506410091,
44.2867253406291,45.2863000402491,46.2858747398691,47.1238898038478),
 .UNSPECIFIED.);
#2819=B_SPLINE_CURVE_WITH_KNOTS('',3,(#60992,#60993,#60994,#60995,#60996,
#60997,#60998,#60999,#61000,#61001,#61002),.UNSPECIFIED.,.F.,.F.,(4,1,1,
1,1,1,1,1,4),(34.5575191894884,34.6061578387614,35.6057325383814,36.6053072380014,
37.6048819376214,38.6044566372414,39.6040313368614,40.6036060364814,40.840704496668),
 .UNSPECIFIED.);
#2820=B_SPLINE_CURVE_WITH_KNOTS('',3,(#61003,#61004,#61005,#61006,#61007,
#61008,#61009,#61010,#61011,#61012),.UNSPECIFIED.,.F.,.F.,(4,1,1,1,1,1,
1,4),(34.5575191894887,35.2905530440491,36.2901277436691,37.2897024432891,
38.2892771429091,39.2888518425291,40.2884265421491,40.8407044966683),
 .UNSPECIFIED.);
#2821=B_SPLINE_CURVE_WITH_KNOTS('',3,(#61017,#61018,#61019,#61020,#61021,
#61022,#61023,#61024,#61025,#61026),.UNSPECIFIED.,.F.,.F.,(4,1,1,1,1,1,
1,4),(28.2743338823088,28.6087096410414,29.6082843406614,30.6078590402814,
31.6074337399014,32.6070084395214,33.6065831391414,34.5575191894884),
 .UNSPECIFIED.);
#2822=B_SPLINE_CURVE_WITH_KNOTS('',3,(#61027,#61028,#61029,#61030,#61031,
#61032,#61033,#61034,#61035,#61036,#61037),.UNSPECIFIED.,.F.,.F.,(4,1,1,
1,1,1,1,1,4),(28.2743338823091,28.2935301467091,29.2931048463291,30.2926795459491,
31.2922542455691,32.2918289451891,33.2914036448091,34.2909783444291,34.5575191894887),
 .UNSPECIFIED.);
#2823=B_SPLINE_CURVE_WITH_KNOTS('',3,(#61042,#61043,#61044,#61045,#61046,
#61047,#61048,#61049,#61050,#61051),.UNSPECIFIED.,.F.,.F.,(4,1,1,1,1,1,
1,4),(21.9911485751293,22.6112614433214,23.6108361429414,24.6104108425614,
25.6099855421814,26.6095602418014,27.6091349414214,28.2743338823088),
 .UNSPECIFIED.);
#2824=B_SPLINE_CURVE_WITH_KNOTS('',3,(#61052,#61053,#61054,#61055,#61056,
#61057,#61058,#61059,#61060,#61061),.UNSPECIFIED.,.F.,.F.,(4,1,1,1,1,1,
1,4),(21.9911485751295,22.2960819489891,23.2956566486091,24.2952313482291,
25.2948060478491,26.2943807474691,27.2939554470891,28.2743338823091),
 .UNSPECIFIED.);
#2825=B_SPLINE_CURVE_WITH_KNOTS('',3,(#61066,#61067,#61068,#61069,#61070,
#61071,#61072,#61073,#61074,#61075),.UNSPECIFIED.,.F.,.F.,(4,1,1,1,1,1,
1,4),(15.7079632679497,16.6138132456014,17.6133879452214,18.6129626448414,
19.6125373444614,20.6121120440814,21.6116867437014,21.9911485751293),
 .UNSPECIFIED.);
#2826=B_SPLINE_CURVE_WITH_KNOTS('',3,(#61076,#61077,#61078,#61079,#61080,
#61081,#61082,#61083,#61084,#61085),.UNSPECIFIED.,.F.,.F.,(4,1,1,1,1,1,
1,4),(15.7079632679499,16.2986337512691,17.2982084508891,18.2977831505091,
19.2973578501291,20.2969325497491,21.2965072493691,21.9911485751295),
 .UNSPECIFIED.);
#2827=B_SPLINE_CURVE_WITH_KNOTS('',3,(#61088,#61089,#61090,#61091,#61092,
#61093,#61094,#61095,#61096,#61097,#61098,#61099,#61100,#61101,#61102,#61103,
#61104,#61105,#61106,#61107,#61108,#61109,#61110,#61111,#61112,#61113,#61114,
#61115,#61116,#61117,#61118,#61119,#61120,#61121,#61122,#61123,#61124,#61125,
#61126,#61127,#61128,#61129,#61130,#61131,#61132,#61133,#61134,#61135,#61136,
#61137,#61138,#61139,#61140,#61141,#61142,#61143,#61144,#61145,#61146,#61147,
#61148,#61149,#61150,#61151,#61152,#61153,#61154,#61155,#61156,#61157,#61158,
#61159,#61160,#61161,#61162,#61163,#61164,#61165,#61166,#61167,#61168,#61169,
#61170,#61171,#61172),.UNSPECIFIED.,.F.,.F.,(4,3,3,3,3,3,3,3,3,3,3,3,3,
3,3,3,3,3,3,3,3,3,3,3,3,3,3,3,4),(-0.276631791712738,-0.26777280382095,
-0.253162595967305,-0.247575468035802,-0.244113223126194,-0.228893324436004,
-0.217867136109351,-0.213228637626788,-0.209216864955607,-0.193459635982162,
-0.177407427195511,-0.168226524852329,-0.162410876603139,-0.159528053086101,
-0.143000073191966,-0.140683817822782,-0.124741429572464,-0.116250765378535,
-0.111155360582251,-0.107652961500464,-0.0910939615488431,-0.0741766492334206,
-0.0647050431380984,-0.0582172002991486,-0.0537828459296116,-0.0363196889473096,
-0.0181598444736548,-0.00111710893352747,0.),.UNSPECIFIED.);
#2828=B_SPLINE_CURVE_WITH_KNOTS('',3,(#61177,#61178,#61179,#61180,#61181,
#61182,#61183,#61184,#61185,#61186,#61187,#61188,#61189,#61190,#61191,#61192,
#61193,#61194,#61195,#61196,#61197,#61198,#61199,#61200,#61201,#61202,#61203,
#61204,#61205,#61206,#61207,#61208,#61209,#61210,#61211,#61212,#61213,#61214,
#61215,#61216,#61217,#61218,#61219,#61220,#61221,#61222,#61223,#61224,#61225,
#61226,#61227,#61228,#61229,#61230,#61231,#61232,#61233,#61234,#61235,#61236,
#61237,#61238,#61239,#61240,#61241,#61242,#61243,#61244,#61245,#61246,#61247,
#61248,#61249,#61250,#61251,#61252,#61253,#61254,#61255,#61256,#61257,#61258),
 .UNSPECIFIED.,.F.,.F.,(4,3,3,3,3,3,3,3,3,3,3,3,3,3,3,3,3,3,3,3,3,3,3,3,
3,3,3,4),(-0.275362278356834,-0.264551439176698,-0.247185256457859,-0.238155454944618,
-0.234297382099102,-0.21709561190626,-0.205661407596225,-0.200946096586765,
-0.196794724908398,-0.180042528899867,-0.163712523477344,-0.154189886964504,
-0.148003615780328,-0.144168982533267,-0.128317505169721,-0.125621977425983,
-0.109669333874548,-0.101986130473596,-0.0960165185644219,-0.093169255793087,
-0.0774033899336095,-0.0617050632725603,-0.0534800915089582,-0.0478612930675681,
-0.0448398831927098,-0.0297305382808535,-0.0148652691404268,0.),
 .UNSPECIFIED.);
#2829=B_SPLINE_CURVE_WITH_KNOTS('',3,(#63011,#63012,#63013,#63014,#63015,
#63016,#63017,#63018,#63019,#63020,#63021,#63022,#63023,#63024,#63025,#63026),
 .UNSPECIFIED.,.F.,.F.,(4,3,3,3,3,4),(428.379342694673,428.81754613698,
429.8171208366,430.81669553622,431.81627023584,432.74182166138),
 .UNSPECIFIED.);
#2830=B_SPLINE_CURVE_WITH_KNOTS('',3,(#63028,#63029,#63030,#63031,#63032,
#63033,#63034,#63035,#63036,#63037,#63038,#63039,#63040,#63041,#63042,#63043,
#63044,#63045,#63046,#63047,#63048,#63049,#63050,#63051,#63052,#63053,#63054,
#63055,#63056,#63057,#63058,#63059,#63060,#63061,#63062,#63063,#63064,#63065,
#63066,#63067,#63068,#63069,#63070,#63071,#63072,#63073,#63074,#63075,#63076,
#63077,#63078,#63079,#63080,#63081,#63082,#63083,#63084,#63085,#63086,#63087,
#63088,#63089,#63090,#63091,#63092,#63093,#63094,#63095,#63096,#63097,#63098,
#63099,#63100,#63101,#63102,#63103,#63104,#63105,#63106,#63107,#63108,#63109,
#63110,#63111,#63112),.UNSPECIFIED.,.F.,.F.,(4,3,3,3,3,3,3,3,3,3,3,3,3,
3,3,3,3,3,3,3,3,3,3,3,3,3,3,3,4),(-0.276631791712687,-0.267772803820864,
-0.253162597214951,-0.24757547093428,-0.244113224588513,-0.228893326817863,
-0.217867138193469,-0.213228641517051,-0.209216865648389,-0.19345963730386,
-0.177407428450592,-0.168226525793622,-0.162410877946272,-0.159528054577906,
-0.143000074615614,-0.140683817822713,-0.124741430017734,-0.116250765733781,
-0.111155360560927,-0.107652961444369,-0.0910939620347423,-0.0741766502224574,
-0.0647050432131039,-0.0582172004360556,-0.0537828456880876,-0.0363196890394545,
-0.0181598445197272,-0.00111710732716392,0.),.UNSPECIFIED.);
#2831=B_SPLINE_CURVE_WITH_KNOTS('',3,(#63113,#63114,#63115,#63116,#63117,
#63118,#63119,#63120,#63121),.UNSPECIFIED.,.F.,.F.,(4,1,1,1,1,1,4),(10.3752088276291,
11.3007602531692,12.3003349527892,13.2999096524091,14.2994843520291,15.2990590516491,
15.7079632679499),.UNSPECIFIED.);
#2832=B_SPLINE_CURVE_WITH_KNOTS('',3,(#63127,#63128,#63129,#63130,#63131,
#63132,#63133,#63134,#63135,#63136,#63137,#63138,#63139,#63140,#63141,#63142,
#63143,#63144,#63145,#63146,#63147,#63148,#63149,#63150,#63151,#63152,#63153,
#63154,#63155,#63156,#63157,#63158,#63159,#63160,#63161,#63162,#63163,#63164,
#63165,#63166,#63167,#63168,#63169,#63170,#63171,#63172,#63173,#63174,#63175,
#63176,#63177,#63178,#63179,#63180,#63181,#63182,#63183,#63184,#63185,#63186,
#63187,#63188,#63189,#63190,#63191,#63192,#63193,#63194,#63195,#63196,#63197,
#63198,#63199,#63200,#63201,#63202,#63203,#63204,#63205,#63206,#63207,#63208),
 .UNSPECIFIED.,.F.,.F.,(4,3,3,3,3,3,3,3,3,3,3,3,3,3,3,3,3,3,3,3,3,3,3,3,
3,3,3,4),(-0.275362278356922,-0.264551439176764,-0.247185256457921,-0.238155454613246,
-0.234297381972466,-0.217095611759951,-0.20566140746821,-0.200946095991088,
-0.196794724755822,-0.180042528611185,-0.163712522131083,-0.154189885954817,
-0.148003612972641,-0.144168982208487,-0.128317503830928,-0.12562197742602,
-0.109669343900505,-0.101986144157958,-0.0960166186373187,-0.0931694064854494,
-0.0774035414773043,-0.0617052132751136,-0.0534801524126021,-0.0478615116658561,
-0.0448398640447273,-0.0297305204847559,-0.0148652602423779,0.),
 .UNSPECIFIED.);
#2833=B_SPLINE_CURVE_WITH_KNOTS('',3,(#63211,#63212,#63213,#63214,#63215,
#63216,#63217,#63218),.UNSPECIFIED.,.F.,.F.,(4,1,1,1,1,4),(11.6159397475014,
12.6155144471214,13.6150891467414,14.6146638463614,15.6142385459814,15.7079632679497),
 .UNSPECIFIED.);
#2834=B_SPLINE_CURVE_WITH_KNOTS('',3,(#64971,#64972,#64973,#64974,#64975,
#64976,#64977,#64978,#64979,#64980,#64981,#64982,#64983),.UNSPECIFIED.,
 .F.,.F.,(4,3,3,3,4),(-434.814994334699,-433.815419635079,-432.815844935459,
-431.816270235839,-431.348624408659),.UNSPECIFIED.);
#3526=FACE_BOUND('',#6788,.T.);
#3527=FACE_BOUND('',#6941,.T.);
#3528=FACE_BOUND('',#6945,.T.);
#3529=FACE_BOUND('',#6946,.T.);
#3530=FACE_BOUND('',#6947,.T.);
#3531=FACE_BOUND('',#6948,.T.);
#3532=FACE_BOUND('',#6949,.T.);
#3533=FACE_BOUND('',#6950,.T.);
#3534=FACE_BOUND('',#6951,.T.);
#3535=FACE_BOUND('',#6952,.T.);
#3536=FACE_BOUND('',#6953,.T.);
#3537=FACE_BOUND('',#6954,.T.);
#3538=FACE_BOUND('',#6955,.T.);
#3539=FACE_BOUND('',#6956,.T.);
#3540=FACE_BOUND('',#6957,.T.);
#3541=FACE_BOUND('',#6958,.T.);
#3542=FACE_BOUND('',#6959,.T.);
#3543=FACE_BOUND('',#6960,.T.);
#3544=FACE_BOUND('',#6961,.T.);
#3545=FACE_BOUND('',#6962,.T.);
#3546=FACE_BOUND('',#6963,.T.);
#3547=FACE_BOUND('',#6964,.T.);
#3548=FACE_BOUND('',#6965,.T.);
#3549=FACE_BOUND('',#6966,.T.);
#3550=FACE_BOUND('',#6967,.T.);
#3551=FACE_BOUND('',#6968,.T.);
#3552=FACE_BOUND('',#6969,.T.);
#3553=FACE_BOUND('',#6970,.T.);
#3554=FACE_BOUND('',#6971,.T.);
#3555=FACE_BOUND('',#6972,.T.);
#3556=FACE_BOUND('',#6973,.T.);
#3557=FACE_BOUND('',#6974,.T.);
#3558=FACE_BOUND('',#6975,.T.);
#3559=FACE_BOUND('',#6976,.T.);
#3560=FACE_BOUND('',#6977,.T.);
#3561=FACE_BOUND('',#6978,.T.);
#3562=FACE_BOUND('',#6979,.T.);
#3563=FACE_BOUND('',#6982,.T.);
#4644=FACE_OUTER_BOUND('',#6642,.T.);
#4645=FACE_OUTER_BOUND('',#6643,.T.);
#4646=FACE_OUTER_BOUND('',#6644,.T.);
#4647=FACE_OUTER_BOUND('',#6645,.T.);
#4648=FACE_OUTER_BOUND('',#6646,.T.);
#4649=FACE_OUTER_BOUND('',#6647,.T.);
#4650=FACE_OUTER_BOUND('',#6648,.T.);
#4651=FACE_OUTER_BOUND('',#6649,.T.);
#4652=FACE_OUTER_BOUND('',#6650,.T.);
#4653=FACE_OUTER_BOUND('',#6651,.T.);
#4654=FACE_OUTER_BOUND('',#6652,.T.);
#4655=FACE_OUTER_BOUND('',#6653,.T.);
#4656=FACE_OUTER_BOUND('',#6654,.T.);
#4657=FACE_OUTER_BOUND('',#6655,.T.);
#4658=FACE_OUTER_BOUND('',#6656,.T.);
#4659=FACE_OUTER_BOUND('',#6657,.T.);
#4660=FACE_OUTER_BOUND('',#6658,.T.);
#4661=FACE_OUTER_BOUND('',#6659,.T.);
#4662=FACE_OUTER_BOUND('',#6660,.T.);
#4663=FACE_OUTER_BOUND('',#6661,.T.);
#4664=FACE_OUTER_BOUND('',#6662,.T.);
#4665=FACE_OUTER_BOUND('',#6663,.T.);
#4666=FACE_OUTER_BOUND('',#6664,.T.);
#4667=FACE_OUTER_BOUND('',#6665,.T.);
#4668=FACE_OUTER_BOUND('',#6666,.T.);
#4669=FACE_OUTER_BOUND('',#6667,.T.);
#4670=FACE_OUTER_BOUND('',#6668,.T.);
#4671=FACE_OUTER_BOUND('',#6669,.T.);
#4672=FACE_OUTER_BOUND('',#6670,.T.);
#4673=FACE_OUTER_BOUND('',#6671,.T.);
#4674=FACE_OUTER_BOUND('',#6672,.T.);
#4675=FACE_OUTER_BOUND('',#6673,.T.);
#4676=FACE_OUTER_BOUND('',#6674,.T.);
#4677=FACE_OUTER_BOUND('',#6675,.T.);
#4678=FACE_OUTER_BOUND('',#6676,.T.);
#4679=FACE_OUTER_BOUND('',#6677,.T.);
#4680=FACE_OUTER_BOUND('',#6678,.T.);
#4681=FACE_OUTER_BOUND('',#6679,.T.);
#4682=FACE_OUTER_BOUND('',#6680,.T.);
#4683=FACE_OUTER_BOUND('',#6681,.T.);
#4684=FACE_OUTER_BOUND('',#6682,.T.);
#4685=FACE_OUTER_BOUND('',#6683,.T.);
#4686=FACE_OUTER_BOUND('',#6684,.T.);
#4687=FACE_OUTER_BOUND('',#6685,.T.);
#4688=FACE_OUTER_BOUND('',#6686,.T.);
#4689=FACE_OUTER_BOUND('',#6687,.T.);
#4690=FACE_OUTER_BOUND('',#6688,.T.);
#4691=FACE_OUTER_BOUND('',#6689,.T.);
#4692=FACE_OUTER_BOUND('',#6690,.T.);
#4693=FACE_OUTER_BOUND('',#6691,.T.);
#4694=FACE_OUTER_BOUND('',#6692,.T.);
#4695=FACE_OUTER_BOUND('',#6693,.T.);
#4696=FACE_OUTER_BOUND('',#6694,.T.);
#4697=FACE_OUTER_BOUND('',#6695,.T.);
#4698=FACE_OUTER_BOUND('',#6696,.T.);
#4699=FACE_OUTER_BOUND('',#6697,.T.);
#4700=FACE_OUTER_BOUND('',#6698,.T.);
#4701=FACE_OUTER_BOUND('',#6699,.T.);
#4702=FACE_OUTER_BOUND('',#6700,.T.);
#4703=FACE_OUTER_BOUND('',#6701,.T.);
#4704=FACE_OUTER_BOUND('',#6702,.T.);
#4705=FACE_OUTER_BOUND('',#6703,.T.);
#4706=FACE_OUTER_BOUND('',#6704,.T.);
#4707=FACE_OUTER_BOUND('',#6705,.T.);
#4708=FACE_OUTER_BOUND('',#6706,.T.);
#4709=FACE_OUTER_BOUND('',#6707,.T.);
#4710=FACE_OUTER_BOUND('',#6708,.T.);
#4711=FACE_OUTER_BOUND('',#6709,.T.);
#4712=FACE_OUTER_BOUND('',#6710,.T.);
#4713=FACE_OUTER_BOUND('',#6711,.T.);
#4714=FACE_OUTER_BOUND('',#6712,.T.);
#4715=FACE_OUTER_BOUND('',#6713,.T.);
#4716=FACE_OUTER_BOUND('',#6714,.T.);
#4717=FACE_OUTER_BOUND('',#6715,.T.);
#4718=FACE_OUTER_BOUND('',#6716,.T.);
#4719=FACE_OUTER_BOUND('',#6717,.T.);
#4720=FACE_OUTER_BOUND('',#6718,.T.);
#4721=FACE_OUTER_BOUND('',#6719,.T.);
#4722=FACE_OUTER_BOUND('',#6720,.T.);
#4723=FACE_OUTER_BOUND('',#6721,.T.);
#4724=FACE_OUTER_BOUND('',#6722,.T.);
#4725=FACE_OUTER_BOUND('',#6723,.T.);
#4726=FACE_OUTER_BOUND('',#6724,.T.);
#4727=FACE_OUTER_BOUND('',#6725,.T.);
#4728=FACE_OUTER_BOUND('',#6726,.T.);
#4729=FACE_OUTER_BOUND('',#6727,.T.);
#4730=FACE_OUTER_BOUND('',#6728,.T.);
#4731=FACE_OUTER_BOUND('',#6729,.T.);
#4732=FACE_OUTER_BOUND('',#6730,.T.);
#4733=FACE_OUTER_BOUND('',#6731,.T.);
#4734=FACE_OUTER_BOUND('',#6732,.T.);
#4735=FACE_OUTER_BOUND('',#6733,.T.);
#4736=FACE_OUTER_BOUND('',#6734,.T.);
#4737=FACE_OUTER_BOUND('',#6735,.T.);
#4738=FACE_OUTER_BOUND('',#6736,.T.);
#4739=FACE_OUTER_BOUND('',#6737,.T.);
#4740=FACE_OUTER_BOUND('',#6738,.T.);
#4741=FACE_OUTER_BOUND('',#6739,.T.);
#4742=FACE_OUTER_BOUND('',#6740,.T.);
#4743=FACE_OUTER_BOUND('',#6741,.T.);
#4744=FACE_OUTER_BOUND('',#6742,.T.);
#4745=FACE_OUTER_BOUND('',#6743,.T.);
#4746=FACE_OUTER_BOUND('',#6744,.T.);
#4747=FACE_OUTER_BOUND('',#6745,.T.);
#4748=FACE_OUTER_BOUND('',#6746,.T.);
#4749=FACE_OUTER_BOUND('',#6747,.T.);
#4750=FACE_OUTER_BOUND('',#6748,.T.);
#4751=FACE_OUTER_BOUND('',#6749,.T.);
#4752=FACE_OUTER_BOUND('',#6750,.T.);
#4753=FACE_OUTER_BOUND('',#6751,.T.);
#4754=FACE_OUTER_BOUND('',#6752,.T.);
#4755=FACE_OUTER_BOUND('',#6753,.T.);
#4756=FACE_OUTER_BOUND('',#6754,.T.);
#4757=FACE_OUTER_BOUND('',#6755,.T.);
#4758=FACE_OUTER_BOUND('',#6756,.T.);
#4759=FACE_OUTER_BOUND('',#6757,.T.);
#4760=FACE_OUTER_BOUND('',#6758,.T.);
#4761=FACE_OUTER_BOUND('',#6759,.T.);
#4762=FACE_OUTER_BOUND('',#6760,.T.);
#4763=FACE_OUTER_BOUND('',#6761,.T.);
#4764=FACE_OUTER_BOUND('',#6762,.T.);
#4765=FACE_OUTER_BOUND('',#6763,.T.);
#4766=FACE_OUTER_BOUND('',#6764,.T.);
#4767=FACE_OUTER_BOUND('',#6765,.T.);
#4768=FACE_OUTER_BOUND('',#6766,.T.);
#4769=FACE_OUTER_BOUND('',#6767,.T.);
#4770=FACE_OUTER_BOUND('',#6768,.T.);
#4771=FACE_OUTER_BOUND('',#6769,.T.);
#4772=FACE_OUTER_BOUND('',#6770,.T.);
#4773=FACE_OUTER_BOUND('',#6771,.T.);
#4774=FACE_OUTER_BOUND('',#6772,.T.);
#4775=FACE_OUTER_BOUND('',#6773,.T.);
#4776=FACE_OUTER_BOUND('',#6774,.T.);
#4777=FACE_OUTER_BOUND('',#6775,.T.);
#4778=FACE_OUTER_BOUND('',#6776,.T.);
#4779=FACE_OUTER_BOUND('',#6777,.T.);
#4780=FACE_OUTER_BOUND('',#6778,.T.);
#4781=FACE_OUTER_BOUND('',#6779,.T.);
#4782=FACE_OUTER_BOUND('',#6780,.T.);
#4783=FACE_OUTER_BOUND('',#6781,.T.);
#4784=FACE_OUTER_BOUND('',#6782,.T.);
#4785=FACE_OUTER_BOUND('',#6783,.T.);
#4786=FACE_OUTER_BOUND('',#6784,.T.);
#4787=FACE_OUTER_BOUND('',#6785,.T.);
#4788=FACE_OUTER_BOUND('',#6786,.T.);
#4789=FACE_OUTER_BOUND('',#6787,.T.);
#4790=FACE_OUTER_BOUND('',#6789,.T.);
#4791=FACE_OUTER_BOUND('',#6790,.T.);
#4792=FACE_OUTER_BOUND('',#6791,.T.);
#4793=FACE_OUTER_BOUND('',#6792,.T.);
#4794=FACE_OUTER_BOUND('',#6793,.T.);
#4795=FACE_OUTER_BOUND('',#6794,.T.);
#4796=FACE_OUTER_BOUND('',#6795,.T.);
#4797=FACE_OUTER_BOUND('',#6796,.T.);
#4798=FACE_OUTER_BOUND('',#6797,.T.);
#4799=FACE_OUTER_BOUND('',#6798,.T.);
#4800=FACE_OUTER_BOUND('',#6799,.T.);
#4801=FACE_OUTER_BOUND('',#6800,.T.);
#4802=FACE_OUTER_BOUND('',#6801,.T.);
#4803=FACE_OUTER_BOUND('',#6802,.T.);
#4804=FACE_OUTER_BOUND('',#6803,.T.);
#4805=FACE_OUTER_BOUND('',#6804,.T.);
#4806=FACE_OUTER_BOUND('',#6805,.T.);
#4807=FACE_OUTER_BOUND('',#6806,.T.);
#4808=FACE_OUTER_BOUND('',#6807,.T.);
#4809=FACE_OUTER_BOUND('',#6808,.T.);
#4810=FACE_OUTER_BOUND('',#6809,.T.);
#4811=FACE_OUTER_BOUND('',#6810,.T.);
#4812=FACE_OUTER_BOUND('',#6811,.T.);
#4813=FACE_OUTER_BOUND('',#6812,.T.);
#4814=FACE_OUTER_BOUND('',#6813,.T.);
#4815=FACE_OUTER_BOUND('',#6814,.T.);
#4816=FACE_OUTER_BOUND('',#6815,.T.);
#4817=FACE_OUTER_BOUND('',#6816,.T.);
#4818=FACE_OUTER_BOUND('',#6817,.T.);
#4819=FACE_OUTER_BOUND('',#6818,.T.);
#4820=FACE_OUTER_BOUND('',#6819,.T.);
#4821=FACE_OUTER_BOUND('',#6820,.T.);
#4822=FACE_OUTER_BOUND('',#6821,.T.);
#4823=FACE_OUTER_BOUND('',#6822,.T.);
#4824=FACE_OUTER_BOUND('',#6823,.T.);
#4825=FACE_OUTER_BOUND('',#6824,.T.);
#4826=FACE_OUTER_BOUND('',#6825,.T.);
#4827=FACE_OUTER_BOUND('',#6826,.T.);
#4828=FACE_OUTER_BOUND('',#6827,.T.);
#4829=FACE_OUTER_BOUND('',#6828,.T.);
#4830=FACE_OUTER_BOUND('',#6829,.T.);
#4831=FACE_OUTER_BOUND('',#6830,.T.);
#4832=FACE_OUTER_BOUND('',#6831,.T.);
#4833=FACE_OUTER_BOUND('',#6832,.T.);
#4834=FACE_OUTER_BOUND('',#6833,.T.);
#4835=FACE_OUTER_BOUND('',#6834,.T.);
#4836=FACE_OUTER_BOUND('',#6835,.T.);
#4837=FACE_OUTER_BOUND('',#6836,.T.);
#4838=FACE_OUTER_BOUND('',#6837,.T.);
#4839=FACE_OUTER_BOUND('',#6838,.T.);
#4840=FACE_OUTER_BOUND('',#6839,.T.);
#4841=FACE_OUTER_BOUND('',#6840,.T.);
#4842=FACE_OUTER_BOUND('',#6841,.T.);
#4843=FACE_OUTER_BOUND('',#6842,.T.);
#4844=FACE_OUTER_BOUND('',#6843,.T.);
#4845=FACE_OUTER_BOUND('',#6844,.T.);
#4846=FACE_OUTER_BOUND('',#6845,.T.);
#4847=FACE_OUTER_BOUND('',#6846,.T.);
#4848=FACE_OUTER_BOUND('',#6847,.T.);
#4849=FACE_OUTER_BOUND('',#6848,.T.);
#4850=FACE_OUTER_BOUND('',#6849,.T.);
#4851=FACE_OUTER_BOUND('',#6850,.T.);
#4852=FACE_OUTER_BOUND('',#6851,.T.);
#4853=FACE_OUTER_BOUND('',#6852,.T.);
#4854=FACE_OUTER_BOUND('',#6853,.T.);
#4855=FACE_OUTER_BOUND('',#6854,.T.);
#4856=FACE_OUTER_BOUND('',#6855,.T.);
#4857=FACE_OUTER_BOUND('',#6856,.T.);
#4858=FACE_OUTER_BOUND('',#6857,.T.);
#4859=FACE_OUTER_BOUND('',#6858,.T.);
#4860=FACE_OUTER_BOUND('',#6859,.T.);
#4861=FACE_OUTER_BOUND('',#6860,.T.);
#4862=FACE_OUTER_BOUND('',#6861,.T.);
#4863=FACE_OUTER_BOUND('',#6862,.T.);
#4864=FACE_OUTER_BOUND('',#6863,.T.);
#4865=FACE_OUTER_BOUND('',#6864,.T.);
#4866=FACE_OUTER_BOUND('',#6865,.T.);
#4867=FACE_OUTER_BOUND('',#6866,.T.);
#4868=FACE_OUTER_BOUND('',#6867,.T.);
#4869=FACE_OUTER_BOUND('',#6868,.T.);
#4870=FACE_OUTER_BOUND('',#6869,.T.);
#4871=FACE_OUTER_BOUND('',#6870,.T.);
#4872=FACE_OUTER_BOUND('',#6871,.T.);
#4873=FACE_OUTER_BOUND('',#6872,.T.);
#4874=FACE_OUTER_BOUND('',#6873,.T.);
#4875=FACE_OUTER_BOUND('',#6874,.T.);
#4876=FACE_OUTER_BOUND('',#6875,.T.);
#4877=FACE_OUTER_BOUND('',#6876,.T.);
#4878=FACE_OUTER_BOUND('',#6877,.T.);
#4879=FACE_OUTER_BOUND('',#6878,.T.);
#4880=FACE_OUTER_BOUND('',#6879,.T.);
#4881=FACE_OUTER_BOUND('',#6880,.T.);
#4882=FACE_OUTER_BOUND('',#6881,.T.);
#4883=FACE_OUTER_BOUND('',#6882,.T.);
#4884=FACE_OUTER_BOUND('',#6883,.T.);
#4885=FACE_OUTER_BOUND('',#6884,.T.);
#4886=FACE_OUTER_BOUND('',#6885,.T.);
#4887=FACE_OUTER_BOUND('',#6886,.T.);
#4888=FACE_OUTER_BOUND('',#6887,.T.);
#4889=FACE_OUTER_BOUND('',#6888,.T.);
#4890=FACE_OUTER_BOUND('',#6889,.T.);
#4891=FACE_OUTER_BOUND('',#6890,.T.);
#4892=FACE_OUTER_BOUND('',#6891,.T.);
#4893=FACE_OUTER_BOUND('',#6892,.T.);
#4894=FACE_OUTER_BOUND('',#6893,.T.);
#4895=FACE_OUTER_BOUND('',#6894,.T.);
#4896=FACE_OUTER_BOUND('',#6895,.T.);
#4897=FACE_OUTER_BOUND('',#6896,.T.);
#4898=FACE_OUTER_BOUND('',#6897,.T.);
#4899=FACE_OUTER_BOUND('',#6898,.T.);
#4900=FACE_OUTER_BOUND('',#6899,.T.);
#4901=FACE_OUTER_BOUND('',#6900,.T.);
#4902=FACE_OUTER_BOUND('',#6901,.T.);
#4903=FACE_OUTER_BOUND('',#6902,.T.);
#4904=FACE_OUTER_BOUND('',#6903,.T.);
#4905=FACE_OUTER_BOUND('',#6904,.T.);
#4906=FACE_OUTER_BOUND('',#6905,.T.);
#4907=FACE_OUTER_BOUND('',#6906,.T.);
#4908=FACE_OUTER_BOUND('',#6907,.T.);
#4909=FACE_OUTER_BOUND('',#6908,.T.);
#4910=FACE_OUTER_BOUND('',#6909,.T.);
#4911=FACE_OUTER_BOUND('',#6910,.T.);
#4912=FACE_OUTER_BOUND('',#6911,.T.);
#4913=FACE_OUTER_BOUND('',#6912,.T.);
#4914=FACE_OUTER_BOUND('',#6913,.T.);
#4915=FACE_OUTER_BOUND('',#6914,.T.);
#4916=FACE_OUTER_BOUND('',#6915,.T.);
#4917=FACE_OUTER_BOUND('',#6916,.T.);
#4918=FACE_OUTER_BOUND('',#6917,.T.);
#4919=FACE_OUTER_BOUND('',#6918,.T.);
#4920=FACE_OUTER_BOUND('',#6919,.T.);
#4921=FACE_OUTER_BOUND('',#6920,.T.);
#4922=FACE_OUTER_BOUND('',#6921,.T.);
#4923=FACE_OUTER_BOUND('',#6922,.T.);
#4924=FACE_OUTER_BOUND('',#6923,.T.);
#4925=FACE_OUTER_BOUND('',#6924,.T.);
#4926=FACE_OUTER_BOUND('',#6925,.T.);
#4927=FACE_OUTER_BOUND('',#6926,.T.);
#4928=FACE_OUTER_BOUND('',#6927,.T.);
#4929=FACE_OUTER_BOUND('',#6928,.T.);
#4930=FACE_OUTER_BOUND('',#6929,.T.);
#4931=FACE_OUTER_BOUND('',#6930,.T.);
#4932=FACE_OUTER_BOUND('',#6931,.T.);
#4933=FACE_OUTER_BOUND('',#6932,.T.);
#4934=FACE_OUTER_BOUND('',#6933,.T.);
#4935=FACE_OUTER_BOUND('',#6934,.T.);
#4936=FACE_OUTER_BOUND('',#6935,.T.);
#4937=FACE_OUTER_BOUND('',#6936,.T.);
#4938=FACE_OUTER_BOUND('',#6937,.T.);
#4939=FACE_OUTER_BOUND('',#6938,.T.);
#4940=FACE_OUTER_BOUND('',#6939,.T.);
#4941=FACE_OUTER_BOUND('',#6940,.T.);
#4942=FACE_OUTER_BOUND('',#6942,.T.);
#4943=FACE_OUTER_BOUND('',#6943,.T.);
#4944=FACE_OUTER_BOUND('',#6944,.T.);
#4945=FACE_OUTER_BOUND('',#6980,.T.);
#4946=FACE_OUTER_BOUND('',#6981,.T.);
#6642=EDGE_LOOP('',(#24345,#24346,#24347,#24348));
#6643=EDGE_LOOP('',(#24349,#24350,#24351,#24352));
#6644=EDGE_LOOP('',(#24353,#24354,#24355,#24356));
#6645=EDGE_LOOP('',(#24357,#24358,#24359,#24360));
#6646=EDGE_LOOP('',(#24361,#24362,#24363,#24364));
#6647=EDGE_LOOP('',(#24365,#24366,#24367,#24368));
#6648=EDGE_LOOP('',(#24369,#24370,#24371,#24372));
#6649=EDGE_LOOP('',(#24373,#24374,#24375,#24376));
#6650=EDGE_LOOP('',(#24377,#24378,#24379,#24380));
#6651=EDGE_LOOP('',(#24381,#24382,#24383,#24384));
#6652=EDGE_LOOP('',(#24385,#24386,#24387,#24388));
#6653=EDGE_LOOP('',(#24389,#24390,#24391,#24392));
#6654=EDGE_LOOP('',(#24393,#24394,#24395,#24396));
#6655=EDGE_LOOP('',(#24397,#24398,#24399,#24400));
#6656=EDGE_LOOP('',(#24401,#24402,#24403,#24404));
#6657=EDGE_LOOP('',(#24405,#24406,#24407,#24408));
#6658=EDGE_LOOP('',(#24409,#24410,#24411,#24412));
#6659=EDGE_LOOP('',(#24413,#24414,#24415,#24416));
#6660=EDGE_LOOP('',(#24417,#24418,#24419,#24420));
#6661=EDGE_LOOP('',(#24421,#24422,#24423,#24424));
#6662=EDGE_LOOP('',(#24425,#24426,#24427,#24428));
#6663=EDGE_LOOP('',(#24429,#24430,#24431,#24432));
#6664=EDGE_LOOP('',(#24433,#24434,#24435,#24436));
#6665=EDGE_LOOP('',(#24437,#24438,#24439,#24440));
#6666=EDGE_LOOP('',(#24441,#24442,#24443,#24444));
#6667=EDGE_LOOP('',(#24445,#24446,#24447,#24448));
#6668=EDGE_LOOP('',(#24449,#24450,#24451,#24452));
#6669=EDGE_LOOP('',(#24453,#24454,#24455,#24456));
#6670=EDGE_LOOP('',(#24457,#24458,#24459,#24460));
#6671=EDGE_LOOP('',(#24461,#24462,#24463,#24464));
#6672=EDGE_LOOP('',(#24465,#24466,#24467,#24468));
#6673=EDGE_LOOP('',(#24469,#24470,#24471,#24472));
#6674=EDGE_LOOP('',(#24473,#24474,#24475,#24476));
#6675=EDGE_LOOP('',(#24477,#24478,#24479,#24480));
#6676=EDGE_LOOP('',(#24481,#24482,#24483,#24484));
#6677=EDGE_LOOP('',(#24485,#24486,#24487,#24488));
#6678=EDGE_LOOP('',(#24489,#24490,#24491,#24492));
#6679=EDGE_LOOP('',(#24493,#24494,#24495,#24496));
#6680=EDGE_LOOP('',(#24497,#24498,#24499,#24500));
#6681=EDGE_LOOP('',(#24501,#24502,#24503,#24504));
#6682=EDGE_LOOP('',(#24505,#24506,#24507,#24508));
#6683=EDGE_LOOP('',(#24509,#24510,#24511,#24512));
#6684=EDGE_LOOP('',(#24513,#24514,#24515,#24516));
#6685=EDGE_LOOP('',(#24517,#24518,#24519,#24520));
#6686=EDGE_LOOP('',(#24521,#24522,#24523,#24524));
#6687=EDGE_LOOP('',(#24525,#24526,#24527,#24528));
#6688=EDGE_LOOP('',(#24529,#24530,#24531,#24532));
#6689=EDGE_LOOP('',(#24533,#24534,#24535,#24536));
#6690=EDGE_LOOP('',(#24537,#24538,#24539,#24540));
#6691=EDGE_LOOP('',(#24541,#24542,#24543,#24544));
#6692=EDGE_LOOP('',(#24545,#24546,#24547,#24548));
#6693=EDGE_LOOP('',(#24549,#24550,#24551,#24552));
#6694=EDGE_LOOP('',(#24553,#24554,#24555,#24556));
#6695=EDGE_LOOP('',(#24557,#24558,#24559,#24560));
#6696=EDGE_LOOP('',(#24561,#24562,#24563,#24564));
#6697=EDGE_LOOP('',(#24565,#24566,#24567,#24568));
#6698=EDGE_LOOP('',(#24569,#24570,#24571,#24572));
#6699=EDGE_LOOP('',(#24573,#24574,#24575,#24576));
#6700=EDGE_LOOP('',(#24577,#24578,#24579,#24580));
#6701=EDGE_LOOP('',(#24581,#24582,#24583,#24584));
#6702=EDGE_LOOP('',(#24585,#24586,#24587,#24588));
#6703=EDGE_LOOP('',(#24589,#24590,#24591,#24592));
#6704=EDGE_LOOP('',(#24593,#24594,#24595,#24596));
#6705=EDGE_LOOP('',(#24597,#24598,#24599,#24600));
#6706=EDGE_LOOP('',(#24601,#24602,#24603,#24604));
#6707=EDGE_LOOP('',(#24605,#24606,#24607,#24608));
#6708=EDGE_LOOP('',(#24609,#24610,#24611,#24612));
#6709=EDGE_LOOP('',(#24613,#24614,#24615,#24616));
#6710=EDGE_LOOP('',(#24617,#24618,#24619,#24620));
#6711=EDGE_LOOP('',(#24621,#24622,#24623,#24624));
#6712=EDGE_LOOP('',(#24625,#24626,#24627,#24628));
#6713=EDGE_LOOP('',(#24629,#24630,#24631,#24632));
#6714=EDGE_LOOP('',(#24633,#24634,#24635,#24636));
#6715=EDGE_LOOP('',(#24637,#24638,#24639,#24640));
#6716=EDGE_LOOP('',(#24641,#24642,#24643,#24644));
#6717=EDGE_LOOP('',(#24645,#24646,#24647,#24648));
#6718=EDGE_LOOP('',(#24649,#24650,#24651,#24652));
#6719=EDGE_LOOP('',(#24653,#24654,#24655,#24656));
#6720=EDGE_LOOP('',(#24657,#24658,#24659,#24660));
#6721=EDGE_LOOP('',(#24661,#24662,#24663,#24664));
#6722=EDGE_LOOP('',(#24665,#24666,#24667,#24668));
#6723=EDGE_LOOP('',(#24669,#24670,#24671,#24672));
#6724=EDGE_LOOP('',(#24673,#24674,#24675,#24676));
#6725=EDGE_LOOP('',(#24677,#24678,#24679,#24680));
#6726=EDGE_LOOP('',(#24681,#24682,#24683,#24684));
#6727=EDGE_LOOP('',(#24685,#24686,#24687,#24688));
#6728=EDGE_LOOP('',(#24689,#24690,#24691,#24692));
#6729=EDGE_LOOP('',(#24693,#24694,#24695,#24696));
#6730=EDGE_LOOP('',(#24697,#24698,#24699,#24700));
#6731=EDGE_LOOP('',(#24701,#24702,#24703,#24704));
#6732=EDGE_LOOP('',(#24705,#24706,#24707,#24708));
#6733=EDGE_LOOP('',(#24709,#24710,#24711,#24712));
#6734=EDGE_LOOP('',(#24713,#24714,#24715,#24716));
#6735=EDGE_LOOP('',(#24717,#24718,#24719,#24720));
#6736=EDGE_LOOP('',(#24721,#24722,#24723,#24724));
#6737=EDGE_LOOP('',(#24725,#24726,#24727,#24728));
#6738=EDGE_LOOP('',(#24729,#24730,#24731,#24732));
#6739=EDGE_LOOP('',(#24733,#24734,#24735,#24736));
#6740=EDGE_LOOP('',(#24737,#24738,#24739,#24740));
#6741=EDGE_LOOP('',(#24741,#24742,#24743,#24744));
#6742=EDGE_LOOP('',(#24745,#24746,#24747,#24748));
#6743=EDGE_LOOP('',(#24749,#24750,#24751,#24752));
#6744=EDGE_LOOP('',(#24753,#24754,#24755,#24756));
#6745=EDGE_LOOP('',(#24757,#24758,#24759,#24760));
#6746=EDGE_LOOP('',(#24761,#24762,#24763,#24764));
#6747=EDGE_LOOP('',(#24765,#24766,#24767,#24768));
#6748=EDGE_LOOP('',(#24769,#24770,#24771,#24772));
#6749=EDGE_LOOP('',(#24773,#24774,#24775,#24776));
#6750=EDGE_LOOP('',(#24777,#24778,#24779,#24780));
#6751=EDGE_LOOP('',(#24781,#24782,#24783,#24784));
#6752=EDGE_LOOP('',(#24785,#24786,#24787,#24788));
#6753=EDGE_LOOP('',(#24789,#24790,#24791,#24792));
#6754=EDGE_LOOP('',(#24793,#24794,#24795,#24796));
#6755=EDGE_LOOP('',(#24797,#24798,#24799,#24800));
#6756=EDGE_LOOP('',(#24801,#24802,#24803,#24804));
#6757=EDGE_LOOP('',(#24805,#24806,#24807,#24808));
#6758=EDGE_LOOP('',(#24809,#24810,#24811,#24812));
#6759=EDGE_LOOP('',(#24813,#24814,#24815,#24816));
#6760=EDGE_LOOP('',(#24817,#24818,#24819,#24820));
#6761=EDGE_LOOP('',(#24821,#24822,#24823,#24824));
#6762=EDGE_LOOP('',(#24825,#24826,#24827,#24828));
#6763=EDGE_LOOP('',(#24829,#24830,#24831,#24832));
#6764=EDGE_LOOP('',(#24833,#24834,#24835,#24836));
#6765=EDGE_LOOP('',(#24837,#24838,#24839,#24840));
#6766=EDGE_LOOP('',(#24841,#24842,#24843,#24844));
#6767=EDGE_LOOP('',(#24845,#24846,#24847,#24848));
#6768=EDGE_LOOP('',(#24849,#24850,#24851,#24852));
#6769=EDGE_LOOP('',(#24853,#24854,#24855,#24856));
#6770=EDGE_LOOP('',(#24857,#24858,#24859,#24860));
#6771=EDGE_LOOP('',(#24861,#24862,#24863,#24864));
#6772=EDGE_LOOP('',(#24865,#24866,#24867,#24868));
#6773=EDGE_LOOP('',(#24869,#24870,#24871,#24872));
#6774=EDGE_LOOP('',(#24873,#24874,#24875,#24876));
#6775=EDGE_LOOP('',(#24877,#24878,#24879,#24880));
#6776=EDGE_LOOP('',(#24881,#24882,#24883,#24884));
#6777=EDGE_LOOP('',(#24885,#24886,#24887,#24888));
#6778=EDGE_LOOP('',(#24889,#24890,#24891,#24892));
#6779=EDGE_LOOP('',(#24893,#24894,#24895,#24896));
#6780=EDGE_LOOP('',(#24897,#24898,#24899,#24900,#24901));
#6781=EDGE_LOOP('',(#24902,#24903,#24904,#24905,#24906,#24907,#24908,#24909,
#24910,#24911,#24912,#24913,#24914,#24915,#24916,#24917,#24918,#24919,#24920,
#24921,#24922,#24923,#24924,#24925,#24926,#24927,#24928,#24929,#24930,#24931,
#24932,#24933,#24934,#24935,#24936,#24937,#24938,#24939,#24940,#24941,#24942,
#24943,#24944,#24945,#24946,#24947,#24948,#24949,#24950,#24951,#24952,#24953,
#24954,#24955,#24956,#24957,#24958,#24959,#24960,#24961,#24962,#24963,#24964,
#24965,#24966,#24967,#24968,#24969,#24970,#24971,#24972,#24973,#24974,#24975,
#24976,#24977,#24978,#24979,#24980,#24981,#24982,#24983,#24984,#24985,#24986,
#24987,#24988,#24989,#24990,#24991,#24992,#24993,#24994,#24995,#24996,#24997,
#24998,#24999,#25000,#25001,#25002,#25003,#25004,#25005,#25006,#25007,#25008,
#25009,#25010,#25011,#25012,#25013,#25014,#25015,#25016,#25017,#25018,#25019,
#25020,#25021,#25022,#25023,#25024,#25025,#25026,#25027,#25028,#25029,#25030,
#25031,#25032,#25033,#25034,#25035,#25036,#25037,#25038,#25039,#25040,#25041,
#25042,#25043));
#6782=EDGE_LOOP('',(#25044,#25045,#25046,#25047,#25048));
#6783=EDGE_LOOP('',(#25049,#25050,#25051,#25052));
#6784=EDGE_LOOP('',(#25053,#25054,#25055,#25056,#25057,#25058,#25059,#25060,
#25061,#25062,#25063,#25064,#25065,#25066,#25067,#25068,#25069,#25070,#25071,
#25072,#25073,#25074,#25075,#25076,#25077,#25078,#25079,#25080,#25081,#25082,
#25083,#25084,#25085,#25086,#25087,#25088,#25089,#25090,#25091,#25092,#25093,
#25094,#25095,#25096,#25097,#25098,#25099,#25100,#25101,#25102,#25103,#25104,
#25105,#25106,#25107,#25108,#25109,#25110,#25111,#25112,#25113,#25114,#25115,
#25116,#25117,#25118,#25119,#25120,#25121,#25122,#25123,#25124,#25125,#25126,
#25127,#25128,#25129,#25130,#25131,#25132,#25133,#25134,#25135,#25136,#25137,
#25138,#25139,#25140,#25141,#25142,#25143,#25144,#25145,#25146,#25147,#25148,
#25149,#25150,#25151,#25152,#25153,#25154,#25155,#25156,#25157,#25158,#25159,
#25160,#25161,#25162,#25163,#25164,#25165,#25166,#25167,#25168,#25169,#25170,
#25171,#25172,#25173,#25174,#25175,#25176,#25177,#25178,#25179,#25180,#25181,
#25182,#25183,#25184,#25185,#25186,#25187,#25188,#25189,#25190,#25191,#25192,
#25193,#25194));
#6785=EDGE_LOOP('',(#25195,#25196,#25197,#25198,#25199,#25200));
#6786=EDGE_LOOP('',(#25201,#25202,#25203,#25204));
#6787=EDGE_LOOP('',(#25205));
#6788=EDGE_LOOP('',(#25206));
#6789=EDGE_LOOP('',(#25207,#25208,#25209,#25210));
#6790=EDGE_LOOP('',(#25211,#25212,#25213));
#6791=EDGE_LOOP('',(#25214,#25215,#25216,#25217));
#6792=EDGE_LOOP('',(#25218,#25219,#25220));
#6793=EDGE_LOOP('',(#25221,#25222,#25223,#25224));
#6794=EDGE_LOOP('',(#25225,#25226,#25227));
#6795=EDGE_LOOP('',(#25228,#25229,#25230,#25231));
#6796=EDGE_LOOP('',(#25232,#25233,#25234));
#6797=EDGE_LOOP('',(#25235,#25236,#25237,#25238));
#6798=EDGE_LOOP('',(#25239,#25240,#25241));
#6799=EDGE_LOOP('',(#25242,#25243,#25244,#25245));
#6800=EDGE_LOOP('',(#25246,#25247,#25248));
#6801=EDGE_LOOP('',(#25249,#25250,#25251,#25252));
#6802=EDGE_LOOP('',(#25253,#25254,#25255));
#6803=EDGE_LOOP('',(#25256,#25257,#25258,#25259));
#6804=EDGE_LOOP('',(#25260,#25261,#25262));
#6805=EDGE_LOOP('',(#25263,#25264,#25265,#25266));
#6806=EDGE_LOOP('',(#25267,#25268,#25269));
#6807=EDGE_LOOP('',(#25270,#25271,#25272,#25273));
#6808=EDGE_LOOP('',(#25274,#25275,#25276));
#6809=EDGE_LOOP('',(#25277,#25278,#25279,#25280));
#6810=EDGE_LOOP('',(#25281,#25282,#25283));
#6811=EDGE_LOOP('',(#25284,#25285,#25286,#25287));
#6812=EDGE_LOOP('',(#25288,#25289,#25290));
#6813=EDGE_LOOP('',(#25291,#25292,#25293,#25294));
#6814=EDGE_LOOP('',(#25295,#25296,#25297));
#6815=EDGE_LOOP('',(#25298,#25299,#25300,#25301));
#6816=EDGE_LOOP('',(#25302,#25303,#25304));
#6817=EDGE_LOOP('',(#25305,#25306,#25307,#25308));
#6818=EDGE_LOOP('',(#25309,#25310,#25311));
#6819=EDGE_LOOP('',(#25312,#25313,#25314,#25315));
#6820=EDGE_LOOP('',(#25316,#25317,#25318));
#6821=EDGE_LOOP('',(#25319,#25320,#25321,#25322));
#6822=EDGE_LOOP('',(#25323,#25324,#25325));
#6823=EDGE_LOOP('',(#25326,#25327,#25328,#25329));
#6824=EDGE_LOOP('',(#25330,#25331,#25332));
#6825=EDGE_LOOP('',(#25333,#25334,#25335,#25336));
#6826=EDGE_LOOP('',(#25337,#25338,#25339));
#6827=EDGE_LOOP('',(#25340,#25341,#25342,#25343));
#6828=EDGE_LOOP('',(#25344,#25345,#25346));
#6829=EDGE_LOOP('',(#25347,#25348,#25349,#25350));
#6830=EDGE_LOOP('',(#25351,#25352,#25353));
#6831=EDGE_LOOP('',(#25354,#25355,#25356,#25357));
#6832=EDGE_LOOP('',(#25358,#25359,#25360));
#6833=EDGE_LOOP('',(#25361,#25362,#25363,#25364));
#6834=EDGE_LOOP('',(#25365,#25366,#25367));
#6835=EDGE_LOOP('',(#25368,#25369,#25370,#25371));
#6836=EDGE_LOOP('',(#25372,#25373,#25374));
#6837=EDGE_LOOP('',(#25375,#25376,#25377,#25378));
#6838=EDGE_LOOP('',(#25379,#25380,#25381));
#6839=EDGE_LOOP('',(#25382,#25383,#25384,#25385));
#6840=EDGE_LOOP('',(#25386,#25387,#25388));
#6841=EDGE_LOOP('',(#25389,#25390,#25391,#25392));
#6842=EDGE_LOOP('',(#25393,#25394,#25395));
#6843=EDGE_LOOP('',(#25396,#25397,#25398,#25399));
#6844=EDGE_LOOP('',(#25400,#25401,#25402));
#6845=EDGE_LOOP('',(#25403,#25404,#25405,#25406));
#6846=EDGE_LOOP('',(#25407,#25408,#25409));
#6847=EDGE_LOOP('',(#25410,#25411,#25412,#25413));
#6848=EDGE_LOOP('',(#25414,#25415,#25416));
#6849=EDGE_LOOP('',(#25417,#25418,#25419,#25420));
#6850=EDGE_LOOP('',(#25421,#25422,#25423));
#6851=EDGE_LOOP('',(#25424,#25425,#25426,#25427));
#6852=EDGE_LOOP('',(#25428,#25429,#25430));
#6853=EDGE_LOOP('',(#25431,#25432,#25433,#25434));
#6854=EDGE_LOOP('',(#25435,#25436,#25437));
#6855=EDGE_LOOP('',(#25438,#25439,#25440,#25441));
#6856=EDGE_LOOP('',(#25442,#25443,#25444));
#6857=EDGE_LOOP('',(#25445,#25446,#25447,#25448));
#6858=EDGE_LOOP('',(#25449,#25450,#25451,#25452));
#6859=EDGE_LOOP('',(#25453,#25454,#25455,#25456));
#6860=EDGE_LOOP('',(#25457,#25458,#25459,#25460));
#6861=EDGE_LOOP('',(#25461,#25462,#25463,#25464));
#6862=EDGE_LOOP('',(#25465,#25466,#25467));
#6863=EDGE_LOOP('',(#25468,#25469,#25470,#25471));
#6864=EDGE_LOOP('',(#25472,#25473,#25474));
#6865=EDGE_LOOP('',(#25475,#25476,#25477,#25478));
#6866=EDGE_LOOP('',(#25479,#25480,#25481));
#6867=EDGE_LOOP('',(#25482,#25483,#25484,#25485));
#6868=EDGE_LOOP('',(#25486,#25487,#25488));
#6869=EDGE_LOOP('',(#25489,#25490,#25491,#25492));
#6870=EDGE_LOOP('',(#25493,#25494,#25495));
#6871=EDGE_LOOP('',(#25496,#25497,#25498,#25499));
#6872=EDGE_LOOP('',(#25500,#25501,#25502));
#6873=EDGE_LOOP('',(#25503,#25504,#25505,#25506));
#6874=EDGE_LOOP('',(#25507,#25508,#25509));
#6875=EDGE_LOOP('',(#25510,#25511,#25512,#25513));
#6876=EDGE_LOOP('',(#25514,#25515,#25516));
#6877=EDGE_LOOP('',(#25517,#25518,#25519,#25520));
#6878=EDGE_LOOP('',(#25521,#25522,#25523));
#6879=EDGE_LOOP('',(#25524,#25525,#25526,#25527));
#6880=EDGE_LOOP('',(#25528,#25529,#25530));
#6881=EDGE_LOOP('',(#25531,#25532,#25533,#25534));
#6882=EDGE_LOOP('',(#25535,#25536,#25537));
#6883=EDGE_LOOP('',(#25538,#25539,#25540,#25541));
#6884=EDGE_LOOP('',(#25542,#25543,#25544));
#6885=EDGE_LOOP('',(#25545,#25546,#25547,#25548));
#6886=EDGE_LOOP('',(#25549,#25550,#25551));
#6887=EDGE_LOOP('',(#25552,#25553,#25554,#25555));
#6888=EDGE_LOOP('',(#25556,#25557,#25558));
#6889=EDGE_LOOP('',(#25559,#25560,#25561,#25562));
#6890=EDGE_LOOP('',(#25563,#25564,#25565));
#6891=EDGE_LOOP('',(#25566,#25567,#25568,#25569));
#6892=EDGE_LOOP('',(#25570,#25571,#25572));
#6893=EDGE_LOOP('',(#25573,#25574,#25575,#25576));
#6894=EDGE_LOOP('',(#25577,#25578,#25579));
#6895=EDGE_LOOP('',(#25580,#25581,#25582,#25583));
#6896=EDGE_LOOP('',(#25584,#25585,#25586));
#6897=EDGE_LOOP('',(#25587,#25588,#25589,#25590));
#6898=EDGE_LOOP('',(#25591,#25592,#25593));
#6899=EDGE_LOOP('',(#25594,#25595,#25596,#25597));
#6900=EDGE_LOOP('',(#25598,#25599,#25600));
#6901=EDGE_LOOP('',(#25601,#25602,#25603,#25604));
#6902=EDGE_LOOP('',(#25605,#25606,#25607));
#6903=EDGE_LOOP('',(#25608,#25609,#25610,#25611));
#6904=EDGE_LOOP('',(#25612,#25613,#25614));
#6905=EDGE_LOOP('',(#25615,#25616,#25617,#25618));
#6906=EDGE_LOOP('',(#25619,#25620,#25621));
#6907=EDGE_LOOP('',(#25622,#25623,#25624,#25625));
#6908=EDGE_LOOP('',(#25626,#25627,#25628));
#6909=EDGE_LOOP('',(#25629,#25630,#25631,#25632));
#6910=EDGE_LOOP('',(#25633,#25634,#25635));
#6911=EDGE_LOOP('',(#25636,#25637,#25638,#25639));
#6912=EDGE_LOOP('',(#25640,#25641,#25642));
#6913=EDGE_LOOP('',(#25643,#25644,#25645,#25646));
#6914=EDGE_LOOP('',(#25647,#25648,#25649));
#6915=EDGE_LOOP('',(#25650,#25651,#25652,#25653));
#6916=EDGE_LOOP('',(#25654,#25655,#25656));
#6917=EDGE_LOOP('',(#25657,#25658,#25659,#25660));
#6918=EDGE_LOOP('',(#25661,#25662,#25663));
#6919=EDGE_LOOP('',(#25664,#25665,#25666,#25667));
#6920=EDGE_LOOP('',(#25668,#25669,#25670));
#6921=EDGE_LOOP('',(#25671,#25672,#25673,#25674));
#6922=EDGE_LOOP('',(#25675,#25676,#25677));
#6923=EDGE_LOOP('',(#25678,#25679,#25680,#25681));
#6924=EDGE_LOOP('',(#25682,#25683,#25684));
#6925=EDGE_LOOP('',(#25685,#25686,#25687,#25688));
#6926=EDGE_LOOP('',(#25689,#25690,#25691));
#6927=EDGE_LOOP('',(#25692,#25693,#25694,#25695));
#6928=EDGE_LOOP('',(#25696,#25697,#25698));
#6929=EDGE_LOOP('',(#25699,#25700,#25701,#25702));
#6930=EDGE_LOOP('',(#25703,#25704,#25705));
#6931=EDGE_LOOP('',(#25706,#25707,#25708,#25709));
#6932=EDGE_LOOP('',(#25710,#25711,#25712));
#6933=EDGE_LOOP('',(#25713,#25714,#25715));
#6934=EDGE_LOOP('',(#25716,#25717,#25718,#25719));
#6935=EDGE_LOOP('',(#25720,#25721,#25722,#25723));
#6936=EDGE_LOOP('',(#25724,#25725,#25726,#25727));
#6937=EDGE_LOOP('',(#25728,#25729,#25730,#25731));
#6938=EDGE_LOOP('',(#25732,#25733,#25734,#25735));
#6939=EDGE_LOOP('',(#25736,#25737,#25738,#25739));
#6940=EDGE_LOOP('',(#25740,#25741,#25742,#25743,#25744,#25745));
#6941=EDGE_LOOP('',(#25746));
#6942=EDGE_LOOP('',(#25747));
#6943=EDGE_LOOP('',(#25748,#25749,#25750,#25751,#25752,#25753));
#6944=EDGE_LOOP('',(#25754,#25755,#25756,#25757,#25758,#25759,#25760,#25761,
#25762,#25763,#25764,#25765));
#6945=EDGE_LOOP('',(#25766,#25767,#25768,#25769));
#6946=EDGE_LOOP('',(#25770,#25771,#25772,#25773));
#6947=EDGE_LOOP('',(#25774,#25775,#25776,#25777));
#6948=EDGE_LOOP('',(#25778,#25779,#25780,#25781));
#6949=EDGE_LOOP('',(#25782,#25783,#25784,#25785));
#6950=EDGE_LOOP('',(#25786,#25787,#25788,#25789));
#6951=EDGE_LOOP('',(#25790,#25791,#25792,#25793));
#6952=EDGE_LOOP('',(#25794,#25795,#25796,#25797));
#6953=EDGE_LOOP('',(#25798,#25799,#25800,#25801));
#6954=EDGE_LOOP('',(#25802,#25803,#25804,#25805));
#6955=EDGE_LOOP('',(#25806,#25807,#25808,#25809));
#6956=EDGE_LOOP('',(#25810,#25811,#25812,#25813));
#6957=EDGE_LOOP('',(#25814,#25815,#25816,#25817));
#6958=EDGE_LOOP('',(#25818,#25819,#25820,#25821));
#6959=EDGE_LOOP('',(#25822,#25823,#25824,#25825));
#6960=EDGE_LOOP('',(#25826,#25827,#25828,#25829));
#6961=EDGE_LOOP('',(#25830,#25831,#25832,#25833));
#6962=EDGE_LOOP('',(#25834,#25835,#25836,#25837));
#6963=EDGE_LOOP('',(#25838,#25839,#25840,#25841));
#6964=EDGE_LOOP('',(#25842,#25843,#25844,#25845));
#6965=EDGE_LOOP('',(#25846,#25847,#25848,#25849));
#6966=EDGE_LOOP('',(#25850,#25851,#25852,#25853));
#6967=EDGE_LOOP('',(#25854,#25855,#25856,#25857));
#6968=EDGE_LOOP('',(#25858,#25859,#25860,#25861));
#6969=EDGE_LOOP('',(#25862,#25863,#25864,#25865));
#6970=EDGE_LOOP('',(#25866,#25867,#25868,#25869));
#6971=EDGE_LOOP('',(#25870,#25871,#25872,#25873));
#6972=EDGE_LOOP('',(#25874,#25875,#25876,#25877));
#6973=EDGE_LOOP('',(#25878,#25879,#25880,#25881));
#6974=EDGE_LOOP('',(#25882,#25883,#25884,#25885));
#6975=EDGE_LOOP('',(#25886,#25887,#25888,#25889));
#6976=EDGE_LOOP('',(#25890,#25891,#25892,#25893));
#6977=EDGE_LOOP('',(#25894,#25895,#25896,#25897));
#6978=EDGE_LOOP('',(#25898,#25899,#25900,#25901));
#6979=EDGE_LOOP('',(#25902,#25903,#25904,#25905));
#6980=EDGE_LOOP('',(#25906,#25907,#25908,#25909));
#6981=EDGE_LOOP('',(#25910));
#6982=EDGE_LOOP('',(#25911,#25912,#25913,#25914,#25915,#25916));
#8845=LINE('',#56001,#11151);
#8846=LINE('',#56025,#11152);
#8847=LINE('',#56073,#11153);
#8848=LINE('',#56121,#11154);
#8849=LINE('',#56169,#11155);
#8850=LINE('',#56223,#11156);
#8851=LINE('',#56271,#11157);
#8852=LINE('',#56319,#11158);
#8853=LINE('',#56373,#11159);
#8854=LINE('',#56421,#11160);
#8855=LINE('',#56469,#11161);
#8856=LINE('',#56517,#11162);
#8857=LINE('',#56571,#11163);
#8858=LINE('',#56619,#11164);
#8859=LINE('',#56667,#11165);
#8860=LINE('',#56721,#11166);
#8861=LINE('',#56769,#11167);
#8862=LINE('',#56817,#11168);
#8863=LINE('',#56865,#11169);
#8864=LINE('',#56919,#11170);
#8865=LINE('',#56967,#11171);
#8866=LINE('',#57015,#11172);
#8867=LINE('',#57069,#11173);
#8868=LINE('',#57117,#11174);
#8869=LINE('',#57165,#11175);
#8870=LINE('',#57213,#11176);
#8871=LINE('',#57267,#11177);
#8872=LINE('',#57315,#11178);
#8873=LINE('',#57363,#11179);
#8874=LINE('',#57417,#11180);
#8875=LINE('',#57465,#11181);
#8876=LINE('',#57513,#11182);
#8877=LINE('',#57561,#11183);
#8878=LINE('',#57615,#11184);
#8879=LINE('',#57663,#11185);
#8880=LINE('',#57711,#11186);
#8881=LINE('',#57765,#11187);
#8882=LINE('',#57813,#11188);
#8883=LINE('',#57861,#11189);
#8884=LINE('',#57909,#11190);
#8885=LINE('',#57963,#11191);
#8886=LINE('',#58011,#11192);
#8887=LINE('',#58059,#11193);
#8888=LINE('',#58113,#11194);
#8889=LINE('',#58161,#11195);
#8890=LINE('',#58209,#11196);
#8891=LINE('',#58257,#11197);
#8892=LINE('',#58311,#11198);
#8893=LINE('',#58359,#11199);
#8894=LINE('',#58407,#11200);
#8895=LINE('',#58461,#11201);
#8896=LINE('',#58509,#11202);
#8897=LINE('',#58557,#11203);
#8898=LINE('',#58605,#11204);
#8899=LINE('',#58659,#11205);
#8900=LINE('',#58707,#11206);
#8901=LINE('',#58755,#11207);
#8902=LINE('',#58809,#11208);
#8903=LINE('',#58857,#11209);
#8904=LINE('',#58905,#11210);
#8905=LINE('',#58953,#11211);
#8906=LINE('',#59007,#11212);
#8907=LINE('',#59055,#11213);
#8908=LINE('',#59103,#11214);
#8909=LINE('',#59157,#11215);
#8910=LINE('',#59205,#11216);
#8911=LINE('',#59253,#11217);
#8912=LINE('',#59301,#11218);
#8913=LINE('',#59355,#11219);
#8914=LINE('',#59403,#11220);
#8915=LINE('',#59419,#11221);
#8916=LINE('',#59443,#11222);
#8917=LINE('',#59468,#11223);
#8918=LINE('',#59493,#11224);
#8919=LINE('',#59517,#11225);
#8920=LINE('',#59541,#11226);
#8921=LINE('',#59566,#11227);
#8922=LINE('',#59591,#11228);
#8923=LINE('',#59615,#11229);
#8924=LINE('',#59640,#11230);
#8925=LINE('',#59665,#11231);
#8926=LINE('',#59689,#11232);
#8927=LINE('',#59713,#11233);
#8928=LINE('',#59738,#11234);
#8929=LINE('',#59763,#11235);
#8930=LINE('',#59787,#11236);
#8931=LINE('',#59812,#11237);
#8932=LINE('',#59837,#11238);
#8933=LINE('',#59861,#11239);
#8934=LINE('',#59885,#11240);
#8935=LINE('',#59910,#11241);
#8936=LINE('',#59935,#11242);
#8937=LINE('',#59959,#11243);
#8938=LINE('',#59984,#11244);
#8939=LINE('',#60009,#11245);
#8940=LINE('',#60033,#11246);
#8941=LINE('',#60057,#11247);
#8942=LINE('',#60082,#11248);
#8943=LINE('',#60107,#11249);
#8944=LINE('',#60131,#11250);
#8945=LINE('',#60156,#11251);
#8946=LINE('',#60181,#11252);
#8947=LINE('',#60205,#11253);
#8948=LINE('',#60229,#11254);
#8949=LINE('',#60254,#11255);
#8950=LINE('',#60279,#11256);
#8951=LINE('',#60303,#11257);
#8952=LINE('',#60328,#11258);
#8953=LINE('',#60353,#11259);
#8954=LINE('',#60377,#11260);
#8955=LINE('',#60401,#11261);
#8956=LINE('',#60426,#11262);
#8957=LINE('',#60451,#11263);
#8958=LINE('',#60475,#11264);
#8959=LINE('',#60500,#11265);
#8960=LINE('',#60525,#11266);
#8961=LINE('',#60549,#11267);
#8962=LINE('',#60573,#11268);
#8963=LINE('',#60598,#11269);
#8964=LINE('',#60623,#11270);
#8965=LINE('',#60647,#11271);
#8966=LINE('',#60672,#11272);
#8967=LINE('',#60697,#11273);
#8968=LINE('',#60721,#11274);
#8969=LINE('',#60745,#11275);
#8970=LINE('',#60770,#11276);
#8971=LINE('',#60795,#11277);
#8972=LINE('',#60819,#11278);
#8973=LINE('',#60844,#11279);
#8974=LINE('',#60869,#11280);
#8975=LINE('',#60893,#11281);
#8976=LINE('',#60917,#11282);
#8977=LINE('',#60942,#11283);
#8978=LINE('',#60967,#11284);
#8979=LINE('',#60991,#11285);
#8980=LINE('',#61016,#11286);
#8981=LINE('',#61041,#11287);
#8982=LINE('',#61065,#11288);
#8983=LINE('',#64996,#11289);
#8984=LINE('',#64998,#11290);
#8985=LINE('',#65000,#11291);
#8986=LINE('',#65001,#11292);
#8987=LINE('',#65005,#11293);
#8988=LINE('',#65008,#11294);
#8989=LINE('',#65009,#11295);
#8990=LINE('',#65015,#11296);
#8991=LINE('',#65017,#11297);
#8992=LINE('',#65019,#11298);
#8993=LINE('',#65020,#11299);
#8994=LINE('',#65024,#11300);
#8995=LINE('',#65027,#11301);
#8996=LINE('',#65028,#11302);
#8997=LINE('',#65034,#11303);
#8998=LINE('',#65036,#11304);
#8999=LINE('',#65038,#11305);
#9000=LINE('',#65039,#11306);
#9001=LINE('',#65043,#11307);
#9002=LINE('',#65046,#11308);
#9003=LINE('',#65047,#11309);
#9004=LINE('',#65053,#11310);
#9005=LINE('',#65055,#11311);
#9006=LINE('',#65057,#11312);
#9007=LINE('',#65058,#11313);
#9008=LINE('',#65062,#11314);
#9009=LINE('',#65065,#11315);
#9010=LINE('',#65066,#11316);
#9011=LINE('',#65072,#11317);
#9012=LINE('',#65074,#11318);
#9013=LINE('',#65076,#11319);
#9014=LINE('',#65077,#11320);
#9015=LINE('',#65081,#11321);
#9016=LINE('',#65084,#11322);
#9017=LINE('',#65085,#11323);
#9018=LINE('',#65091,#11324);
#9019=LINE('',#65093,#11325);
#9020=LINE('',#65095,#11326);
#9021=LINE('',#65096,#11327);
#9022=LINE('',#65100,#11328);
#9023=LINE('',#65103,#11329);
#9024=LINE('',#65104,#11330);
#9025=LINE('',#65110,#11331);
#9026=LINE('',#65112,#11332);
#9027=LINE('',#65114,#11333);
#9028=LINE('',#65115,#11334);
#9029=LINE('',#65119,#11335);
#9030=LINE('',#65122,#11336);
#9031=LINE('',#65123,#11337);
#9032=LINE('',#65129,#11338);
#9033=LINE('',#65131,#11339);
#9034=LINE('',#65133,#11340);
#9035=LINE('',#65134,#11341);
#9036=LINE('',#65138,#11342);
#9037=LINE('',#65141,#11343);
#9038=LINE('',#65142,#11344);
#9039=LINE('',#65148,#11345);
#9040=LINE('',#65150,#11346);
#9041=LINE('',#65152,#11347);
#9042=LINE('',#65153,#11348);
#9043=LINE('',#65157,#11349);
#9044=LINE('',#65160,#11350);
#9045=LINE('',#65161,#11351);
#9046=LINE('',#65167,#11352);
#9047=LINE('',#65169,#11353);
#9048=LINE('',#65171,#11354);
#9049=LINE('',#65172,#11355);
#9050=LINE('',#65176,#11356);
#9051=LINE('',#65179,#11357);
#9052=LINE('',#65180,#11358);
#9053=LINE('',#65186,#11359);
#9054=LINE('',#65188,#11360);
#9055=LINE('',#65190,#11361);
#9056=LINE('',#65191,#11362);
#9057=LINE('',#65195,#11363);
#9058=LINE('',#65198,#11364);
#9059=LINE('',#65199,#11365);
#9060=LINE('',#65205,#11366);
#9061=LINE('',#65207,#11367);
#9062=LINE('',#65209,#11368);
#9063=LINE('',#65210,#11369);
#9064=LINE('',#65214,#11370);
#9065=LINE('',#65217,#11371);
#9066=LINE('',#65218,#11372);
#9067=LINE('',#65224,#11373);
#9068=LINE('',#65226,#11374);
#9069=LINE('',#65228,#11375);
#9070=LINE('',#65229,#11376);
#9071=LINE('',#65233,#11377);
#9072=LINE('',#65236,#11378);
#9073=LINE('',#65237,#11379);
#9074=LINE('',#65243,#11380);
#9075=LINE('',#65245,#11381);
#9076=LINE('',#65247,#11382);
#9077=LINE('',#65248,#11383);
#9078=LINE('',#65252,#11384);
#9079=LINE('',#65255,#11385);
#9080=LINE('',#65256,#11386);
#9081=LINE('',#65262,#11387);
#9082=LINE('',#65264,#11388);
#9083=LINE('',#65266,#11389);
#9084=LINE('',#65267,#11390);
#9085=LINE('',#65271,#11391);
#9086=LINE('',#65274,#11392);
#9087=LINE('',#65275,#11393);
#9088=LINE('',#65281,#11394);
#9089=LINE('',#65283,#11395);
#9090=LINE('',#65285,#11396);
#9091=LINE('',#65286,#11397);
#9092=LINE('',#65290,#11398);
#9093=LINE('',#65293,#11399);
#9094=LINE('',#65294,#11400);
#9095=LINE('',#65300,#11401);
#9096=LINE('',#65302,#11402);
#9097=LINE('',#65304,#11403);
#9098=LINE('',#65305,#11404);
#9099=LINE('',#65309,#11405);
#9100=LINE('',#65312,#11406);
#9101=LINE('',#65313,#11407);
#9102=LINE('',#65319,#11408);
#9103=LINE('',#65321,#11409);
#9104=LINE('',#65323,#11410);
#9105=LINE('',#65324,#11411);
#9106=LINE('',#65329,#11412);
#9107=LINE('',#65333,#11413);
#9108=LINE('',#65334,#11414);
#9109=LINE('',#65342,#11415);
#9110=LINE('',#65344,#11416);
#9111=LINE('',#65346,#11417);
#9112=LINE('',#65347,#11418);
#9113=LINE('',#65351,#11419);
#9114=LINE('',#65354,#11420);
#9115=LINE('',#65355,#11421);
#9116=LINE('',#65361,#11422);
#9117=LINE('',#65363,#11423);
#9118=LINE('',#65365,#11424);
#9119=LINE('',#65366,#11425);
#9120=LINE('',#65370,#11426);
#9121=LINE('',#65373,#11427);
#9122=LINE('',#65374,#11428);
#9123=LINE('',#65380,#11429);
#9124=LINE('',#65382,#11430);
#9125=LINE('',#65384,#11431);
#9126=LINE('',#65385,#11432);
#9127=LINE('',#65389,#11433);
#9128=LINE('',#65392,#11434);
#9129=LINE('',#65393,#11435);
#9130=LINE('',#65399,#11436);
#9131=LINE('',#65401,#11437);
#9132=LINE('',#65403,#11438);
#9133=LINE('',#65404,#11439);
#9134=LINE('',#65408,#11440);
#9135=LINE('',#65411,#11441);
#9136=LINE('',#65412,#11442);
#9137=LINE('',#65418,#11443);
#9138=LINE('',#65420,#11444);
#9139=LINE('',#65422,#11445);
#9140=LINE('',#65423,#11446);
#9141=LINE('',#65427,#11447);
#9142=LINE('',#65430,#11448);
#9143=LINE('',#65431,#11449);
#9144=LINE('',#65437,#11450);
#9145=LINE('',#65439,#11451);
#9146=LINE('',#65441,#11452);
#9147=LINE('',#65442,#11453);
#9148=LINE('',#65446,#11454);
#9149=LINE('',#65449,#11455);
#9150=LINE('',#65450,#11456);
#9151=LINE('',#65456,#11457);
#9152=LINE('',#65458,#11458);
#9153=LINE('',#65460,#11459);
#9154=LINE('',#65461,#11460);
#9155=LINE('',#65465,#11461);
#9156=LINE('',#65468,#11462);
#9157=LINE('',#65469,#11463);
#9158=LINE('',#65475,#11464);
#9159=LINE('',#65477,#11465);
#9160=LINE('',#65479,#11466);
#9161=LINE('',#65480,#11467);
#9162=LINE('',#65484,#11468);
#9163=LINE('',#65487,#11469);
#9164=LINE('',#65488,#11470);
#9165=LINE('',#65494,#11471);
#9166=LINE('',#65496,#11472);
#9167=LINE('',#65498,#11473);
#9168=LINE('',#65499,#11474);
#9169=LINE('',#65503,#11475);
#9170=LINE('',#65506,#11476);
#9171=LINE('',#65507,#11477);
#9172=LINE('',#65513,#11478);
#9173=LINE('',#65515,#11479);
#9174=LINE('',#65517,#11480);
#9175=LINE('',#65518,#11481);
#9176=LINE('',#65522,#11482);
#9177=LINE('',#65525,#11483);
#9178=LINE('',#65526,#11484);
#9179=LINE('',#65532,#11485);
#9180=LINE('',#65534,#11486);
#9181=LINE('',#65536,#11487);
#9182=LINE('',#65537,#11488);
#9183=LINE('',#65541,#11489);
#9184=LINE('',#65544,#11490);
#9185=LINE('',#65545,#11491);
#9186=LINE('',#65551,#11492);
#9187=LINE('',#65553,#11493);
#9188=LINE('',#65555,#11494);
#9189=LINE('',#65556,#11495);
#9190=LINE('',#65560,#11496);
#9191=LINE('',#65563,#11497);
#9192=LINE('',#65564,#11498);
#9193=LINE('',#65570,#11499);
#9194=LINE('',#65572,#11500);
#9195=LINE('',#65574,#11501);
#9196=LINE('',#65575,#11502);
#9197=LINE('',#65579,#11503);
#9198=LINE('',#65582,#11504);
#9199=LINE('',#65583,#11505);
#9200=LINE('',#65589,#11506);
#9201=LINE('',#65591,#11507);
#9202=LINE('',#65593,#11508);
#9203=LINE('',#65594,#11509);
#9204=LINE('',#65598,#11510);
#9205=LINE('',#65601,#11511);
#9206=LINE('',#65602,#11512);
#9207=LINE('',#65608,#11513);
#9208=LINE('',#65610,#11514);
#9209=LINE('',#65612,#11515);
#9210=LINE('',#65613,#11516);
#9211=LINE('',#65617,#11517);
#9212=LINE('',#65620,#11518);
#9213=LINE('',#65621,#11519);
#9214=LINE('',#65627,#11520);
#9215=LINE('',#65629,#11521);
#9216=LINE('',#65631,#11522);
#9217=LINE('',#65632,#11523);
#9218=LINE('',#65636,#11524);
#9219=LINE('',#65639,#11525);
#9220=LINE('',#65640,#11526);
#9221=LINE('',#65646,#11527);
#9222=LINE('',#65648,#11528);
#9223=LINE('',#65650,#11529);
#9224=LINE('',#65651,#11530);
#9225=LINE('',#65655,#11531);
#9226=LINE('',#65658,#11532);
#9227=LINE('',#65659,#11533);
#9228=LINE('',#65665,#11534);
#9229=LINE('',#65667,#11535);
#9230=LINE('',#65669,#11536);
#9231=LINE('',#65670,#11537);
#9232=LINE('',#65674,#11538);
#9233=LINE('',#65677,#11539);
#9234=LINE('',#65678,#11540);
#9235=LINE('',#65684,#11541);
#9236=LINE('',#65689,#11542);
#9237=LINE('',#65691,#11543);
#9238=LINE('',#65693,#11544);
#9239=LINE('',#65694,#11545);
#9240=LINE('',#65697,#11546);
#9241=LINE('',#65699,#11547);
#9242=LINE('',#65700,#11548);
#9243=LINE('',#65703,#11549);
#9244=LINE('',#65705,#11550);
#9245=LINE('',#65706,#11551);
#9246=LINE('',#65709,#11552);
#9247=LINE('',#65711,#11553);
#9248=LINE('',#65712,#11554);
#9249=LINE('',#65715,#11555);
#9250=LINE('',#65717,#11556);
#9251=LINE('',#65718,#11557);
#9252=LINE('',#65720,#11558);
#9253=LINE('',#65721,#11559);
#9254=LINE('',#65727,#11560);
#9255=LINE('',#65731,#11561);
#9256=LINE('',#65732,#11562);
#9257=LINE('',#65736,#11563);
#11151=VECTOR('',#38008,1.5);
#11152=VECTOR('',#38013,1.5);
#11153=VECTOR('',#38016,1.5);
#11154=VECTOR('',#38019,1.5);
#11155=VECTOR('',#38022,1.5);
#11156=VECTOR('',#38025,1.5);
#11157=VECTOR('',#38028,1.5);
#11158=VECTOR('',#38031,1.5);
#11159=VECTOR('',#38034,1.5);
#11160=VECTOR('',#38037,1.5);
#11161=VECTOR('',#38040,1.5);
#11162=VECTOR('',#38043,1.5);
#11163=VECTOR('',#38046,1.5);
#11164=VECTOR('',#38049,1.5);
#11165=VECTOR('',#38052,1.5);
#11166=VECTOR('',#38055,1.5);
#11167=VECTOR('',#38058,1.5);
#11168=VECTOR('',#38061,1.5);
#11169=VECTOR('',#38064,1.5);
#11170=VECTOR('',#38067,1.5);
#11171=VECTOR('',#38070,1.5);
#11172=VECTOR('',#38073,1.5);
#11173=VECTOR('',#38076,1.5);
#11174=VECTOR('',#38079,1.5);
#11175=VECTOR('',#38082,1.5);
#11176=VECTOR('',#38085,1.5);
#11177=VECTOR('',#38088,1.5);
#11178=VECTOR('',#38091,1.5);
#11179=VECTOR('',#38094,1.5);
#11180=VECTOR('',#38097,1.5);
#11181=VECTOR('',#38100,1.5);
#11182=VECTOR('',#38103,1.5);
#11183=VECTOR('',#38106,1.5);
#11184=VECTOR('',#38109,1.5);
#11185=VECTOR('',#38112,1.5);
#11186=VECTOR('',#38115,1.5);
#11187=VECTOR('',#38118,1.5);
#11188=VECTOR('',#38121,1.5);
#11189=VECTOR('',#38124,1.5);
#11190=VECTOR('',#38127,1.5);
#11191=VECTOR('',#38130,1.5);
#11192=VECTOR('',#38133,1.5);
#11193=VECTOR('',#38136,1.5);
#11194=VECTOR('',#38139,1.5);
#11195=VECTOR('',#38142,1.5);
#11196=VECTOR('',#38145,1.5);
#11197=VECTOR('',#38148,1.5);
#11198=VECTOR('',#38151,1.5);
#11199=VECTOR('',#38154,1.5);
#11200=VECTOR('',#38157,1.5);
#11201=VECTOR('',#38160,1.5);
#11202=VECTOR('',#38163,1.5);
#11203=VECTOR('',#38166,1.5);
#11204=VECTOR('',#38169,1.5);
#11205=VECTOR('',#38172,1.5);
#11206=VECTOR('',#38175,1.5);
#11207=VECTOR('',#38178,1.5);
#11208=VECTOR('',#38181,1.5);
#11209=VECTOR('',#38184,1.5);
#11210=VECTOR('',#38187,1.5);
#11211=VECTOR('',#38190,1.5);
#11212=VECTOR('',#38193,1.5);
#11213=VECTOR('',#38196,1.5);
#11214=VECTOR('',#38199,1.5);
#11215=VECTOR('',#38202,1.5);
#11216=VECTOR('',#38205,1.5);
#11217=VECTOR('',#38208,1.5);
#11218=VECTOR('',#38211,1.5);
#11219=VECTOR('',#38214,1.5);
#11220=VECTOR('',#38217,1.17775);
#11221=VECTOR('',#38222,1.17775);
#11222=VECTOR('',#38225,1.17775);
#11223=VECTOR('',#38228,1.17775);
#11224=VECTOR('',#38231,1.17775);
#11225=VECTOR('',#38234,1.17775);
#11226=VECTOR('',#38237,1.17775);
#11227=VECTOR('',#38240,1.17775);
#11228=VECTOR('',#38243,1.17775);
#11229=VECTOR('',#38246,1.17775);
#11230=VECTOR('',#38249,1.17775);
#11231=VECTOR('',#38252,1.17775);
#11232=VECTOR('',#38255,1.17775);
#11233=VECTOR('',#38258,1.17775);
#11234=VECTOR('',#38261,1.17775);
#11235=VECTOR('',#38264,1.17775);
#11236=VECTOR('',#38267,1.17775);
#11237=VECTOR('',#38270,1.17775);
#11238=VECTOR('',#38273,1.17775);
#11239=VECTOR('',#38276,1.17775);
#11240=VECTOR('',#38279,1.17775);
#11241=VECTOR('',#38282,1.17775);
#11242=VECTOR('',#38285,1.17775);
#11243=VECTOR('',#38288,1.17775);
#11244=VECTOR('',#38291,1.17775);
#11245=VECTOR('',#38294,1.17775);
#11246=VECTOR('',#38297,1.17775);
#11247=VECTOR('',#38300,1.17775);
#11248=VECTOR('',#38303,1.17775);
#11249=VECTOR('',#38306,1.17775);
#11250=VECTOR('',#38309,1.17775);
#11251=VECTOR('',#38312,1.17775);
#11252=VECTOR('',#38315,1.17775);
#11253=VECTOR('',#38318,1.17775);
#11254=VECTOR('',#38321,1.17775);
#11255=VECTOR('',#38324,1.17775);
#11256=VECTOR('',#38327,1.17775);
#11257=VECTOR('',#38330,1.17775);
#11258=VECTOR('',#38333,1.17775);
#11259=VECTOR('',#38336,1.17775);
#11260=VECTOR('',#38339,1.17775);
#11261=VECTOR('',#38342,1.17775);
#11262=VECTOR('',#38345,1.17775);
#11263=VECTOR('',#38348,1.17775);
#11264=VECTOR('',#38351,1.17775);
#11265=VECTOR('',#38354,1.17775);
#11266=VECTOR('',#38357,1.17775);
#11267=VECTOR('',#38360,1.17775);
#11268=VECTOR('',#38363,1.17775);
#11269=VECTOR('',#38366,1.17775);
#11270=VECTOR('',#38369,1.17775);
#11271=VECTOR('',#38372,1.17775);
#11272=VECTOR('',#38375,1.17775);
#11273=VECTOR('',#38378,1.17775);
#11274=VECTOR('',#38381,1.17775);
#11275=VECTOR('',#38384,1.17775);
#11276=VECTOR('',#38387,1.17775);
#11277=VECTOR('',#38390,1.17775);
#11278=VECTOR('',#38393,1.17775);
#11279=VECTOR('',#38396,1.17775);
#11280=VECTOR('',#38399,1.17775);
#11281=VECTOR('',#38402,1.17775);
#11282=VECTOR('',#38405,1.17775);
#11283=VECTOR('',#38408,1.17775);
#11284=VECTOR('',#38411,1.17775);
#11285=VECTOR('',#38414,1.17775);
#11286=VECTOR('',#38417,1.17775);
#11287=VECTOR('',#38420,1.17775);
#11288=VECTOR('',#38423,1.17775);
#11289=VECTOR('',#38456,10.);
#11290=VECTOR('',#38457,10.);
#11291=VECTOR('',#38458,10.);
#11292=VECTOR('',#38459,10.);
#11293=VECTOR('',#38464,10.);
#11294=VECTOR('',#38467,10.);
#11295=VECTOR('',#38468,10.);
#11296=VECTOR('',#38475,10.);
#11297=VECTOR('',#38476,10.);
#11298=VECTOR('',#38477,10.);
#11299=VECTOR('',#38478,10.);
#11300=VECTOR('',#38483,10.);
#11301=VECTOR('',#38486,10.);
#11302=VECTOR('',#38487,10.);
#11303=VECTOR('',#38494,10.);
#11304=VECTOR('',#38495,10.);
#11305=VECTOR('',#38496,10.);
#11306=VECTOR('',#38497,10.);
#11307=VECTOR('',#38502,10.);
#11308=VECTOR('',#38505,10.);
#11309=VECTOR('',#38506,10.);
#11310=VECTOR('',#38513,10.);
#11311=VECTOR('',#38514,10.);
#11312=VECTOR('',#38515,10.);
#11313=VECTOR('',#38516,10.);
#11314=VECTOR('',#38521,10.);
#11315=VECTOR('',#38524,10.);
#11316=VECTOR('',#38525,10.);
#11317=VECTOR('',#38532,10.);
#11318=VECTOR('',#38533,10.);
#11319=VECTOR('',#38534,10.);
#11320=VECTOR('',#38535,10.);
#11321=VECTOR('',#38540,10.);
#11322=VECTOR('',#38543,10.);
#11323=VECTOR('',#38544,10.);
#11324=VECTOR('',#38551,10.);
#11325=VECTOR('',#38552,10.);
#11326=VECTOR('',#38553,10.);
#11327=VECTOR('',#38554,10.);
#11328=VECTOR('',#38559,10.);
#11329=VECTOR('',#38562,10.);
#11330=VECTOR('',#38563,10.);
#11331=VECTOR('',#38570,10.);
#11332=VECTOR('',#38571,10.);
#11333=VECTOR('',#38572,10.);
#11334=VECTOR('',#38573,10.);
#11335=VECTOR('',#38578,10.);
#11336=VECTOR('',#38581,10.);
#11337=VECTOR('',#38582,10.);
#11338=VECTOR('',#38589,10.);
#11339=VECTOR('',#38590,10.);
#11340=VECTOR('',#38591,10.);
#11341=VECTOR('',#38592,10.);
#11342=VECTOR('',#38597,10.);
#11343=VECTOR('',#38600,10.);
#11344=VECTOR('',#38601,10.);
#11345=VECTOR('',#38608,10.);
#11346=VECTOR('',#38609,10.);
#11347=VECTOR('',#38610,10.);
#11348=VECTOR('',#38611,10.);
#11349=VECTOR('',#38616,10.);
#11350=VECTOR('',#38619,10.);
#11351=VECTOR('',#38620,10.);
#11352=VECTOR('',#38627,10.);
#11353=VECTOR('',#38628,10.);
#11354=VECTOR('',#38629,10.);
#11355=VECTOR('',#38630,10.);
#11356=VECTOR('',#38635,10.);
#11357=VECTOR('',#38638,10.);
#11358=VECTOR('',#38639,10.);
#11359=VECTOR('',#38646,10.);
#11360=VECTOR('',#38647,10.);
#11361=VECTOR('',#38648,10.);
#11362=VECTOR('',#38649,10.);
#11363=VECTOR('',#38654,10.);
#11364=VECTOR('',#38657,10.);
#11365=VECTOR('',#38658,10.);
#11366=VECTOR('',#38665,10.);
#11367=VECTOR('',#38666,10.);
#11368=VECTOR('',#38667,10.);
#11369=VECTOR('',#38668,10.);
#11370=VECTOR('',#38673,10.);
#11371=VECTOR('',#38676,10.);
#11372=VECTOR('',#38677,10.);
#11373=VECTOR('',#38684,10.);
#11374=VECTOR('',#38685,10.);
#11375=VECTOR('',#38686,10.);
#11376=VECTOR('',#38687,10.);
#11377=VECTOR('',#38692,10.);
#11378=VECTOR('',#38695,10.);
#11379=VECTOR('',#38696,10.);
#11380=VECTOR('',#38703,10.);
#11381=VECTOR('',#38704,10.);
#11382=VECTOR('',#38705,10.);
#11383=VECTOR('',#38706,10.);
#11384=VECTOR('',#38711,10.);
#11385=VECTOR('',#38714,10.);
#11386=VECTOR('',#38715,10.);
#11387=VECTOR('',#38722,10.);
#11388=VECTOR('',#38723,10.);
#11389=VECTOR('',#38724,10.);
#11390=VECTOR('',#38725,10.);
#11391=VECTOR('',#38730,10.);
#11392=VECTOR('',#38733,10.);
#11393=VECTOR('',#38734,10.);
#11394=VECTOR('',#38741,10.);
#11395=VECTOR('',#38742,10.);
#11396=VECTOR('',#38743,10.);
#11397=VECTOR('',#38744,10.);
#11398=VECTOR('',#38749,10.);
#11399=VECTOR('',#38752,10.);
#11400=VECTOR('',#38753,10.);
#11401=VECTOR('',#38760,10.);
#11402=VECTOR('',#38761,10.);
#11403=VECTOR('',#38762,10.);
#11404=VECTOR('',#38763,10.);
#11405=VECTOR('',#38768,10.);
#11406=VECTOR('',#38771,10.);
#11407=VECTOR('',#38772,10.);
#11408=VECTOR('',#38779,10.);
#11409=VECTOR('',#38780,10.);
#11410=VECTOR('',#38781,10.);
#11411=VECTOR('',#38782,10.);
#11412=VECTOR('',#38787,10.);
#11413=VECTOR('',#38792,10.);
#11414=VECTOR('',#38793,10.);
#11415=VECTOR('',#38802,10.);
#11416=VECTOR('',#38803,10.);
#11417=VECTOR('',#38804,10.);
#11418=VECTOR('',#38805,10.);
#11419=VECTOR('',#38810,10.);
#11420=VECTOR('',#38813,10.);
#11421=VECTOR('',#38814,10.);
#11422=VECTOR('',#38821,10.);
#11423=VECTOR('',#38822,10.);
#11424=VECTOR('',#38823,10.);
#11425=VECTOR('',#38824,10.);
#11426=VECTOR('',#38829,10.);
#11427=VECTOR('',#38832,10.);
#11428=VECTOR('',#38833,10.);
#11429=VECTOR('',#38840,10.);
#11430=VECTOR('',#38841,10.);
#11431=VECTOR('',#38842,10.);
#11432=VECTOR('',#38843,10.);
#11433=VECTOR('',#38848,10.);
#11434=VECTOR('',#38851,10.);
#11435=VECTOR('',#38852,10.);
#11436=VECTOR('',#38859,10.);
#11437=VECTOR('',#38860,10.);
#11438=VECTOR('',#38861,10.);
#11439=VECTOR('',#38862,10.);
#11440=VECTOR('',#38867,10.);
#11441=VECTOR('',#38870,10.);
#11442=VECTOR('',#38871,10.);
#11443=VECTOR('',#38878,10.);
#11444=VECTOR('',#38879,10.);
#11445=VECTOR('',#38880,10.);
#11446=VECTOR('',#38881,10.);
#11447=VECTOR('',#38886,10.);
#11448=VECTOR('',#38889,10.);
#11449=VECTOR('',#38890,10.);
#11450=VECTOR('',#38897,10.);
#11451=VECTOR('',#38898,10.);
#11452=VECTOR('',#38899,10.);
#11453=VECTOR('',#38900,10.);
#11454=VECTOR('',#38905,10.);
#11455=VECTOR('',#38908,10.);
#11456=VECTOR('',#38909,10.);
#11457=VECTOR('',#38916,10.);
#11458=VECTOR('',#38917,10.);
#11459=VECTOR('',#38918,10.);
#11460=VECTOR('',#38919,10.);
#11461=VECTOR('',#38924,10.);
#11462=VECTOR('',#38927,10.);
#11463=VECTOR('',#38928,10.);
#11464=VECTOR('',#38935,10.);
#11465=VECTOR('',#38936,10.);
#11466=VECTOR('',#38937,10.);
#11467=VECTOR('',#38938,10.);
#11468=VECTOR('',#38943,10.);
#11469=VECTOR('',#38946,10.);
#11470=VECTOR('',#38947,10.);
#11471=VECTOR('',#38954,10.);
#11472=VECTOR('',#38955,10.);
#11473=VECTOR('',#38956,10.);
#11474=VECTOR('',#38957,10.);
#11475=VECTOR('',#38962,10.);
#11476=VECTOR('',#38965,10.);
#11477=VECTOR('',#38966,10.);
#11478=VECTOR('',#38973,10.);
#11479=VECTOR('',#38974,10.);
#11480=VECTOR('',#38975,10.);
#11481=VECTOR('',#38976,10.);
#11482=VECTOR('',#38981,10.);
#11483=VECTOR('',#38984,10.);
#11484=VECTOR('',#38985,10.);
#11485=VECTOR('',#38992,10.);
#11486=VECTOR('',#38993,10.);
#11487=VECTOR('',#38994,10.);
#11488=VECTOR('',#38995,10.);
#11489=VECTOR('',#39000,10.);
#11490=VECTOR('',#39003,10.);
#11491=VECTOR('',#39004,10.);
#11492=VECTOR('',#39011,10.);
#11493=VECTOR('',#39012,10.);
#11494=VECTOR('',#39013,10.);
#11495=VECTOR('',#39014,10.);
#11496=VECTOR('',#39019,10.);
#11497=VECTOR('',#39022,10.);
#11498=VECTOR('',#39023,10.);
#11499=VECTOR('',#39030,10.);
#11500=VECTOR('',#39031,10.);
#11501=VECTOR('',#39032,10.);
#11502=VECTOR('',#39033,10.);
#11503=VECTOR('',#39038,10.);
#11504=VECTOR('',#39041,10.);
#11505=VECTOR('',#39042,10.);
#11506=VECTOR('',#39049,10.);
#11507=VECTOR('',#39050,10.);
#11508=VECTOR('',#39051,10.);
#11509=VECTOR('',#39052,10.);
#11510=VECTOR('',#39057,10.);
#11511=VECTOR('',#39060,10.);
#11512=VECTOR('',#39061,10.);
#11513=VECTOR('',#39068,10.);
#11514=VECTOR('',#39069,10.);
#11515=VECTOR('',#39070,10.);
#11516=VECTOR('',#39071,10.);
#11517=VECTOR('',#39076,10.);
#11518=VECTOR('',#39079,10.);
#11519=VECTOR('',#39080,10.);
#11520=VECTOR('',#39087,10.);
#11521=VECTOR('',#39088,10.);
#11522=VECTOR('',#39089,10.);
#11523=VECTOR('',#39090,10.);
#11524=VECTOR('',#39095,10.);
#11525=VECTOR('',#39098,10.);
#11526=VECTOR('',#39099,10.);
#11527=VECTOR('',#39106,10.);
#11528=VECTOR('',#39107,10.);
#11529=VECTOR('',#39108,10.);
#11530=VECTOR('',#39109,10.);
#11531=VECTOR('',#39114,10.);
#11532=VECTOR('',#39117,10.);
#11533=VECTOR('',#39118,10.);
#11534=VECTOR('',#39125,10.);
#11535=VECTOR('',#39126,10.);
#11536=VECTOR('',#39127,10.);
#11537=VECTOR('',#39128,10.);
#11538=VECTOR('',#39133,10.);
#11539=VECTOR('',#39136,10.);
#11540=VECTOR('',#39137,10.);
#11541=VECTOR('',#39144,0.625);
#11542=VECTOR('',#39149,10.);
#11543=VECTOR('',#39150,10.);
#11544=VECTOR('',#39151,10.);
#11545=VECTOR('',#39152,10.);
#11546=VECTOR('',#39155,10.);
#11547=VECTOR('',#39156,10.);
#11548=VECTOR('',#39157,10.);
#11549=VECTOR('',#39160,10.);
#11550=VECTOR('',#39161,10.);
#11551=VECTOR('',#39162,10.);
#11552=VECTOR('',#39165,10.);
#11553=VECTOR('',#39166,10.);
#11554=VECTOR('',#39167,10.);
#11555=VECTOR('',#39170,10.);
#11556=VECTOR('',#39171,10.);
#11557=VECTOR('',#39172,10.);
#11558=VECTOR('',#39175,10.);
#11559=VECTOR('',#39176,10.);
#11560=VECTOR('',#39185,1.3);
#11561=VECTOR('',#39190,2.75);
#11562=VECTOR('',#39191,2.75);
#11563=VECTOR('',#39196,2.6);
#13613=VERTEX_POINT('',#55999);
#13614=VERTEX_POINT('',#56000);
#13615=VERTEX_POINT('',#56002);
#13616=VERTEX_POINT('',#56013);
#13617=VERTEX_POINT('',#56023);
#13618=VERTEX_POINT('',#56024);
#13619=VERTEX_POINT('',#56071);
#13620=VERTEX_POINT('',#56072);
#13621=VERTEX_POINT('',#56119);
#13622=VERTEX_POINT('',#56120);
#13623=VERTEX_POINT('',#56167);
#13624=VERTEX_POINT('',#56168);
#13625=VERTEX_POINT('',#56221);
#13626=VERTEX_POINT('',#56222);
#13627=VERTEX_POINT('',#56269);
#13628=VERTEX_POINT('',#56270);
#13629=VERTEX_POINT('',#56317);
#13630=VERTEX_POINT('',#56318);
#13631=VERTEX_POINT('',#56371);
#13632=VERTEX_POINT('',#56372);
#13633=VERTEX_POINT('',#56419);
#13634=VERTEX_POINT('',#56420);
#13635=VERTEX_POINT('',#56467);
#13636=VERTEX_POINT('',#56468);
#13637=VERTEX_POINT('',#56515);
#13638=VERTEX_POINT('',#56516);
#13639=VERTEX_POINT('',#56569);
#13640=VERTEX_POINT('',#56570);
#13641=VERTEX_POINT('',#56617);
#13642=VERTEX_POINT('',#56618);
#13643=VERTEX_POINT('',#56665);
#13644=VERTEX_POINT('',#56666);
#13645=VERTEX_POINT('',#56719);
#13646=VERTEX_POINT('',#56720);
#13647=VERTEX_POINT('',#56767);
#13648=VERTEX_POINT('',#56768);
#13649=VERTEX_POINT('',#56815);
#13650=VERTEX_POINT('',#56816);
#13651=VERTEX_POINT('',#56863);
#13652=VERTEX_POINT('',#56864);
#13653=VERTEX_POINT('',#56917);
#13654=VERTEX_POINT('',#56918);
#13655=VERTEX_POINT('',#56965);
#13656=VERTEX_POINT('',#56966);
#13657=VERTEX_POINT('',#57013);
#13658=VERTEX_POINT('',#57014);
#13659=VERTEX_POINT('',#57067);
#13660=VERTEX_POINT('',#57068);
#13661=VERTEX_POINT('',#57115);
#13662=VERTEX_POINT('',#57116);
#13663=VERTEX_POINT('',#57163);
#13664=VERTEX_POINT('',#57164);
#13665=VERTEX_POINT('',#57211);
#13666=VERTEX_POINT('',#57212);
#13667=VERTEX_POINT('',#57265);
#13668=VERTEX_POINT('',#57266);
#13669=VERTEX_POINT('',#57313);
#13670=VERTEX_POINT('',#57314);
#13671=VERTEX_POINT('',#57361);
#13672=VERTEX_POINT('',#57362);
#13673=VERTEX_POINT('',#57415);
#13674=VERTEX_POINT('',#57416);
#13675=VERTEX_POINT('',#57463);
#13676=VERTEX_POINT('',#57464);
#13677=VERTEX_POINT('',#57511);
#13678=VERTEX_POINT('',#57512);
#13679=VERTEX_POINT('',#57559);
#13680=VERTEX_POINT('',#57560);
#13681=VERTEX_POINT('',#57613);
#13682=VERTEX_POINT('',#57614);
#13683=VERTEX_POINT('',#57661);
#13684=VERTEX_POINT('',#57662);
#13685=VERTEX_POINT('',#57709);
#13686=VERTEX_POINT('',#57710);
#13687=VERTEX_POINT('',#57763);
#13688=VERTEX_POINT('',#57764);
#13689=VERTEX_POINT('',#57811);
#13690=VERTEX_POINT('',#57812);
#13691=VERTEX_POINT('',#57859);
#13692=VERTEX_POINT('',#57860);
#13693=VERTEX_POINT('',#57907);
#13694=VERTEX_POINT('',#57908);
#13695=VERTEX_POINT('',#57961);
#13696=VERTEX_POINT('',#57962);
#13697=VERTEX_POINT('',#58009);
#13698=VERTEX_POINT('',#58010);
#13699=VERTEX_POINT('',#58057);
#13700=VERTEX_POINT('',#58058);
#13701=VERTEX_POINT('',#58111);
#13702=VERTEX_POINT('',#58112);
#13703=VERTEX_POINT('',#58159);
#13704=VERTEX_POINT('',#58160);
#13705=VERTEX_POINT('',#58207);
#13706=VERTEX_POINT('',#58208);
#13707=VERTEX_POINT('',#58255);
#13708=VERTEX_POINT('',#58256);
#13709=VERTEX_POINT('',#58309);
#13710=VERTEX_POINT('',#58310);
#13711=VERTEX_POINT('',#58357);
#13712=VERTEX_POINT('',#58358);
#13713=VERTEX_POINT('',#58405);
#13714=VERTEX_POINT('',#58406);
#13715=VERTEX_POINT('',#58459);
#13716=VERTEX_POINT('',#58460);
#13717=VERTEX_POINT('',#58507);
#13718=VERTEX_POINT('',#58508);
#13719=VERTEX_POINT('',#58555);
#13720=VERTEX_POINT('',#58556);
#13721=VERTEX_POINT('',#58603);
#13722=VERTEX_POINT('',#58604);
#13723=VERTEX_POINT('',#58657);
#13724=VERTEX_POINT('',#58658);
#13725=VERTEX_POINT('',#58705);
#13726=VERTEX_POINT('',#58706);
#13727=VERTEX_POINT('',#58753);
#13728=VERTEX_POINT('',#58754);
#13729=VERTEX_POINT('',#58807);
#13730=VERTEX_POINT('',#58808);
#13731=VERTEX_POINT('',#58855);
#13732=VERTEX_POINT('',#58856);
#13733=VERTEX_POINT('',#58903);
#13734=VERTEX_POINT('',#58904);
#13735=VERTEX_POINT('',#58951);
#13736=VERTEX_POINT('',#58952);
#13737=VERTEX_POINT('',#59005);
#13738=VERTEX_POINT('',#59006);
#13739=VERTEX_POINT('',#59053);
#13740=VERTEX_POINT('',#59054);
#13741=VERTEX_POINT('',#59101);
#13742=VERTEX_POINT('',#59102);
#13743=VERTEX_POINT('',#59155);
#13744=VERTEX_POINT('',#59156);
#13745=VERTEX_POINT('',#59203);
#13746=VERTEX_POINT('',#59204);
#13747=VERTEX_POINT('',#59251);
#13748=VERTEX_POINT('',#59252);
#13749=VERTEX_POINT('',#59299);
#13750=VERTEX_POINT('',#59300);
#13751=VERTEX_POINT('',#59353);
#13752=VERTEX_POINT('',#59354);
#13753=VERTEX_POINT('',#59401);
#13754=VERTEX_POINT('',#59402);
#13755=VERTEX_POINT('',#59404);
#13756=VERTEX_POINT('',#59410);
#13757=VERTEX_POINT('',#59417);
#13758=VERTEX_POINT('',#59418);
#13759=VERTEX_POINT('',#59441);
#13760=VERTEX_POINT('',#59442);
#13761=VERTEX_POINT('',#59466);
#13762=VERTEX_POINT('',#59467);
#13763=VERTEX_POINT('',#59491);
#13764=VERTEX_POINT('',#59492);
#13765=VERTEX_POINT('',#59515);
#13766=VERTEX_POINT('',#59516);
#13767=VERTEX_POINT('',#59539);
#13768=VERTEX_POINT('',#59540);
#13769=VERTEX_POINT('',#59564);
#13770=VERTEX_POINT('',#59565);
#13771=VERTEX_POINT('',#59589);
#13772=VERTEX_POINT('',#59590);
#13773=VERTEX_POINT('',#59613);
#13774=VERTEX_POINT('',#59614);
#13775=VERTEX_POINT('',#59638);
#13776=VERTEX_POINT('',#59639);
#13777=VERTEX_POINT('',#59663);
#13778=VERTEX_POINT('',#59664);
#13779=VERTEX_POINT('',#59687);
#13780=VERTEX_POINT('',#59688);
#13781=VERTEX_POINT('',#59711);
#13782=VERTEX_POINT('',#59712);
#13783=VERTEX_POINT('',#59736);
#13784=VERTEX_POINT('',#59737);
#13785=VERTEX_POINT('',#59761);
#13786=VERTEX_POINT('',#59762);
#13787=VERTEX_POINT('',#59785);
#13788=VERTEX_POINT('',#59786);
#13789=VERTEX_POINT('',#59810);
#13790=VERTEX_POINT('',#59811);
#13791=VERTEX_POINT('',#59835);
#13792=VERTEX_POINT('',#59836);
#13793=VERTEX_POINT('',#59859);
#13794=VERTEX_POINT('',#59860);
#13795=VERTEX_POINT('',#59883);
#13796=VERTEX_POINT('',#59884);
#13797=VERTEX_POINT('',#59908);
#13798=VERTEX_POINT('',#59909);
#13799=VERTEX_POINT('',#59933);
#13800=VERTEX_POINT('',#59934);
#13801=VERTEX_POINT('',#59957);
#13802=VERTEX_POINT('',#59958);
#13803=VERTEX_POINT('',#59982);
#13804=VERTEX_POINT('',#59983);
#13805=VERTEX_POINT('',#60007);
#13806=VERTEX_POINT('',#60008);
#13807=VERTEX_POINT('',#60031);
#13808=VERTEX_POINT('',#60032);
#13809=VERTEX_POINT('',#60055);
#13810=VERTEX_POINT('',#60056);
#13811=VERTEX_POINT('',#60080);
#13812=VERTEX_POINT('',#60081);
#13813=VERTEX_POINT('',#60105);
#13814=VERTEX_POINT('',#60106);
#13815=VERTEX_POINT('',#60129);
#13816=VERTEX_POINT('',#60130);
#13817=VERTEX_POINT('',#60154);
#13818=VERTEX_POINT('',#60155);
#13819=VERTEX_POINT('',#60179);
#13820=VERTEX_POINT('',#60180);
#13821=VERTEX_POINT('',#60203);
#13822=VERTEX_POINT('',#60204);
#13823=VERTEX_POINT('',#60227);
#13824=VERTEX_POINT('',#60228);
#13825=VERTEX_POINT('',#60252);
#13826=VERTEX_POINT('',#60253);
#13827=VERTEX_POINT('',#60277);
#13828=VERTEX_POINT('',#60278);
#13829=VERTEX_POINT('',#60301);
#13830=VERTEX_POINT('',#60302);
#13831=VERTEX_POINT('',#60326);
#13832=VERTEX_POINT('',#60327);
#13833=VERTEX_POINT('',#60351);
#13834=VERTEX_POINT('',#60352);
#13835=VERTEX_POINT('',#60375);
#13836=VERTEX_POINT('',#60376);
#13837=VERTEX_POINT('',#60399);
#13838=VERTEX_POINT('',#60400);
#13839=VERTEX_POINT('',#60424);
#13840=VERTEX_POINT('',#60425);
#13841=VERTEX_POINT('',#60449);
#13842=VERTEX_POINT('',#60450);
#13843=VERTEX_POINT('',#60473);
#13844=VERTEX_POINT('',#60474);
#13845=VERTEX_POINT('',#60498);
#13846=VERTEX_POINT('',#60499);
#13847=VERTEX_POINT('',#60523);
#13848=VERTEX_POINT('',#60524);
#13849=VERTEX_POINT('',#60547);
#13850=VERTEX_POINT('',#60548);
#13851=VERTEX_POINT('',#60571);
#13852=VERTEX_POINT('',#60572);
#13853=VERTEX_POINT('',#60596);
#13854=VERTEX_POINT('',#60597);
#13855=VERTEX_POINT('',#60621);
#13856=VERTEX_POINT('',#60622);
#13857=VERTEX_POINT('',#60645);
#13858=VERTEX_POINT('',#60646);
#13859=VERTEX_POINT('',#60670);
#13860=VERTEX_POINT('',#60671);
#13861=VERTEX_POINT('',#60695);
#13862=VERTEX_POINT('',#60696);
#13863=VERTEX_POINT('',#60719);
#13864=VERTEX_POINT('',#60720);
#13865=VERTEX_POINT('',#60743);
#13866=VERTEX_POINT('',#60744);
#13867=VERTEX_POINT('',#60768);
#13868=VERTEX_POINT('',#60769);
#13869=VERTEX_POINT('',#60793);
#13870=VERTEX_POINT('',#60794);
#13871=VERTEX_POINT('',#60817);
#13872=VERTEX_POINT('',#60818);
#13873=VERTEX_POINT('',#60842);
#13874=VERTEX_POINT('',#60843);
#13875=VERTEX_POINT('',#60867);
#13876=VERTEX_POINT('',#60868);
#13877=VERTEX_POINT('',#60891);
#13878=VERTEX_POINT('',#60892);
#13879=VERTEX_POINT('',#60915);
#13880=VERTEX_POINT('',#60916);
#13881=VERTEX_POINT('',#60940);
#13882=VERTEX_POINT('',#60941);
#13883=VERTEX_POINT('',#60965);
#13884=VERTEX_POINT('',#60966);
#13885=VERTEX_POINT('',#60989);
#13886=VERTEX_POINT('',#60990);
#13887=VERTEX_POINT('',#61014);
#13888=VERTEX_POINT('',#61015);
#13889=VERTEX_POINT('',#61039);
#13890=VERTEX_POINT('',#61040);
#13891=VERTEX_POINT('',#61063);
#13892=VERTEX_POINT('',#61064);
#13893=VERTEX_POINT('',#61087);
#13894=VERTEX_POINT('',#61173);
#13895=VERTEX_POINT('',#61175);
#13896=VERTEX_POINT('',#63027);
#13897=VERTEX_POINT('',#63123);
#13898=VERTEX_POINT('',#63126);
#13899=VERTEX_POINT('',#64985);
#13900=VERTEX_POINT('',#64991);
#13901=VERTEX_POINT('',#64994);
#13902=VERTEX_POINT('',#64995);
#13903=VERTEX_POINT('',#64997);
#13904=VERTEX_POINT('',#64999);
#13905=VERTEX_POINT('',#65003);
#13906=VERTEX_POINT('',#65007);
#13907=VERTEX_POINT('',#65013);
#13908=VERTEX_POINT('',#65014);
#13909=VERTEX_POINT('',#65016);
#13910=VERTEX_POINT('',#65018);
#13911=VERTEX_POINT('',#65022);
#13912=VERTEX_POINT('',#65026);
#13913=VERTEX_POINT('',#65032);
#13914=VERTEX_POINT('',#65033);
#13915=VERTEX_POINT('',#65035);
#13916=VERTEX_POINT('',#65037);
#13917=VERTEX_POINT('',#65041);
#13918=VERTEX_POINT('',#65045);
#13919=VERTEX_POINT('',#65051);
#13920=VERTEX_POINT('',#65052);
#13921=VERTEX_POINT('',#65054);
#13922=VERTEX_POINT('',#65056);
#13923=VERTEX_POINT('',#65060);
#13924=VERTEX_POINT('',#65064);
#13925=VERTEX_POINT('',#65070);
#13926=VERTEX_POINT('',#65071);
#13927=VERTEX_POINT('',#65073);
#13928=VERTEX_POINT('',#65075);
#13929=VERTEX_POINT('',#65079);
#13930=VERTEX_POINT('',#65083);
#13931=VERTEX_POINT('',#65089);
#13932=VERTEX_POINT('',#65090);
#13933=VERTEX_POINT('',#65092);
#13934=VERTEX_POINT('',#65094);
#13935=VERTEX_POINT('',#65098);
#13936=VERTEX_POINT('',#65102);
#13937=VERTEX_POINT('',#65108);
#13938=VERTEX_POINT('',#65109);
#13939=VERTEX_POINT('',#65111);
#13940=VERTEX_POINT('',#65113);
#13941=VERTEX_POINT('',#65117);
#13942=VERTEX_POINT('',#65121);
#13943=VERTEX_POINT('',#65127);
#13944=VERTEX_POINT('',#65128);
#13945=VERTEX_POINT('',#65130);
#13946=VERTEX_POINT('',#65132);
#13947=VERTEX_POINT('',#65136);
#13948=VERTEX_POINT('',#65140);
#13949=VERTEX_POINT('',#65146);
#13950=VERTEX_POINT('',#65147);
#13951=VERTEX_POINT('',#65149);
#13952=VERTEX_POINT('',#65151);
#13953=VERTEX_POINT('',#65155);
#13954=VERTEX_POINT('',#65159);
#13955=VERTEX_POINT('',#65165);
#13956=VERTEX_POINT('',#65166);
#13957=VERTEX_POINT('',#65168);
#13958=VERTEX_POINT('',#65170);
#13959=VERTEX_POINT('',#65174);
#13960=VERTEX_POINT('',#65178);
#13961=VERTEX_POINT('',#65184);
#13962=VERTEX_POINT('',#65185);
#13963=VERTEX_POINT('',#65187);
#13964=VERTEX_POINT('',#65189);
#13965=VERTEX_POINT('',#65193);
#13966=VERTEX_POINT('',#65197);
#13967=VERTEX_POINT('',#65203);
#13968=VERTEX_POINT('',#65204);
#13969=VERTEX_POINT('',#65206);
#13970=VERTEX_POINT('',#65208);
#13971=VERTEX_POINT('',#65212);
#13972=VERTEX_POINT('',#65216);
#13973=VERTEX_POINT('',#65222);
#13974=VERTEX_POINT('',#65223);
#13975=VERTEX_POINT('',#65225);
#13976=VERTEX_POINT('',#65227);
#13977=VERTEX_POINT('',#65231);
#13978=VERTEX_POINT('',#65235);
#13979=VERTEX_POINT('',#65241);
#13980=VERTEX_POINT('',#65242);
#13981=VERTEX_POINT('',#65244);
#13982=VERTEX_POINT('',#65246);
#13983=VERTEX_POINT('',#65250);
#13984=VERTEX_POINT('',#65254);
#13985=VERTEX_POINT('',#65260);
#13986=VERTEX_POINT('',#65261);
#13987=VERTEX_POINT('',#65263);
#13988=VERTEX_POINT('',#65265);
#13989=VERTEX_POINT('',#65269);
#13990=VERTEX_POINT('',#65273);
#13991=VERTEX_POINT('',#65279);
#13992=VERTEX_POINT('',#65280);
#13993=VERTEX_POINT('',#65282);
#13994=VERTEX_POINT('',#65284);
#13995=VERTEX_POINT('',#65288);
#13996=VERTEX_POINT('',#65292);
#13997=VERTEX_POINT('',#65298);
#13998=VERTEX_POINT('',#65299);
#13999=VERTEX_POINT('',#65301);
#14000=VERTEX_POINT('',#65303);
#14001=VERTEX_POINT('',#65307);
#14002=VERTEX_POINT('',#65311);
#14003=VERTEX_POINT('',#65317);
#14004=VERTEX_POINT('',#65318);
#14005=VERTEX_POINT('',#65320);
#14006=VERTEX_POINT('',#65322);
#14007=VERTEX_POINT('',#65326);
#14008=VERTEX_POINT('',#65328);
#14009=VERTEX_POINT('',#65332);
#14010=VERTEX_POINT('',#65336);
#14011=VERTEX_POINT('',#65340);
#14012=VERTEX_POINT('',#65341);
#14013=VERTEX_POINT('',#65343);
#14014=VERTEX_POINT('',#65345);
#14015=VERTEX_POINT('',#65349);
#14016=VERTEX_POINT('',#65353);
#14017=VERTEX_POINT('',#65359);
#14018=VERTEX_POINT('',#65360);
#14019=VERTEX_POINT('',#65362);
#14020=VERTEX_POINT('',#65364);
#14021=VERTEX_POINT('',#65368);
#14022=VERTEX_POINT('',#65372);
#14023=VERTEX_POINT('',#65378);
#14024=VERTEX_POINT('',#65379);
#14025=VERTEX_POINT('',#65381);
#14026=VERTEX_POINT('',#65383);
#14027=VERTEX_POINT('',#65387);
#14028=VERTEX_POINT('',#65391);
#14029=VERTEX_POINT('',#65397);
#14030=VERTEX_POINT('',#65398);
#14031=VERTEX_POINT('',#65400);
#14032=VERTEX_POINT('',#65402);
#14033=VERTEX_POINT('',#65406);
#14034=VERTEX_POINT('',#65410);
#14035=VERTEX_POINT('',#65416);
#14036=VERTEX_POINT('',#65417);
#14037=VERTEX_POINT('',#65419);
#14038=VERTEX_POINT('',#65421);
#14039=VERTEX_POINT('',#65425);
#14040=VERTEX_POINT('',#65429);
#14041=VERTEX_POINT('',#65435);
#14042=VERTEX_POINT('',#65436);
#14043=VERTEX_POINT('',#65438);
#14044=VERTEX_POINT('',#65440);
#14045=VERTEX_POINT('',#65444);
#14046=VERTEX_POINT('',#65448);
#14047=VERTEX_POINT('',#65454);
#14048=VERTEX_POINT('',#65455);
#14049=VERTEX_POINT('',#65457);
#14050=VERTEX_POINT('',#65459);
#14051=VERTEX_POINT('',#65463);
#14052=VERTEX_POINT('',#65467);
#14053=VERTEX_POINT('',#65473);
#14054=VERTEX_POINT('',#65474);
#14055=VERTEX_POINT('',#65476);
#14056=VERTEX_POINT('',#65478);
#14057=VERTEX_POINT('',#65482);
#14058=VERTEX_POINT('',#65486);
#14059=VERTEX_POINT('',#65492);
#14060=VERTEX_POINT('',#65493);
#14061=VERTEX_POINT('',#65495);
#14062=VERTEX_POINT('',#65497);
#14063=VERTEX_POINT('',#65501);
#14064=VERTEX_POINT('',#65505);
#14065=VERTEX_POINT('',#65511);
#14066=VERTEX_POINT('',#65512);
#14067=VERTEX_POINT('',#65514);
#14068=VERTEX_POINT('',#65516);
#14069=VERTEX_POINT('',#65520);
#14070=VERTEX_POINT('',#65524);
#14071=VERTEX_POINT('',#65530);
#14072=VERTEX_POINT('',#65531);
#14073=VERTEX_POINT('',#65533);
#14074=VERTEX_POINT('',#65535);
#14075=VERTEX_POINT('',#65539);
#14076=VERTEX_POINT('',#65543);
#14077=VERTEX_POINT('',#65549);
#14078=VERTEX_POINT('',#65550);
#14079=VERTEX_POINT('',#65552);
#14080=VERTEX_POINT('',#65554);
#14081=VERTEX_POINT('',#65558);
#14082=VERTEX_POINT('',#65562);
#14083=VERTEX_POINT('',#65568);
#14084=VERTEX_POINT('',#65569);
#14085=VERTEX_POINT('',#65571);
#14086=VERTEX_POINT('',#65573);
#14087=VERTEX_POINT('',#65577);
#14088=VERTEX_POINT('',#65581);
#14089=VERTEX_POINT('',#65587);
#14090=VERTEX_POINT('',#65588);
#14091=VERTEX_POINT('',#65590);
#14092=VERTEX_POINT('',#65592);
#14093=VERTEX_POINT('',#65596);
#14094=VERTEX_POINT('',#65600);
#14095=VERTEX_POINT('',#65606);
#14096=VERTEX_POINT('',#65607);
#14097=VERTEX_POINT('',#65609);
#14098=VERTEX_POINT('',#65611);
#14099=VERTEX_POINT('',#65615);
#14100=VERTEX_POINT('',#65619);
#14101=VERTEX_POINT('',#65625);
#14102=VERTEX_POINT('',#65626);
#14103=VERTEX_POINT('',#65628);
#14104=VERTEX_POINT('',#65630);
#14105=VERTEX_POINT('',#65634);
#14106=VERTEX_POINT('',#65638);
#14107=VERTEX_POINT('',#65644);
#14108=VERTEX_POINT('',#65645);
#14109=VERTEX_POINT('',#65647);
#14110=VERTEX_POINT('',#65649);
#14111=VERTEX_POINT('',#65653);
#14112=VERTEX_POINT('',#65657);
#14113=VERTEX_POINT('',#65663);
#14114=VERTEX_POINT('',#65664);
#14115=VERTEX_POINT('',#65666);
#14116=VERTEX_POINT('',#65668);
#14117=VERTEX_POINT('',#65672);
#14118=VERTEX_POINT('',#65676);
#14119=VERTEX_POINT('',#65682);
#14120=VERTEX_POINT('',#65683);
#14121=VERTEX_POINT('',#65687);
#14122=VERTEX_POINT('',#65688);
#14123=VERTEX_POINT('',#65690);
#14124=VERTEX_POINT('',#65692);
#14125=VERTEX_POINT('',#65696);
#14126=VERTEX_POINT('',#65698);
#14127=VERTEX_POINT('',#65702);
#14128=VERTEX_POINT('',#65704);
#14129=VERTEX_POINT('',#65708);
#14130=VERTEX_POINT('',#65710);
#14131=VERTEX_POINT('',#65714);
#14132=VERTEX_POINT('',#65716);
#14133=VERTEX_POINT('',#65724);
#14134=VERTEX_POINT('',#65729);
#14135=VERTEX_POINT('',#65734);
#17394=EDGE_CURVE('',#13613,#13614,#8845,.T.);
#17395=EDGE_CURVE('',#13613,#13615,#2551,.T.);
#17396=EDGE_CURVE('',#13615,#13616,#1635,.T.);
#17397=EDGE_CURVE('',#13616,#13614,#2552,.T.);
#17398=EDGE_CURVE('',#13617,#13618,#8846,.T.);
#17399=EDGE_CURVE('',#13617,#13613,#2553,.T.);
#17400=EDGE_CURVE('',#13614,#13618,#2554,.T.);
#17401=EDGE_CURVE('',#13619,#13620,#8847,.T.);
#17402=EDGE_CURVE('',#13619,#13617,#2555,.T.);
#17403=EDGE_CURVE('',#13618,#13620,#2556,.T.);
#17404=EDGE_CURVE('',#13621,#13622,#8848,.T.);
#17405=EDGE_CURVE('',#13621,#13619,#2557,.T.);
#17406=EDGE_CURVE('',#13620,#13622,#2558,.T.);
#17407=EDGE_CURVE('',#13623,#13624,#8849,.T.);
#17408=EDGE_CURVE('',#13623,#13621,#2559,.T.);
#17409=EDGE_CURVE('',#13622,#13624,#2560,.T.);
#17410=EDGE_CURVE('',#13625,#13626,#8850,.T.);
#17411=EDGE_CURVE('',#13625,#13623,#2561,.T.);
#17412=EDGE_CURVE('',#13624,#13626,#2562,.T.);
#17413=EDGE_CURVE('',#13627,#13628,#8851,.T.);
#17414=EDGE_CURVE('',#13627,#13625,#2563,.T.);
#17415=EDGE_CURVE('',#13626,#13628,#2564,.T.);
#17416=EDGE_CURVE('',#13629,#13630,#8852,.T.);
#17417=EDGE_CURVE('',#13629,#13627,#2565,.T.);
#17418=EDGE_CURVE('',#13628,#13630,#2566,.T.);
#17419=EDGE_CURVE('',#13631,#13632,#8853,.T.);
#17420=EDGE_CURVE('',#13631,#13629,#2567,.T.);
#17421=EDGE_CURVE('',#13630,#13632,#2568,.T.);
#17422=EDGE_CURVE('',#13633,#13634,#8854,.T.);
#17423=EDGE_CURVE('',#13633,#13631,#2569,.T.);
#17424=EDGE_CURVE('',#13632,#13634,#2570,.T.);
#17425=EDGE_CURVE('',#13635,#13636,#8855,.T.);
#17426=EDGE_CURVE('',#13635,#13633,#2571,.T.);
#17427=EDGE_CURVE('',#13634,#13636,#2572,.T.);
#17428=EDGE_CURVE('',#13637,#13638,#8856,.T.);
#17429=EDGE_CURVE('',#13637,#13635,#2573,.T.);
#17430=EDGE_CURVE('',#13636,#13638,#2574,.T.);
#17431=EDGE_CURVE('',#13639,#13640,#8857,.T.);
#17432=EDGE_CURVE('',#13639,#13637,#2575,.T.);
#17433=EDGE_CURVE('',#13638,#13640,#2576,.T.);
#17434=EDGE_CURVE('',#13641,#13642,#8858,.T.);
#17435=EDGE_CURVE('',#13641,#13639,#2577,.T.);
#17436=EDGE_CURVE('',#13640,#13642,#2578,.T.);
#17437=EDGE_CURVE('',#13643,#13644,#8859,.T.);
#17438=EDGE_CURVE('',#13643,#13641,#2579,.T.);
#17439=EDGE_CURVE('',#13642,#13644,#2580,.T.);
#17440=EDGE_CURVE('',#13645,#13646,#8860,.T.);
#17441=EDGE_CURVE('',#13645,#13643,#2581,.T.);
#17442=EDGE_CURVE('',#13644,#13646,#2582,.T.);
#17443=EDGE_CURVE('',#13647,#13648,#8861,.T.);
#17444=EDGE_CURVE('',#13647,#13645,#2583,.T.);
#17445=EDGE_CURVE('',#13646,#13648,#2584,.T.);
#17446=EDGE_CURVE('',#13649,#13650,#8862,.T.);
#17447=EDGE_CURVE('',#13649,#13647,#2585,.T.);
#17448=EDGE_CURVE('',#13648,#13650,#2586,.T.);
#17449=EDGE_CURVE('',#13651,#13652,#8863,.T.);
#17450=EDGE_CURVE('',#13651,#13649,#2587,.T.);
#17451=EDGE_CURVE('',#13650,#13652,#2588,.T.);
#17452=EDGE_CURVE('',#13653,#13654,#8864,.T.);
#17453=EDGE_CURVE('',#13653,#13651,#2589,.T.);
#17454=EDGE_CURVE('',#13652,#13654,#2590,.T.);
#17455=EDGE_CURVE('',#13655,#13656,#8865,.T.);
#17456=EDGE_CURVE('',#13655,#13653,#2591,.T.);
#17457=EDGE_CURVE('',#13654,#13656,#2592,.T.);
#17458=EDGE_CURVE('',#13657,#13658,#8866,.T.);
#17459=EDGE_CURVE('',#13657,#13655,#2593,.T.);
#17460=EDGE_CURVE('',#13656,#13658,#2594,.T.);
#17461=EDGE_CURVE('',#13659,#13660,#8867,.T.);
#17462=EDGE_CURVE('',#13659,#13657,#2595,.T.);
#17463=EDGE_CURVE('',#13658,#13660,#2596,.T.);
#17464=EDGE_CURVE('',#13661,#13662,#8868,.T.);
#17465=EDGE_CURVE('',#13661,#13659,#2597,.T.);
#17466=EDGE_CURVE('',#13660,#13662,#2598,.T.);
#17467=EDGE_CURVE('',#13663,#13664,#8869,.T.);
#17468=EDGE_CURVE('',#13663,#13661,#2599,.T.);
#17469=EDGE_CURVE('',#13662,#13664,#2600,.T.);
#17470=EDGE_CURVE('',#13665,#13666,#8870,.T.);
#17471=EDGE_CURVE('',#13665,#13663,#2601,.T.);
#17472=EDGE_CURVE('',#13664,#13666,#2602,.T.);
#17473=EDGE_CURVE('',#13667,#13668,#8871,.T.);
#17474=EDGE_CURVE('',#13667,#13665,#2603,.T.);
#17475=EDGE_CURVE('',#13666,#13668,#2604,.T.);
#17476=EDGE_CURVE('',#13669,#13670,#8872,.T.);
#17477=EDGE_CURVE('',#13669,#13667,#2605,.T.);
#17478=EDGE_CURVE('',#13668,#13670,#2606,.T.);
#17479=EDGE_CURVE('',#13671,#13672,#8873,.T.);
#17480=EDGE_CURVE('',#13671,#13669,#2607,.T.);
#17481=EDGE_CURVE('',#13670,#13672,#2608,.T.);
#17482=EDGE_CURVE('',#13673,#13674,#8874,.T.);
#17483=EDGE_CURVE('',#13673,#13671,#2609,.T.);
#17484=EDGE_CURVE('',#13672,#13674,#2610,.T.);
#17485=EDGE_CURVE('',#13675,#13676,#8875,.T.);
#17486=EDGE_CURVE('',#13675,#13673,#2611,.T.);
#17487=EDGE_CURVE('',#13674,#13676,#2612,.T.);
#17488=EDGE_CURVE('',#13677,#13678,#8876,.T.);
#17489=EDGE_CURVE('',#13677,#13675,#2613,.T.);
#17490=EDGE_CURVE('',#13676,#13678,#2614,.T.);
#17491=EDGE_CURVE('',#13679,#13680,#8877,.T.);
#17492=EDGE_CURVE('',#13679,#13677,#2615,.T.);
#17493=EDGE_CURVE('',#13678,#13680,#2616,.T.);
#17494=EDGE_CURVE('',#13681,#13682,#8878,.T.);
#17495=EDGE_CURVE('',#13681,#13679,#2617,.T.);
#17496=EDGE_CURVE('',#13680,#13682,#2618,.T.);
#17497=EDGE_CURVE('',#13683,#13684,#8879,.T.);
#17498=EDGE_CURVE('',#13683,#13681,#2619,.T.);
#17499=EDGE_CURVE('',#13682,#13684,#2620,.T.);
#17500=EDGE_CURVE('',#13685,#13686,#8880,.T.);
#17501=EDGE_CURVE('',#13685,#13683,#2621,.T.);
#17502=EDGE_CURVE('',#13684,#13686,#2622,.T.);
#17503=EDGE_CURVE('',#13687,#13688,#8881,.T.);
#17504=EDGE_CURVE('',#13687,#13685,#2623,.T.);
#17505=EDGE_CURVE('',#13686,#13688,#2624,.T.);
#17506=EDGE_CURVE('',#13689,#13690,#8882,.T.);
#17507=EDGE_CURVE('',#13689,#13687,#2625,.T.);
#17508=EDGE_CURVE('',#13688,#13690,#2626,.T.);
#17509=EDGE_CURVE('',#13691,#13692,#8883,.T.);
#17510=EDGE_CURVE('',#13691,#13689,#2627,.T.);
#17511=EDGE_CURVE('',#13690,#13692,#2628,.T.);
#17512=EDGE_CURVE('',#13693,#13694,#8884,.T.);
#17513=EDGE_CURVE('',#13693,#13691,#2629,.T.);
#17514=EDGE_CURVE('',#13692,#13694,#2630,.T.);
#17515=EDGE_CURVE('',#13695,#13696,#8885,.T.);
#17516=EDGE_CURVE('',#13695,#13693,#2631,.T.);
#17517=EDGE_CURVE('',#13694,#13696,#2632,.T.);
#17518=EDGE_CURVE('',#13697,#13698,#8886,.T.);
#17519=EDGE_CURVE('',#13697,#13695,#2633,.T.);
#17520=EDGE_CURVE('',#13696,#13698,#2634,.T.);
#17521=EDGE_CURVE('',#13699,#13700,#8887,.T.);
#17522=EDGE_CURVE('',#13699,#13697,#2635,.T.);
#17523=EDGE_CURVE('',#13698,#13700,#2636,.T.);
#17524=EDGE_CURVE('',#13701,#13702,#8888,.T.);
#17525=EDGE_CURVE('',#13701,#13699,#2637,.T.);
#17526=EDGE_CURVE('',#13700,#13702,#2638,.T.);
#17527=EDGE_CURVE('',#13703,#13704,#8889,.T.);
#17528=EDGE_CURVE('',#13703,#13701,#2639,.T.);
#17529=EDGE_CURVE('',#13702,#13704,#2640,.T.);
#17530=EDGE_CURVE('',#13705,#13706,#8890,.T.);
#17531=EDGE_CURVE('',#13705,#13703,#2641,.T.);
#17532=EDGE_CURVE('',#13704,#13706,#2642,.T.);
#17533=EDGE_CURVE('',#13707,#13708,#8891,.T.);
#17534=EDGE_CURVE('',#13707,#13705,#2643,.T.);
#17535=EDGE_CURVE('',#13706,#13708,#2644,.T.);
#17536=EDGE_CURVE('',#13709,#13710,#8892,.T.);
#17537=EDGE_CURVE('',#13709,#13707,#2645,.T.);
#17538=EDGE_CURVE('',#13708,#13710,#2646,.T.);
#17539=EDGE_CURVE('',#13711,#13712,#8893,.T.);
#17540=EDGE_CURVE('',#13711,#13709,#2647,.T.);
#17541=EDGE_CURVE('',#13710,#13712,#2648,.T.);
#17542=EDGE_CURVE('',#13713,#13714,#8894,.T.);
#17543=EDGE_CURVE('',#13713,#13711,#2649,.T.);
#17544=EDGE_CURVE('',#13712,#13714,#2650,.T.);
#17545=EDGE_CURVE('',#13715,#13716,#8895,.T.);
#17546=EDGE_CURVE('',#13715,#13713,#2651,.T.);
#17547=EDGE_CURVE('',#13714,#13716,#2652,.T.);
#17548=EDGE_CURVE('',#13717,#13718,#8896,.T.);
#17549=EDGE_CURVE('',#13717,#13715,#2653,.T.);
#17550=EDGE_CURVE('',#13716,#13718,#2654,.T.);
#17551=EDGE_CURVE('',#13719,#13720,#8897,.T.);
#17552=EDGE_CURVE('',#13719,#13717,#2655,.T.);
#17553=EDGE_CURVE('',#13718,#13720,#2656,.T.);
#17554=EDGE_CURVE('',#13721,#13722,#8898,.T.);
#17555=EDGE_CURVE('',#13721,#13719,#2657,.T.);
#17556=EDGE_CURVE('',#13720,#13722,#2658,.T.);
#17557=EDGE_CURVE('',#13723,#13724,#8899,.T.);
#17558=EDGE_CURVE('',#13723,#13721,#2659,.T.);
#17559=EDGE_CURVE('',#13722,#13724,#2660,.T.);
#17560=EDGE_CURVE('',#13725,#13726,#8900,.T.);
#17561=EDGE_CURVE('',#13725,#13723,#2661,.T.);
#17562=EDGE_CURVE('',#13724,#13726,#2662,.T.);
#17563=EDGE_CURVE('',#13727,#13728,#8901,.T.);
#17564=EDGE_CURVE('',#13727,#13725,#2663,.T.);
#17565=EDGE_CURVE('',#13726,#13728,#2664,.T.);
#17566=EDGE_CURVE('',#13729,#13730,#8902,.T.);
#17567=EDGE_CURVE('',#13729,#13727,#2665,.T.);
#17568=EDGE_CURVE('',#13728,#13730,#2666,.T.);
#17569=EDGE_CURVE('',#13731,#13732,#8903,.T.);
#17570=EDGE_CURVE('',#13731,#13729,#2667,.T.);
#17571=EDGE_CURVE('',#13730,#13732,#2668,.T.);
#17572=EDGE_CURVE('',#13733,#13734,#8904,.T.);
#17573=EDGE_CURVE('',#13733,#13731,#2669,.T.);
#17574=EDGE_CURVE('',#13732,#13734,#2670,.T.);
#17575=EDGE_CURVE('',#13735,#13736,#8905,.T.);
#17576=EDGE_CURVE('',#13735,#13733,#2671,.T.);
#17577=EDGE_CURVE('',#13734,#13736,#2672,.T.);
#17578=EDGE_CURVE('',#13737,#13738,#8906,.T.);
#17579=EDGE_CURVE('',#13737,#13735,#2673,.T.);
#17580=EDGE_CURVE('',#13736,#13738,#2674,.T.);
#17581=EDGE_CURVE('',#13739,#13740,#8907,.T.);
#17582=EDGE_CURVE('',#13739,#13737,#2675,.T.);
#17583=EDGE_CURVE('',#13738,#13740,#2676,.T.);
#17584=EDGE_CURVE('',#13741,#13742,#8908,.T.);
#17585=EDGE_CURVE('',#13741,#13739,#2677,.T.);
#17586=EDGE_CURVE('',#13740,#13742,#2678,.T.);
#17587=EDGE_CURVE('',#13743,#13744,#8909,.T.);
#17588=EDGE_CURVE('',#13743,#13741,#2679,.T.);
#17589=EDGE_CURVE('',#13742,#13744,#2680,.T.);
#17590=EDGE_CURVE('',#13745,#13746,#8910,.T.);
#17591=EDGE_CURVE('',#13745,#13743,#2681,.T.);
#17592=EDGE_CURVE('',#13744,#13746,#2682,.T.);
#17593=EDGE_CURVE('',#13747,#13748,#8911,.T.);
#17594=EDGE_CURVE('',#13747,#13745,#2683,.T.);
#17595=EDGE_CURVE('',#13746,#13748,#2684,.T.);
#17596=EDGE_CURVE('',#13749,#13750,#8912,.T.);
#17597=EDGE_CURVE('',#13749,#13747,#2685,.T.);
#17598=EDGE_CURVE('',#13748,#13750,#2686,.T.);
#17599=EDGE_CURVE('',#13751,#13752,#8913,.T.);
#17600=EDGE_CURVE('',#13751,#13749,#2687,.T.);
#17601=EDGE_CURVE('',#13750,#13752,#2688,.T.);
#17602=EDGE_CURVE('',#13753,#13754,#8914,.T.);
#17603=EDGE_CURVE('',#13753,#13755,#2689,.T.);
#17604=EDGE_CURVE('',#13756,#13755,#1636,.T.);
#17605=EDGE_CURVE('',#13754,#13756,#2690,.T.);
#17606=EDGE_CURVE('',#13757,#13758,#8915,.T.);
#17607=EDGE_CURVE('',#13757,#13753,#2691,.T.);
#17608=EDGE_CURVE('',#13758,#13754,#2692,.T.);
#17609=EDGE_CURVE('',#13759,#13760,#8916,.T.);
#17610=EDGE_CURVE('',#13759,#13757,#2693,.T.);
#17611=EDGE_CURVE('',#13760,#13758,#2694,.T.);
#17612=EDGE_CURVE('',#13761,#13762,#8917,.T.);
#17613=EDGE_CURVE('',#13761,#13759,#2695,.T.);
#17614=EDGE_CURVE('',#13762,#13760,#2696,.T.);
#17615=EDGE_CURVE('',#13763,#13764,#8918,.T.);
#17616=EDGE_CURVE('',#13763,#13761,#2697,.T.);
#17617=EDGE_CURVE('',#13764,#13762,#2698,.T.);
#17618=EDGE_CURVE('',#13765,#13766,#8919,.T.);
#17619=EDGE_CURVE('',#13765,#13763,#2699,.T.);
#17620=EDGE_CURVE('',#13766,#13764,#2700,.T.);
#17621=EDGE_CURVE('',#13767,#13768,#8920,.T.);
#17622=EDGE_CURVE('',#13767,#13765,#2701,.T.);
#17623=EDGE_CURVE('',#13768,#13766,#2702,.T.);
#17624=EDGE_CURVE('',#13769,#13770,#8921,.T.);
#17625=EDGE_CURVE('',#13769,#13767,#2703,.T.);
#17626=EDGE_CURVE('',#13770,#13768,#2704,.T.);
#17627=EDGE_CURVE('',#13771,#13772,#8922,.T.);
#17628=EDGE_CURVE('',#13771,#13769,#2705,.T.);
#17629=EDGE_CURVE('',#13772,#13770,#2706,.T.);
#17630=EDGE_CURVE('',#13773,#13774,#8923,.T.);
#17631=EDGE_CURVE('',#13773,#13771,#2707,.T.);
#17632=EDGE_CURVE('',#13774,#13772,#2708,.T.);
#17633=EDGE_CURVE('',#13775,#13776,#8924,.T.);
#17634=EDGE_CURVE('',#13775,#13773,#2709,.T.);
#17635=EDGE_CURVE('',#13776,#13774,#2710,.T.);
#17636=EDGE_CURVE('',#13777,#13778,#8925,.T.);
#17637=EDGE_CURVE('',#13777,#13775,#2711,.T.);
#17638=EDGE_CURVE('',#13778,#13776,#2712,.T.);
#17639=EDGE_CURVE('',#13779,#13780,#8926,.T.);
#17640=EDGE_CURVE('',#13779,#13777,#2713,.T.);
#17641=EDGE_CURVE('',#13780,#13778,#2714,.T.);
#17642=EDGE_CURVE('',#13781,#13782,#8927,.T.);
#17643=EDGE_CURVE('',#13781,#13779,#2715,.T.);
#17644=EDGE_CURVE('',#13782,#13780,#2716,.T.);
#17645=EDGE_CURVE('',#13783,#13784,#8928,.T.);
#17646=EDGE_CURVE('',#13783,#13781,#2717,.T.);
#17647=EDGE_CURVE('',#13784,#13782,#2718,.T.);
#17648=EDGE_CURVE('',#13785,#13786,#8929,.T.);
#17649=EDGE_CURVE('',#13785,#13783,#2719,.T.);
#17650=EDGE_CURVE('',#13786,#13784,#2720,.T.);
#17651=EDGE_CURVE('',#13787,#13788,#8930,.T.);
#17652=EDGE_CURVE('',#13787,#13785,#2721,.T.);
#17653=EDGE_CURVE('',#13788,#13786,#2722,.T.);
#17654=EDGE_CURVE('',#13789,#13790,#8931,.T.);
#17655=EDGE_CURVE('',#13789,#13787,#2723,.T.);
#17656=EDGE_CURVE('',#13790,#13788,#2724,.T.);
#17657=EDGE_CURVE('',#13791,#13792,#8932,.T.);
#17658=EDGE_CURVE('',#13791,#13789,#2725,.T.);
#17659=EDGE_CURVE('',#13792,#13790,#2726,.T.);
#17660=EDGE_CURVE('',#13793,#13794,#8933,.T.);
#17661=EDGE_CURVE('',#13793,#13791,#2727,.T.);
#17662=EDGE_CURVE('',#13794,#13792,#2728,.T.);
#17663=EDGE_CURVE('',#13795,#13796,#8934,.T.);
#17664=EDGE_CURVE('',#13795,#13793,#2729,.T.);
#17665=EDGE_CURVE('',#13796,#13794,#2730,.T.);
#17666=EDGE_CURVE('',#13797,#13798,#8935,.T.);
#17667=EDGE_CURVE('',#13797,#13795,#2731,.T.);
#17668=EDGE_CURVE('',#13798,#13796,#2732,.T.);
#17669=EDGE_CURVE('',#13799,#13800,#8936,.T.);
#17670=EDGE_CURVE('',#13799,#13797,#2733,.T.);
#17671=EDGE_CURVE('',#13800,#13798,#2734,.T.);
#17672=EDGE_CURVE('',#13801,#13802,#8937,.T.);
#17673=EDGE_CURVE('',#13801,#13799,#2735,.T.);
#17674=EDGE_CURVE('',#13802,#13800,#2736,.T.);
#17675=EDGE_CURVE('',#13803,#13804,#8938,.T.);
#17676=EDGE_CURVE('',#13803,#13801,#2737,.T.);
#17677=EDGE_CURVE('',#13804,#13802,#2738,.T.);
#17678=EDGE_CURVE('',#13805,#13806,#8939,.T.);
#17679=EDGE_CURVE('',#13805,#13803,#2739,.T.);
#17680=EDGE_CURVE('',#13806,#13804,#2740,.T.);
#17681=EDGE_CURVE('',#13807,#13808,#8940,.T.);
#17682=EDGE_CURVE('',#13807,#13805,#2741,.T.);
#17683=EDGE_CURVE('',#13808,#13806,#2742,.T.);
#17684=EDGE_CURVE('',#13809,#13810,#8941,.T.);
#17685=EDGE_CURVE('',#13809,#13807,#2743,.T.);
#17686=EDGE_CURVE('',#13810,#13808,#2744,.T.);
#17687=EDGE_CURVE('',#13811,#13812,#8942,.T.);
#17688=EDGE_CURVE('',#13811,#13809,#2745,.T.);
#17689=EDGE_CURVE('',#13812,#13810,#2746,.T.);
#17690=EDGE_CURVE('',#13813,#13814,#8943,.T.);
#17691=EDGE_CURVE('',#13813,#13811,#2747,.T.);
#17692=EDGE_CURVE('',#13814,#13812,#2748,.T.);
#17693=EDGE_CURVE('',#13815,#13816,#8944,.T.);
#17694=EDGE_CURVE('',#13815,#13813,#2749,.T.);
#17695=EDGE_CURVE('',#13816,#13814,#2750,.T.);
#17696=EDGE_CURVE('',#13817,#13818,#8945,.T.);
#17697=EDGE_CURVE('',#13817,#13815,#2751,.T.);
#17698=EDGE_CURVE('',#13818,#13816,#2752,.T.);
#17699=EDGE_CURVE('',#13819,#13820,#8946,.T.);
#17700=EDGE_CURVE('',#13819,#13817,#2753,.T.);
#17701=EDGE_CURVE('',#13820,#13818,#2754,.T.);
#17702=EDGE_CURVE('',#13821,#13822,#8947,.T.);
#17703=EDGE_CURVE('',#13821,#13819,#2755,.T.);
#17704=EDGE_CURVE('',#13822,#13820,#2756,.T.);
#17705=EDGE_CURVE('',#13823,#13824,#8948,.T.);
#17706=EDGE_CURVE('',#13823,#13821,#2757,.T.);
#17707=EDGE_CURVE('',#13824,#13822,#2758,.T.);
#17708=EDGE_CURVE('',#13825,#13826,#8949,.T.);
#17709=EDGE_CURVE('',#13825,#13823,#2759,.T.);
#17710=EDGE_CURVE('',#13826,#13824,#2760,.T.);
#17711=EDGE_CURVE('',#13827,#13828,#8950,.T.);
#17712=EDGE_CURVE('',#13827,#13825,#2761,.T.);
#17713=EDGE_CURVE('',#13828,#13826,#2762,.T.);
#17714=EDGE_CURVE('',#13829,#13830,#8951,.T.);
#17715=EDGE_CURVE('',#13829,#13827,#2763,.T.);
#17716=EDGE_CURVE('',#13830,#13828,#2764,.T.);
#17717=EDGE_CURVE('',#13831,#13832,#8952,.T.);
#17718=EDGE_CURVE('',#13831,#13829,#2765,.T.);
#17719=EDGE_CURVE('',#13832,#13830,#2766,.T.);
#17720=EDGE_CURVE('',#13833,#13834,#8953,.T.);
#17721=EDGE_CURVE('',#13833,#13831,#2767,.T.);
#17722=EDGE_CURVE('',#13834,#13832,#2768,.T.);
#17723=EDGE_CURVE('',#13835,#13836,#8954,.T.);
#17724=EDGE_CURVE('',#13835,#13833,#2769,.T.);
#17725=EDGE_CURVE('',#13836,#13834,#2770,.T.);
#17726=EDGE_CURVE('',#13837,#13838,#8955,.T.);
#17727=EDGE_CURVE('',#13837,#13835,#2771,.T.);
#17728=EDGE_CURVE('',#13838,#13836,#2772,.T.);
#17729=EDGE_CURVE('',#13839,#13840,#8956,.T.);
#17730=EDGE_CURVE('',#13839,#13837,#2773,.T.);
#17731=EDGE_CURVE('',#13840,#13838,#2774,.T.);
#17732=EDGE_CURVE('',#13841,#13842,#8957,.T.);
#17733=EDGE_CURVE('',#13841,#13839,#2775,.T.);
#17734=EDGE_CURVE('',#13842,#13840,#2776,.T.);
#17735=EDGE_CURVE('',#13843,#13844,#8958,.T.);
#17736=EDGE_CURVE('',#13843,#13841,#2777,.T.);
#17737=EDGE_CURVE('',#13844,#13842,#2778,.T.);
#17738=EDGE_CURVE('',#13845,#13846,#8959,.T.);
#17739=EDGE_CURVE('',#13845,#13843,#2779,.T.);
#17740=EDGE_CURVE('',#13846,#13844,#2780,.T.);
#17741=EDGE_CURVE('',#13847,#13848,#8960,.T.);
#17742=EDGE_CURVE('',#13847,#13845,#2781,.T.);
#17743=EDGE_CURVE('',#13848,#13846,#2782,.T.);
#17744=EDGE_CURVE('',#13849,#13850,#8961,.T.);
#17745=EDGE_CURVE('',#13849,#13847,#2783,.T.);
#17746=EDGE_CURVE('',#13850,#13848,#2784,.T.);
#17747=EDGE_CURVE('',#13851,#13852,#8962,.T.);
#17748=EDGE_CURVE('',#13851,#13849,#2785,.T.);
#17749=EDGE_CURVE('',#13852,#13850,#2786,.T.);
#17750=EDGE_CURVE('',#13853,#13854,#8963,.T.);
#17751=EDGE_CURVE('',#13853,#13851,#2787,.T.);
#17752=EDGE_CURVE('',#13854,#13852,#2788,.T.);
#17753=EDGE_CURVE('',#13855,#13856,#8964,.T.);
#17754=EDGE_CURVE('',#13855,#13853,#2789,.T.);
#17755=EDGE_CURVE('',#13856,#13854,#2790,.T.);
#17756=EDGE_CURVE('',#13857,#13858,#8965,.T.);
#17757=EDGE_CURVE('',#13857,#13855,#2791,.T.);
#17758=EDGE_CURVE('',#13858,#13856,#2792,.T.);
#17759=EDGE_CURVE('',#13859,#13860,#8966,.T.);
#17760=EDGE_CURVE('',#13859,#13857,#2793,.T.);
#17761=EDGE_CURVE('',#13860,#13858,#2794,.T.);
#17762=EDGE_CURVE('',#13861,#13862,#8967,.T.);
#17763=EDGE_CURVE('',#13861,#13859,#2795,.T.);
#17764=EDGE_CURVE('',#13862,#13860,#2796,.T.);
#17765=EDGE_CURVE('',#13863,#13864,#8968,.T.);
#17766=EDGE_CURVE('',#13863,#13861,#2797,.T.);
#17767=EDGE_CURVE('',#13864,#13862,#2798,.T.);
#17768=EDGE_CURVE('',#13865,#13866,#8969,.T.);
#17769=EDGE_CURVE('',#13865,#13863,#2799,.T.);
#17770=EDGE_CURVE('',#13866,#13864,#2800,.T.);
#17771=EDGE_CURVE('',#13867,#13868,#8970,.T.);
#17772=EDGE_CURVE('',#13867,#13865,#2801,.T.);
#17773=EDGE_CURVE('',#13868,#13866,#2802,.T.);
#17774=EDGE_CURVE('',#13869,#13870,#8971,.T.);
#17775=EDGE_CURVE('',#13869,#13867,#2803,.T.);
#17776=EDGE_CURVE('',#13870,#13868,#2804,.T.);
#17777=EDGE_CURVE('',#13871,#13872,#8972,.T.);
#17778=EDGE_CURVE('',#13871,#13869,#2805,.T.);
#17779=EDGE_CURVE('',#13872,#13870,#2806,.T.);
#17780=EDGE_CURVE('',#13873,#13874,#8973,.T.);
#17781=EDGE_CURVE('',#13873,#13871,#2807,.T.);
#17782=EDGE_CURVE('',#13874,#13872,#2808,.T.);
#17783=EDGE_CURVE('',#13875,#13876,#8974,.T.);
#17784=EDGE_CURVE('',#13875,#13873,#2809,.T.);
#17785=EDGE_CURVE('',#13876,#13874,#2810,.T.);
#17786=EDGE_CURVE('',#13877,#13878,#8975,.T.);
#17787=EDGE_CURVE('',#13877,#13875,#2811,.T.);
#17788=EDGE_CURVE('',#13878,#13876,#2812,.T.);
#17789=EDGE_CURVE('',#13879,#13880,#8976,.T.);
#17790=EDGE_CURVE('',#13879,#13877,#2813,.T.);
#17791=EDGE_CURVE('',#13880,#13878,#2814,.T.);
#17792=EDGE_CURVE('',#13881,#13882,#8977,.T.);
#17793=EDGE_CURVE('',#13881,#13879,#2815,.T.);
#17794=EDGE_CURVE('',#13882,#13880,#2816,.T.);
#17795=EDGE_CURVE('',#13883,#13884,#8978,.T.);
#17796=EDGE_CURVE('',#13883,#13881,#2817,.T.);
#17797=EDGE_CURVE('',#13884,#13882,#2818,.T.);
#17798=EDGE_CURVE('',#13885,#13886,#8979,.T.);
#17799=EDGE_CURVE('',#13885,#13883,#2819,.T.);
#17800=EDGE_CURVE('',#13886,#13884,#2820,.T.);
#17801=EDGE_CURVE('',#13887,#13888,#8980,.T.);
#17802=EDGE_CURVE('',#13887,#13885,#2821,.T.);
#17803=EDGE_CURVE('',#13888,#13886,#2822,.T.);
#17804=EDGE_CURVE('',#13889,#13890,#8981,.T.);
#17805=EDGE_CURVE('',#13889,#13887,#2823,.T.);
#17806=EDGE_CURVE('',#13890,#13888,#2824,.T.);
#17807=EDGE_CURVE('',#13891,#13892,#8982,.T.);
#17808=EDGE_CURVE('',#13891,#13889,#2825,.T.);
#17809=EDGE_CURVE('',#13892,#13890,#2826,.T.);
#17810=EDGE_CURVE('',#13755,#13893,#2827,.T.);
#17811=EDGE_CURVE('',#13894,#13893,#1637,.T.);
#17812=EDGE_CURVE('',#13895,#13894,#1638,.T.);
#17813=EDGE_CURVE('',#13895,#13756,#2828,.T.);
#17814=EDGE_CURVE('',#13752,#13895,#2829,.T.);
#17815=EDGE_CURVE('',#13896,#13616,#2830,.T.);
#17816=EDGE_CURVE('',#13896,#13892,#2831,.T.);
#17817=EDGE_CURVE('',#13616,#13897,#1639,.T.);
#17818=EDGE_CURVE('',#13897,#13615,#1640,.T.);
#17819=EDGE_CURVE('',#13615,#13898,#2832,.T.);
#17820=EDGE_CURVE('',#13898,#13896,#1641,.T.);
#17821=EDGE_CURVE('',#13898,#13891,#2833,.T.);
#17822=EDGE_CURVE('',#13893,#13751,#2834,.T.);
#17823=EDGE_CURVE('',#13894,#13899,#1642,.T.);
#17824=EDGE_CURVE('',#13899,#13899,#1643,.T.);
#17825=EDGE_CURVE('',#13893,#13895,#1644,.T.);
#17826=EDGE_CURVE('',#13900,#13900,#1645,.T.);
#17827=EDGE_CURVE('',#13901,#13902,#8983,.T.);
#17828=EDGE_CURVE('',#13901,#13903,#8984,.T.);
#17829=EDGE_CURVE('',#13904,#13903,#8985,.T.);
#17830=EDGE_CURVE('',#13902,#13904,#8986,.T.);
#17831=EDGE_CURVE('',#13902,#13905,#1646,.T.);
#17832=EDGE_CURVE('',#13904,#13905,#8987,.T.);
#17833=EDGE_CURVE('',#13905,#13906,#8988,.T.);
#17834=EDGE_CURVE('',#13903,#13906,#8989,.T.);
#17835=EDGE_CURVE('',#13906,#13901,#1647,.T.);
#17836=EDGE_CURVE('',#13907,#13908,#8990,.T.);
#17837=EDGE_CURVE('',#13907,#13909,#8991,.T.);
#17838=EDGE_CURVE('',#13910,#13909,#8992,.T.);
#17839=EDGE_CURVE('',#13908,#13910,#8993,.T.);
#17840=EDGE_CURVE('',#13908,#13911,#1648,.T.);
#17841=EDGE_CURVE('',#13910,#13911,#8994,.T.);
#17842=EDGE_CURVE('',#13911,#13912,#8995,.T.);
#17843=EDGE_CURVE('',#13909,#13912,#8996,.T.);
#17844=EDGE_CURVE('',#13912,#13907,#1649,.T.);
#17845=EDGE_CURVE('',#13913,#13914,#8997,.T.);
#17846=EDGE_CURVE('',#13913,#13915,#8998,.T.);
#17847=EDGE_CURVE('',#13916,#13915,#8999,.T.);
#17848=EDGE_CURVE('',#13914,#13916,#9000,.T.);
#17849=EDGE_CURVE('',#13914,#13917,#1650,.T.);
#17850=EDGE_CURVE('',#13916,#13917,#9001,.T.);
#17851=EDGE_CURVE('',#13917,#13918,#9002,.T.);
#17852=EDGE_CURVE('',#13915,#13918,#9003,.T.);
#17853=EDGE_CURVE('',#13918,#13913,#1651,.T.);
#17854=EDGE_CURVE('',#13919,#13920,#9004,.T.);
#17855=EDGE_CURVE('',#13919,#13921,#9005,.T.);
#17856=EDGE_CURVE('',#13922,#13921,#9006,.T.);
#17857=EDGE_CURVE('',#13920,#13922,#9007,.T.);
#17858=EDGE_CURVE('',#13920,#13923,#1652,.T.);
#17859=EDGE_CURVE('',#13922,#13923,#9008,.T.);
#17860=EDGE_CURVE('',#13923,#13924,#9009,.T.);
#17861=EDGE_CURVE('',#13921,#13924,#9010,.T.);
#17862=EDGE_CURVE('',#13924,#13919,#1653,.T.);
#17863=EDGE_CURVE('',#13925,#13926,#9011,.T.);
#17864=EDGE_CURVE('',#13925,#13927,#9012,.T.);
#17865=EDGE_CURVE('',#13928,#13927,#9013,.T.);
#17866=EDGE_CURVE('',#13926,#13928,#9014,.T.);
#17867=EDGE_CURVE('',#13926,#13929,#1654,.T.);
#17868=EDGE_CURVE('',#13928,#13929,#9015,.T.);
#17869=EDGE_CURVE('',#13929,#13930,#9016,.T.);
#17870=EDGE_CURVE('',#13927,#13930,#9017,.T.);
#17871=EDGE_CURVE('',#13930,#13925,#1655,.T.);
#17872=EDGE_CURVE('',#13931,#13932,#9018,.T.);
#17873=EDGE_CURVE('',#13931,#13933,#9019,.T.);
#17874=EDGE_CURVE('',#13934,#13933,#9020,.T.);
#17875=EDGE_CURVE('',#13932,#13934,#9021,.T.);
#17876=EDGE_CURVE('',#13932,#13935,#1656,.T.);
#17877=EDGE_CURVE('',#13934,#13935,#9022,.T.);
#17878=EDGE_CURVE('',#13935,#13936,#9023,.T.);
#17879=EDGE_CURVE('',#13933,#13936,#9024,.T.);
#17880=EDGE_CURVE('',#13936,#13931,#1657,.T.);
#17881=EDGE_CURVE('',#13937,#13938,#9025,.T.);
#17882=EDGE_CURVE('',#13937,#13939,#9026,.T.);
#17883=EDGE_CURVE('',#13940,#13939,#9027,.T.);
#17884=EDGE_CURVE('',#13938,#13940,#9028,.T.);
#17885=EDGE_CURVE('',#13938,#13941,#1658,.T.);
#17886=EDGE_CURVE('',#13940,#13941,#9029,.T.);
#17887=EDGE_CURVE('',#13941,#13942,#9030,.T.);
#17888=EDGE_CURVE('',#13939,#13942,#9031,.T.);
#17889=EDGE_CURVE('',#13942,#13937,#1659,.T.);
#17890=EDGE_CURVE('',#13943,#13944,#9032,.T.);
#17891=EDGE_CURVE('',#13943,#13945,#9033,.T.);
#17892=EDGE_CURVE('',#13946,#13945,#9034,.T.);
#17893=EDGE_CURVE('',#13944,#13946,#9035,.T.);
#17894=EDGE_CURVE('',#13944,#13947,#1660,.T.);
#17895=EDGE_CURVE('',#13946,#13947,#9036,.T.);
#17896=EDGE_CURVE('',#13947,#13948,#9037,.T.);
#17897=EDGE_CURVE('',#13945,#13948,#9038,.T.);
#17898=EDGE_CURVE('',#13948,#13943,#1661,.T.);
#17899=EDGE_CURVE('',#13949,#13950,#9039,.T.);
#17900=EDGE_CURVE('',#13949,#13951,#9040,.T.);
#17901=EDGE_CURVE('',#13952,#13951,#9041,.T.);
#17902=EDGE_CURVE('',#13950,#13952,#9042,.T.);
#17903=EDGE_CURVE('',#13950,#13953,#1662,.T.);
#17904=EDGE_CURVE('',#13952,#13953,#9043,.T.);
#17905=EDGE_CURVE('',#13953,#13954,#9044,.T.);
#17906=EDGE_CURVE('',#13951,#13954,#9045,.T.);
#17907=EDGE_CURVE('',#13954,#13949,#1663,.T.);
#17908=EDGE_CURVE('',#13955,#13956,#9046,.T.);
#17909=EDGE_CURVE('',#13955,#13957,#9047,.T.);
#17910=EDGE_CURVE('',#13958,#13957,#9048,.T.);
#17911=EDGE_CURVE('',#13956,#13958,#9049,.T.);
#17912=EDGE_CURVE('',#13956,#13959,#1664,.T.);
#17913=EDGE_CURVE('',#13958,#13959,#9050,.T.);
#17914=EDGE_CURVE('',#13959,#13960,#9051,.T.);
#17915=EDGE_CURVE('',#13957,#13960,#9052,.T.);
#17916=EDGE_CURVE('',#13960,#13955,#1665,.T.);
#17917=EDGE_CURVE('',#13961,#13962,#9053,.T.);
#17918=EDGE_CURVE('',#13961,#13963,#9054,.T.);
#17919=EDGE_CURVE('',#13964,#13963,#9055,.T.);
#17920=EDGE_CURVE('',#13962,#13964,#9056,.T.);
#17921=EDGE_CURVE('',#13962,#13965,#1666,.T.);
#17922=EDGE_CURVE('',#13964,#13965,#9057,.T.);
#17923=EDGE_CURVE('',#13965,#13966,#9058,.T.);
#17924=EDGE_CURVE('',#13963,#13966,#9059,.T.);
#17925=EDGE_CURVE('',#13966,#13961,#1667,.T.);
#17926=EDGE_CURVE('',#13967,#13968,#9060,.T.);
#17927=EDGE_CURVE('',#13967,#13969,#9061,.T.);
#17928=EDGE_CURVE('',#13970,#13969,#9062,.T.);
#17929=EDGE_CURVE('',#13968,#13970,#9063,.T.);
#17930=EDGE_CURVE('',#13968,#13971,#1668,.T.);
#17931=EDGE_CURVE('',#13970,#13971,#9064,.T.);
#17932=EDGE_CURVE('',#13971,#13972,#9065,.T.);
#17933=EDGE_CURVE('',#13969,#13972,#9066,.T.);
#17934=EDGE_CURVE('',#13972,#13967,#1669,.T.);
#17935=EDGE_CURVE('',#13973,#13974,#9067,.T.);
#17936=EDGE_CURVE('',#13973,#13975,#9068,.T.);
#17937=EDGE_CURVE('',#13976,#13975,#9069,.T.);
#17938=EDGE_CURVE('',#13974,#13976,#9070,.T.);
#17939=EDGE_CURVE('',#13974,#13977,#1670,.T.);
#17940=EDGE_CURVE('',#13976,#13977,#9071,.T.);
#17941=EDGE_CURVE('',#13977,#13978,#9072,.T.);
#17942=EDGE_CURVE('',#13975,#13978,#9073,.T.);
#17943=EDGE_CURVE('',#13978,#13973,#1671,.T.);
#17944=EDGE_CURVE('',#13979,#13980,#9074,.T.);
#17945=EDGE_CURVE('',#13979,#13981,#9075,.T.);
#17946=EDGE_CURVE('',#13982,#13981,#9076,.T.);
#17947=EDGE_CURVE('',#13980,#13982,#9077,.T.);
#17948=EDGE_CURVE('',#13980,#13983,#1672,.T.);
#17949=EDGE_CURVE('',#13982,#13983,#9078,.T.);
#17950=EDGE_CURVE('',#13983,#13984,#9079,.T.);
#17951=EDGE_CURVE('',#13981,#13984,#9080,.T.);
#17952=EDGE_CURVE('',#13984,#13979,#1673,.T.);
#17953=EDGE_CURVE('',#13985,#13986,#9081,.T.);
#17954=EDGE_CURVE('',#13985,#13987,#9082,.T.);
#17955=EDGE_CURVE('',#13988,#13987,#9083,.T.);
#17956=EDGE_CURVE('',#13986,#13988,#9084,.T.);
#17957=EDGE_CURVE('',#13986,#13989,#1674,.T.);
#17958=EDGE_CURVE('',#13988,#13989,#9085,.T.);
#17959=EDGE_CURVE('',#13989,#13990,#9086,.T.);
#17960=EDGE_CURVE('',#13987,#13990,#9087,.T.);
#17961=EDGE_CURVE('',#13990,#13985,#1675,.T.);
#17962=EDGE_CURVE('',#13991,#13992,#9088,.T.);
#17963=EDGE_CURVE('',#13991,#13993,#9089,.T.);
#17964=EDGE_CURVE('',#13994,#13993,#9090,.T.);
#17965=EDGE_CURVE('',#13992,#13994,#9091,.T.);
#17966=EDGE_CURVE('',#13992,#13995,#1676,.T.);
#17967=EDGE_CURVE('',#13994,#13995,#9092,.T.);
#17968=EDGE_CURVE('',#13995,#13996,#9093,.T.);
#17969=EDGE_CURVE('',#13993,#13996,#9094,.T.);
#17970=EDGE_CURVE('',#13996,#13991,#1677,.T.);
#17971=EDGE_CURVE('',#13997,#13998,#9095,.T.);
#17972=EDGE_CURVE('',#13997,#13999,#9096,.T.);
#17973=EDGE_CURVE('',#14000,#13999,#9097,.T.);
#17974=EDGE_CURVE('',#13998,#14000,#9098,.T.);
#17975=EDGE_CURVE('',#13998,#14001,#1678,.T.);
#17976=EDGE_CURVE('',#14000,#14001,#9099,.T.);
#17977=EDGE_CURVE('',#14001,#14002,#9100,.T.);
#17978=EDGE_CURVE('',#13999,#14002,#9101,.T.);
#17979=EDGE_CURVE('',#14002,#13997,#1679,.T.);
#17980=EDGE_CURVE('',#14003,#14004,#9102,.T.);
#17981=EDGE_CURVE('',#14003,#14005,#9103,.T.);
#17982=EDGE_CURVE('',#14006,#14005,#9104,.T.);
#17983=EDGE_CURVE('',#14004,#14006,#9105,.T.);
#17984=EDGE_CURVE('',#14004,#14007,#1680,.T.);
#17985=EDGE_CURVE('',#14006,#14008,#9106,.T.);
#17986=EDGE_CURVE('',#14007,#14008,#1681,.T.);
#17987=EDGE_CURVE('',#14008,#14009,#9107,.T.);
#17988=EDGE_CURVE('',#14005,#14009,#9108,.T.);
#17989=EDGE_CURVE('',#14009,#14010,#1682,.T.);
#17990=EDGE_CURVE('',#14010,#14003,#1683,.T.);
#17991=EDGE_CURVE('',#14011,#14012,#9109,.T.);
#17992=EDGE_CURVE('',#14011,#14013,#9110,.T.);
#17993=EDGE_CURVE('',#14014,#14013,#9111,.T.);
#17994=EDGE_CURVE('',#14012,#14014,#9112,.T.);
#17995=EDGE_CURVE('',#14012,#14015,#1684,.T.);
#17996=EDGE_CURVE('',#14014,#14015,#9113,.T.);
#17997=EDGE_CURVE('',#14015,#14016,#9114,.T.);
#17998=EDGE_CURVE('',#14013,#14016,#9115,.T.);
#17999=EDGE_CURVE('',#14016,#14011,#1685,.T.);
#18000=EDGE_CURVE('',#14017,#14018,#9116,.T.);
#18001=EDGE_CURVE('',#14017,#14019,#9117,.T.);
#18002=EDGE_CURVE('',#14020,#14019,#9118,.T.);
#18003=EDGE_CURVE('',#14018,#14020,#9119,.T.);
#18004=EDGE_CURVE('',#14018,#14021,#1686,.T.);
#18005=EDGE_CURVE('',#14020,#14021,#9120,.T.);
#18006=EDGE_CURVE('',#14021,#14022,#9121,.T.);
#18007=EDGE_CURVE('',#14019,#14022,#9122,.T.);
#18008=EDGE_CURVE('',#14022,#14017,#1687,.T.);
#18009=EDGE_CURVE('',#14023,#14024,#9123,.T.);
#18010=EDGE_CURVE('',#14023,#14025,#9124,.T.);
#18011=EDGE_CURVE('',#14026,#14025,#9125,.T.);
#18012=EDGE_CURVE('',#14024,#14026,#9126,.T.);
#18013=EDGE_CURVE('',#14024,#14027,#1688,.T.);
#18014=EDGE_CURVE('',#14026,#14027,#9127,.T.);
#18015=EDGE_CURVE('',#14027,#14028,#9128,.T.);
#18016=EDGE_CURVE('',#14025,#14028,#9129,.T.);
#18017=EDGE_CURVE('',#14028,#14023,#1689,.T.);
#18018=EDGE_CURVE('',#14029,#14030,#9130,.T.);
#18019=EDGE_CURVE('',#14029,#14031,#9131,.T.);
#18020=EDGE_CURVE('',#14032,#14031,#9132,.T.);
#18021=EDGE_CURVE('',#14030,#14032,#9133,.T.);
#18022=EDGE_CURVE('',#14030,#14033,#1690,.T.);
#18023=EDGE_CURVE('',#14032,#14033,#9134,.T.);
#18024=EDGE_CURVE('',#14033,#14034,#9135,.T.);
#18025=EDGE_CURVE('',#14031,#14034,#9136,.T.);
#18026=EDGE_CURVE('',#14034,#14029,#1691,.T.);
#18027=EDGE_CURVE('',#14035,#14036,#9137,.T.);
#18028=EDGE_CURVE('',#14035,#14037,#9138,.T.);
#18029=EDGE_CURVE('',#14038,#14037,#9139,.T.);
#18030=EDGE_CURVE('',#14036,#14038,#9140,.T.);
#18031=EDGE_CURVE('',#14036,#14039,#1692,.T.);
#18032=EDGE_CURVE('',#14038,#14039,#9141,.T.);
#18033=EDGE_CURVE('',#14039,#14040,#9142,.T.);
#18034=EDGE_CURVE('',#14037,#14040,#9143,.T.);
#18035=EDGE_CURVE('',#14040,#14035,#1693,.T.);
#18036=EDGE_CURVE('',#14041,#14042,#9144,.T.);
#18037=EDGE_CURVE('',#14041,#14043,#9145,.T.);
#18038=EDGE_CURVE('',#14044,#14043,#9146,.T.);
#18039=EDGE_CURVE('',#14042,#14044,#9147,.T.);
#18040=EDGE_CURVE('',#14042,#14045,#1694,.T.);
#18041=EDGE_CURVE('',#14044,#14045,#9148,.T.);
#18042=EDGE_CURVE('',#14045,#14046,#9149,.T.);
#18043=EDGE_CURVE('',#14043,#14046,#9150,.T.);
#18044=EDGE_CURVE('',#14046,#14041,#1695,.T.);
#18045=EDGE_CURVE('',#14047,#14048,#9151,.T.);
#18046=EDGE_CURVE('',#14047,#14049,#9152,.T.);
#18047=EDGE_CURVE('',#14050,#14049,#9153,.T.);
#18048=EDGE_CURVE('',#14048,#14050,#9154,.T.);
#18049=EDGE_CURVE('',#14048,#14051,#1696,.T.);
#18050=EDGE_CURVE('',#14050,#14051,#9155,.T.);
#18051=EDGE_CURVE('',#14051,#14052,#9156,.T.);
#18052=EDGE_CURVE('',#14049,#14052,#9157,.T.);
#18053=EDGE_CURVE('',#14052,#14047,#1697,.T.);
#18054=EDGE_CURVE('',#14053,#14054,#9158,.T.);
#18055=EDGE_CURVE('',#14053,#14055,#9159,.T.);
#18056=EDGE_CURVE('',#14056,#14055,#9160,.T.);
#18057=EDGE_CURVE('',#14054,#14056,#9161,.T.);
#18058=EDGE_CURVE('',#14054,#14057,#1698,.T.);
#18059=EDGE_CURVE('',#14056,#14057,#9162,.T.);
#18060=EDGE_CURVE('',#14057,#14058,#9163,.T.);
#18061=EDGE_CURVE('',#14055,#14058,#9164,.T.);
#18062=EDGE_CURVE('',#14058,#14053,#1699,.T.);
#18063=EDGE_CURVE('',#14059,#14060,#9165,.T.);
#18064=EDGE_CURVE('',#14059,#14061,#9166,.T.);
#18065=EDGE_CURVE('',#14062,#14061,#9167,.T.);
#18066=EDGE_CURVE('',#14060,#14062,#9168,.T.);
#18067=EDGE_CURVE('',#14060,#14063,#1700,.T.);
#18068=EDGE_CURVE('',#14062,#14063,#9169,.T.);
#18069=EDGE_CURVE('',#14063,#14064,#9170,.T.);
#18070=EDGE_CURVE('',#14061,#14064,#9171,.T.);
#18071=EDGE_CURVE('',#14064,#14059,#1701,.T.);
#18072=EDGE_CURVE('',#14065,#14066,#9172,.T.);
#18073=EDGE_CURVE('',#14065,#14067,#9173,.T.);
#18074=EDGE_CURVE('',#14068,#14067,#9174,.T.);
#18075=EDGE_CURVE('',#14066,#14068,#9175,.T.);
#18076=EDGE_CURVE('',#14066,#14069,#1702,.T.);
#18077=EDGE_CURVE('',#14068,#14069,#9176,.T.);
#18078=EDGE_CURVE('',#14069,#14070,#9177,.T.);
#18079=EDGE_CURVE('',#14067,#14070,#9178,.T.);
#18080=EDGE_CURVE('',#14070,#14065,#1703,.T.);
#18081=EDGE_CURVE('',#14071,#14072,#9179,.T.);
#18082=EDGE_CURVE('',#14071,#14073,#9180,.T.);
#18083=EDGE_CURVE('',#14074,#14073,#9181,.T.);
#18084=EDGE_CURVE('',#14072,#14074,#9182,.T.);
#18085=EDGE_CURVE('',#14072,#14075,#1704,.T.);
#18086=EDGE_CURVE('',#14074,#14075,#9183,.T.);
#18087=EDGE_CURVE('',#14075,#14076,#9184,.T.);
#18088=EDGE_CURVE('',#14073,#14076,#9185,.T.);
#18089=EDGE_CURVE('',#14076,#14071,#1705,.T.);
#18090=EDGE_CURVE('',#14077,#14078,#9186,.T.);
#18091=EDGE_CURVE('',#14077,#14079,#9187,.T.);
#18092=EDGE_CURVE('',#14080,#14079,#9188,.T.);
#18093=EDGE_CURVE('',#14078,#14080,#9189,.T.);
#18094=EDGE_CURVE('',#14078,#14081,#1706,.T.);
#18095=EDGE_CURVE('',#14080,#14081,#9190,.T.);
#18096=EDGE_CURVE('',#14081,#14082,#9191,.T.);
#18097=EDGE_CURVE('',#14079,#14082,#9192,.T.);
#18098=EDGE_CURVE('',#14082,#14077,#1707,.T.);
#18099=EDGE_CURVE('',#14083,#14084,#9193,.T.);
#18100=EDGE_CURVE('',#14083,#14085,#9194,.T.);
#18101=EDGE_CURVE('',#14086,#14085,#9195,.T.);
#18102=EDGE_CURVE('',#14084,#14086,#9196,.T.);
#18103=EDGE_CURVE('',#14084,#14087,#1708,.T.);
#18104=EDGE_CURVE('',#14086,#14087,#9197,.T.);
#18105=EDGE_CURVE('',#14087,#14088,#9198,.T.);
#18106=EDGE_CURVE('',#14085,#14088,#9199,.T.);
#18107=EDGE_CURVE('',#14088,#14083,#1709,.T.);
#18108=EDGE_CURVE('',#14089,#14090,#9200,.T.);
#18109=EDGE_CURVE('',#14089,#14091,#9201,.T.);
#18110=EDGE_CURVE('',#14092,#14091,#9202,.T.);
#18111=EDGE_CURVE('',#14090,#14092,#9203,.T.);
#18112=EDGE_CURVE('',#14090,#14093,#1710,.T.);
#18113=EDGE_CURVE('',#14092,#14093,#9204,.T.);
#18114=EDGE_CURVE('',#14093,#14094,#9205,.T.);
#18115=EDGE_CURVE('',#14091,#14094,#9206,.T.);
#18116=EDGE_CURVE('',#14094,#14089,#1711,.T.);
#18117=EDGE_CURVE('',#14095,#14096,#9207,.T.);
#18118=EDGE_CURVE('',#14095,#14097,#9208,.T.);
#18119=EDGE_CURVE('',#14098,#14097,#9209,.T.);
#18120=EDGE_CURVE('',#14096,#14098,#9210,.T.);
#18121=EDGE_CURVE('',#14096,#14099,#1712,.T.);
#18122=EDGE_CURVE('',#14098,#14099,#9211,.T.);
#18123=EDGE_CURVE('',#14099,#14100,#9212,.T.);
#18124=EDGE_CURVE('',#14097,#14100,#9213,.T.);
#18125=EDGE_CURVE('',#14100,#14095,#1713,.T.);
#18126=EDGE_CURVE('',#14101,#14102,#9214,.T.);
#18127=EDGE_CURVE('',#14101,#14103,#9215,.T.);
#18128=EDGE_CURVE('',#14104,#14103,#9216,.T.);
#18129=EDGE_CURVE('',#14102,#14104,#9217,.T.);
#18130=EDGE_CURVE('',#14102,#14105,#1714,.T.);
#18131=EDGE_CURVE('',#14104,#14105,#9218,.T.);
#18132=EDGE_CURVE('',#14105,#14106,#9219,.T.);
#18133=EDGE_CURVE('',#14103,#14106,#9220,.T.);
#18134=EDGE_CURVE('',#14106,#14101,#1715,.T.);
#18135=EDGE_CURVE('',#14107,#14108,#9221,.T.);
#18136=EDGE_CURVE('',#14107,#14109,#9222,.T.);
#18137=EDGE_CURVE('',#14110,#14109,#9223,.T.);
#18138=EDGE_CURVE('',#14108,#14110,#9224,.T.);
#18139=EDGE_CURVE('',#14108,#14111,#1716,.T.);
#18140=EDGE_CURVE('',#14110,#14111,#9225,.T.);
#18141=EDGE_CURVE('',#14111,#14112,#9226,.T.);
#18142=EDGE_CURVE('',#14109,#14112,#9227,.T.);
#18143=EDGE_CURVE('',#14112,#14107,#1717,.T.);
#18144=EDGE_CURVE('',#14113,#14114,#9228,.T.);
#18145=EDGE_CURVE('',#14113,#14115,#9229,.T.);
#18146=EDGE_CURVE('',#14116,#14115,#9230,.T.);
#18147=EDGE_CURVE('',#14114,#14116,#9231,.T.);
#18148=EDGE_CURVE('',#14114,#14117,#1718,.T.);
#18149=EDGE_CURVE('',#14116,#14117,#9232,.T.);
#18150=EDGE_CURVE('',#14117,#14118,#9233,.T.);
#18151=EDGE_CURVE('',#14115,#14118,#9234,.T.);
#18152=EDGE_CURVE('',#14118,#14113,#1719,.T.);
#18153=EDGE_CURVE('',#14119,#14120,#9235,.T.);
#18154=EDGE_CURVE('',#14120,#14120,#1720,.T.);
#18155=EDGE_CURVE('',#14121,#14122,#9236,.T.);
#18156=EDGE_CURVE('',#14121,#14123,#9237,.T.);
#18157=EDGE_CURVE('',#14123,#14124,#9238,.T.);
#18158=EDGE_CURVE('',#14122,#14124,#9239,.T.);
#18159=EDGE_CURVE('',#14125,#14121,#9240,.T.);
#18160=EDGE_CURVE('',#14125,#14126,#9241,.T.);
#18161=EDGE_CURVE('',#14126,#14123,#9242,.T.);
#18162=EDGE_CURVE('',#14127,#14125,#9243,.T.);
#18163=EDGE_CURVE('',#14127,#14128,#9244,.T.);
#18164=EDGE_CURVE('',#14128,#14126,#9245,.T.);
#18165=EDGE_CURVE('',#14129,#14127,#9246,.T.);
#18166=EDGE_CURVE('',#14129,#14130,#9247,.T.);
#18167=EDGE_CURVE('',#14130,#14128,#9248,.T.);
#18168=EDGE_CURVE('',#14131,#14129,#9249,.T.);
#18169=EDGE_CURVE('',#14131,#14132,#9250,.T.);
#18170=EDGE_CURVE('',#14132,#14130,#9251,.T.);
#18171=EDGE_CURVE('',#14122,#14131,#9252,.T.);
#18172=EDGE_CURVE('',#14124,#14132,#9253,.T.);
#18173=EDGE_CURVE('',#14133,#14133,#1721,.T.);
#18174=EDGE_CURVE('',#13897,#14133,#9254,.T.);
#18175=EDGE_CURVE('',#14134,#14134,#1722,.T.);
#18176=EDGE_CURVE('',#14134,#14010,#9255,.T.);
#18177=EDGE_CURVE('',#14007,#13900,#9256,.T.);
#18178=EDGE_CURVE('',#14135,#14135,#1723,.T.);
#18179=EDGE_CURVE('',#14135,#14134,#9257,.T.);
#24345=ORIENTED_EDGE('',*,*,#17394,.F.);
#24346=ORIENTED_EDGE('',*,*,#17395,.T.);
#24347=ORIENTED_EDGE('',*,*,#17396,.T.);
#24348=ORIENTED_EDGE('',*,*,#17397,.T.);
#24349=ORIENTED_EDGE('',*,*,#17398,.F.);
#24350=ORIENTED_EDGE('',*,*,#17399,.T.);
#24351=ORIENTED_EDGE('',*,*,#17394,.T.);
#24352=ORIENTED_EDGE('',*,*,#17400,.T.);
#24353=ORIENTED_EDGE('',*,*,#17401,.F.);
#24354=ORIENTED_EDGE('',*,*,#17402,.T.);
#24355=ORIENTED_EDGE('',*,*,#17398,.T.);
#24356=ORIENTED_EDGE('',*,*,#17403,.T.);
#24357=ORIENTED_EDGE('',*,*,#17404,.F.);
#24358=ORIENTED_EDGE('',*,*,#17405,.T.);
#24359=ORIENTED_EDGE('',*,*,#17401,.T.);
#24360=ORIENTED_EDGE('',*,*,#17406,.T.);
#24361=ORIENTED_EDGE('',*,*,#17407,.F.);
#24362=ORIENTED_EDGE('',*,*,#17408,.T.);
#24363=ORIENTED_EDGE('',*,*,#17404,.T.);
#24364=ORIENTED_EDGE('',*,*,#17409,.T.);
#24365=ORIENTED_EDGE('',*,*,#17410,.F.);
#24366=ORIENTED_EDGE('',*,*,#17411,.T.);
#24367=ORIENTED_EDGE('',*,*,#17407,.T.);
#24368=ORIENTED_EDGE('',*,*,#17412,.T.);
#24369=ORIENTED_EDGE('',*,*,#17413,.F.);
#24370=ORIENTED_EDGE('',*,*,#17414,.T.);
#24371=ORIENTED_EDGE('',*,*,#17410,.T.);
#24372=ORIENTED_EDGE('',*,*,#17415,.T.);
#24373=ORIENTED_EDGE('',*,*,#17416,.F.);
#24374=ORIENTED_EDGE('',*,*,#17417,.T.);
#24375=ORIENTED_EDGE('',*,*,#17413,.T.);
#24376=ORIENTED_EDGE('',*,*,#17418,.T.);
#24377=ORIENTED_EDGE('',*,*,#17419,.F.);
#24378=ORIENTED_EDGE('',*,*,#17420,.T.);
#24379=ORIENTED_EDGE('',*,*,#17416,.T.);
#24380=ORIENTED_EDGE('',*,*,#17421,.T.);
#24381=ORIENTED_EDGE('',*,*,#17422,.F.);
#24382=ORIENTED_EDGE('',*,*,#17423,.T.);
#24383=ORIENTED_EDGE('',*,*,#17419,.T.);
#24384=ORIENTED_EDGE('',*,*,#17424,.T.);
#24385=ORIENTED_EDGE('',*,*,#17425,.F.);
#24386=ORIENTED_EDGE('',*,*,#17426,.T.);
#24387=ORIENTED_EDGE('',*,*,#17422,.T.);
#24388=ORIENTED_EDGE('',*,*,#17427,.T.);
#24389=ORIENTED_EDGE('',*,*,#17428,.F.);
#24390=ORIENTED_EDGE('',*,*,#17429,.T.);
#24391=ORIENTED_EDGE('',*,*,#17425,.T.);
#24392=ORIENTED_EDGE('',*,*,#17430,.T.);
#24393=ORIENTED_EDGE('',*,*,#17431,.F.);
#24394=ORIENTED_EDGE('',*,*,#17432,.T.);
#24395=ORIENTED_EDGE('',*,*,#17428,.T.);
#24396=ORIENTED_EDGE('',*,*,#17433,.T.);
#24397=ORIENTED_EDGE('',*,*,#17434,.F.);
#24398=ORIENTED_EDGE('',*,*,#17435,.T.);
#24399=ORIENTED_EDGE('',*,*,#17431,.T.);
#24400=ORIENTED_EDGE('',*,*,#17436,.T.);
#24401=ORIENTED_EDGE('',*,*,#17437,.F.);
#24402=ORIENTED_EDGE('',*,*,#17438,.T.);
#24403=ORIENTED_EDGE('',*,*,#17434,.T.);
#24404=ORIENTED_EDGE('',*,*,#17439,.T.);
#24405=ORIENTED_EDGE('',*,*,#17440,.F.);
#24406=ORIENTED_EDGE('',*,*,#17441,.T.);
#24407=ORIENTED_EDGE('',*,*,#17437,.T.);
#24408=ORIENTED_EDGE('',*,*,#17442,.T.);
#24409=ORIENTED_EDGE('',*,*,#17443,.F.);
#24410=ORIENTED_EDGE('',*,*,#17444,.T.);
#24411=ORIENTED_EDGE('',*,*,#17440,.T.);
#24412=ORIENTED_EDGE('',*,*,#17445,.T.);
#24413=ORIENTED_EDGE('',*,*,#17446,.F.);
#24414=ORIENTED_EDGE('',*,*,#17447,.T.);
#24415=ORIENTED_EDGE('',*,*,#17443,.T.);
#24416=ORIENTED_EDGE('',*,*,#17448,.T.);
#24417=ORIENTED_EDGE('',*,*,#17449,.F.);
#24418=ORIENTED_EDGE('',*,*,#17450,.T.);
#24419=ORIENTED_EDGE('',*,*,#17446,.T.);
#24420=ORIENTED_EDGE('',*,*,#17451,.T.);
#24421=ORIENTED_EDGE('',*,*,#17452,.F.);
#24422=ORIENTED_EDGE('',*,*,#17453,.T.);
#24423=ORIENTED_EDGE('',*,*,#17449,.T.);
#24424=ORIENTED_EDGE('',*,*,#17454,.T.);
#24425=ORIENTED_EDGE('',*,*,#17455,.F.);
#24426=ORIENTED_EDGE('',*,*,#17456,.T.);
#24427=ORIENTED_EDGE('',*,*,#17452,.T.);
#24428=ORIENTED_EDGE('',*,*,#17457,.T.);
#24429=ORIENTED_EDGE('',*,*,#17458,.F.);
#24430=ORIENTED_EDGE('',*,*,#17459,.T.);
#24431=ORIENTED_EDGE('',*,*,#17455,.T.);
#24432=ORIENTED_EDGE('',*,*,#17460,.T.);
#24433=ORIENTED_EDGE('',*,*,#17461,.F.);
#24434=ORIENTED_EDGE('',*,*,#17462,.T.);
#24435=ORIENTED_EDGE('',*,*,#17458,.T.);
#24436=ORIENTED_EDGE('',*,*,#17463,.T.);
#24437=ORIENTED_EDGE('',*,*,#17464,.F.);
#24438=ORIENTED_EDGE('',*,*,#17465,.T.);
#24439=ORIENTED_EDGE('',*,*,#17461,.T.);
#24440=ORIENTED_EDGE('',*,*,#17466,.T.);
#24441=ORIENTED_EDGE('',*,*,#17467,.F.);
#24442=ORIENTED_EDGE('',*,*,#17468,.T.);
#24443=ORIENTED_EDGE('',*,*,#17464,.T.);
#24444=ORIENTED_EDGE('',*,*,#17469,.T.);
#24445=ORIENTED_EDGE('',*,*,#17470,.F.);
#24446=ORIENTED_EDGE('',*,*,#17471,.T.);
#24447=ORIENTED_EDGE('',*,*,#17467,.T.);
#24448=ORIENTED_EDGE('',*,*,#17472,.T.);
#24449=ORIENTED_EDGE('',*,*,#17473,.F.);
#24450=ORIENTED_EDGE('',*,*,#17474,.T.);
#24451=ORIENTED_EDGE('',*,*,#17470,.T.);
#24452=ORIENTED_EDGE('',*,*,#17475,.T.);
#24453=ORIENTED_EDGE('',*,*,#17476,.F.);
#24454=ORIENTED_EDGE('',*,*,#17477,.T.);
#24455=ORIENTED_EDGE('',*,*,#17473,.T.);
#24456=ORIENTED_EDGE('',*,*,#17478,.T.);
#24457=ORIENTED_EDGE('',*,*,#17479,.F.);
#24458=ORIENTED_EDGE('',*,*,#17480,.T.);
#24459=ORIENTED_EDGE('',*,*,#17476,.T.);
#24460=ORIENTED_EDGE('',*,*,#17481,.T.);
#24461=ORIENTED_EDGE('',*,*,#17482,.F.);
#24462=ORIENTED_EDGE('',*,*,#17483,.T.);
#24463=ORIENTED_EDGE('',*,*,#17479,.T.);
#24464=ORIENTED_EDGE('',*,*,#17484,.T.);
#24465=ORIENTED_EDGE('',*,*,#17485,.F.);
#24466=ORIENTED_EDGE('',*,*,#17486,.T.);
#24467=ORIENTED_EDGE('',*,*,#17482,.T.);
#24468=ORIENTED_EDGE('',*,*,#17487,.T.);
#24469=ORIENTED_EDGE('',*,*,#17488,.F.);
#24470=ORIENTED_EDGE('',*,*,#17489,.T.);
#24471=ORIENTED_EDGE('',*,*,#17485,.T.);
#24472=ORIENTED_EDGE('',*,*,#17490,.T.);
#24473=ORIENTED_EDGE('',*,*,#17491,.F.);
#24474=ORIENTED_EDGE('',*,*,#17492,.T.);
#24475=ORIENTED_EDGE('',*,*,#17488,.T.);
#24476=ORIENTED_EDGE('',*,*,#17493,.T.);
#24477=ORIENTED_EDGE('',*,*,#17494,.F.);
#24478=ORIENTED_EDGE('',*,*,#17495,.T.);
#24479=ORIENTED_EDGE('',*,*,#17491,.T.);
#24480=ORIENTED_EDGE('',*,*,#17496,.T.);
#24481=ORIENTED_EDGE('',*,*,#17497,.F.);
#24482=ORIENTED_EDGE('',*,*,#17498,.T.);
#24483=ORIENTED_EDGE('',*,*,#17494,.T.);
#24484=ORIENTED_EDGE('',*,*,#17499,.T.);
#24485=ORIENTED_EDGE('',*,*,#17500,.F.);
#24486=ORIENTED_EDGE('',*,*,#17501,.T.);
#24487=ORIENTED_EDGE('',*,*,#17497,.T.);
#24488=ORIENTED_EDGE('',*,*,#17502,.T.);
#24489=ORIENTED_EDGE('',*,*,#17503,.F.);
#24490=ORIENTED_EDGE('',*,*,#17504,.T.);
#24491=ORIENTED_EDGE('',*,*,#17500,.T.);
#24492=ORIENTED_EDGE('',*,*,#17505,.T.);
#24493=ORIENTED_EDGE('',*,*,#17506,.F.);
#24494=ORIENTED_EDGE('',*,*,#17507,.T.);
#24495=ORIENTED_EDGE('',*,*,#17503,.T.);
#24496=ORIENTED_EDGE('',*,*,#17508,.T.);
#24497=ORIENTED_EDGE('',*,*,#17509,.F.);
#24498=ORIENTED_EDGE('',*,*,#17510,.T.);
#24499=ORIENTED_EDGE('',*,*,#17506,.T.);
#24500=ORIENTED_EDGE('',*,*,#17511,.T.);
#24501=ORIENTED_EDGE('',*,*,#17512,.F.);
#24502=ORIENTED_EDGE('',*,*,#17513,.T.);
#24503=ORIENTED_EDGE('',*,*,#17509,.T.);
#24504=ORIENTED_EDGE('',*,*,#17514,.T.);
#24505=ORIENTED_EDGE('',*,*,#17515,.F.);
#24506=ORIENTED_EDGE('',*,*,#17516,.T.);
#24507=ORIENTED_EDGE('',*,*,#17512,.T.);
#24508=ORIENTED_EDGE('',*,*,#17517,.T.);
#24509=ORIENTED_EDGE('',*,*,#17518,.F.);
#24510=ORIENTED_EDGE('',*,*,#17519,.T.);
#24511=ORIENTED_EDGE('',*,*,#17515,.T.);
#24512=ORIENTED_EDGE('',*,*,#17520,.T.);
#24513=ORIENTED_EDGE('',*,*,#17521,.F.);
#24514=ORIENTED_EDGE('',*,*,#17522,.T.);
#24515=ORIENTED_EDGE('',*,*,#17518,.T.);
#24516=ORIENTED_EDGE('',*,*,#17523,.T.);
#24517=ORIENTED_EDGE('',*,*,#17524,.F.);
#24518=ORIENTED_EDGE('',*,*,#17525,.T.);
#24519=ORIENTED_EDGE('',*,*,#17521,.T.);
#24520=ORIENTED_EDGE('',*,*,#17526,.T.);
#24521=ORIENTED_EDGE('',*,*,#17527,.F.);
#24522=ORIENTED_EDGE('',*,*,#17528,.T.);
#24523=ORIENTED_EDGE('',*,*,#17524,.T.);
#24524=ORIENTED_EDGE('',*,*,#17529,.T.);
#24525=ORIENTED_EDGE('',*,*,#17530,.F.);
#24526=ORIENTED_EDGE('',*,*,#17531,.T.);
#24527=ORIENTED_EDGE('',*,*,#17527,.T.);
#24528=ORIENTED_EDGE('',*,*,#17532,.T.);
#24529=ORIENTED_EDGE('',*,*,#17533,.F.);
#24530=ORIENTED_EDGE('',*,*,#17534,.T.);
#24531=ORIENTED_EDGE('',*,*,#17530,.T.);
#24532=ORIENTED_EDGE('',*,*,#17535,.T.);
#24533=ORIENTED_EDGE('',*,*,#17536,.F.);
#24534=ORIENTED_EDGE('',*,*,#17537,.T.);
#24535=ORIENTED_EDGE('',*,*,#17533,.T.);
#24536=ORIENTED_EDGE('',*,*,#17538,.T.);
#24537=ORIENTED_EDGE('',*,*,#17539,.F.);
#24538=ORIENTED_EDGE('',*,*,#17540,.T.);
#24539=ORIENTED_EDGE('',*,*,#17536,.T.);
#24540=ORIENTED_EDGE('',*,*,#17541,.T.);
#24541=ORIENTED_EDGE('',*,*,#17542,.F.);
#24542=ORIENTED_EDGE('',*,*,#17543,.T.);
#24543=ORIENTED_EDGE('',*,*,#17539,.T.);
#24544=ORIENTED_EDGE('',*,*,#17544,.T.);
#24545=ORIENTED_EDGE('',*,*,#17545,.F.);
#24546=ORIENTED_EDGE('',*,*,#17546,.T.);
#24547=ORIENTED_EDGE('',*,*,#17542,.T.);
#24548=ORIENTED_EDGE('',*,*,#17547,.T.);
#24549=ORIENTED_EDGE('',*,*,#17548,.F.);
#24550=ORIENTED_EDGE('',*,*,#17549,.T.);
#24551=ORIENTED_EDGE('',*,*,#17545,.T.);
#24552=ORIENTED_EDGE('',*,*,#17550,.T.);
#24553=ORIENTED_EDGE('',*,*,#17551,.F.);
#24554=ORIENTED_EDGE('',*,*,#17552,.T.);
#24555=ORIENTED_EDGE('',*,*,#17548,.T.);
#24556=ORIENTED_EDGE('',*,*,#17553,.T.);
#24557=ORIENTED_EDGE('',*,*,#17554,.F.);
#24558=ORIENTED_EDGE('',*,*,#17555,.T.);
#24559=ORIENTED_EDGE('',*,*,#17551,.T.);
#24560=ORIENTED_EDGE('',*,*,#17556,.T.);
#24561=ORIENTED_EDGE('',*,*,#17557,.F.);
#24562=ORIENTED_EDGE('',*,*,#17558,.T.);
#24563=ORIENTED_EDGE('',*,*,#17554,.T.);
#24564=ORIENTED_EDGE('',*,*,#17559,.T.);
#24565=ORIENTED_EDGE('',*,*,#17560,.F.);
#24566=ORIENTED_EDGE('',*,*,#17561,.T.);
#24567=ORIENTED_EDGE('',*,*,#17557,.T.);
#24568=ORIENTED_EDGE('',*,*,#17562,.T.);
#24569=ORIENTED_EDGE('',*,*,#17563,.F.);
#24570=ORIENTED_EDGE('',*,*,#17564,.T.);
#24571=ORIENTED_EDGE('',*,*,#17560,.T.);
#24572=ORIENTED_EDGE('',*,*,#17565,.T.);
#24573=ORIENTED_EDGE('',*,*,#17566,.F.);
#24574=ORIENTED_EDGE('',*,*,#17567,.T.);
#24575=ORIENTED_EDGE('',*,*,#17563,.T.);
#24576=ORIENTED_EDGE('',*,*,#17568,.T.);
#24577=ORIENTED_EDGE('',*,*,#17569,.F.);
#24578=ORIENTED_EDGE('',*,*,#17570,.T.);
#24579=ORIENTED_EDGE('',*,*,#17566,.T.);
#24580=ORIENTED_EDGE('',*,*,#17571,.T.);
#24581=ORIENTED_EDGE('',*,*,#17572,.F.);
#24582=ORIENTED_EDGE('',*,*,#17573,.T.);
#24583=ORIENTED_EDGE('',*,*,#17569,.T.);
#24584=ORIENTED_EDGE('',*,*,#17574,.T.);
#24585=ORIENTED_EDGE('',*,*,#17575,.F.);
#24586=ORIENTED_EDGE('',*,*,#17576,.T.);
#24587=ORIENTED_EDGE('',*,*,#17572,.T.);
#24588=ORIENTED_EDGE('',*,*,#17577,.T.);
#24589=ORIENTED_EDGE('',*,*,#17578,.F.);
#24590=ORIENTED_EDGE('',*,*,#17579,.T.);
#24591=ORIENTED_EDGE('',*,*,#17575,.T.);
#24592=ORIENTED_EDGE('',*,*,#17580,.T.);
#24593=ORIENTED_EDGE('',*,*,#17581,.F.);
#24594=ORIENTED_EDGE('',*,*,#17582,.T.);
#24595=ORIENTED_EDGE('',*,*,#17578,.T.);
#24596=ORIENTED_EDGE('',*,*,#17583,.T.);
#24597=ORIENTED_EDGE('',*,*,#17584,.F.);
#24598=ORIENTED_EDGE('',*,*,#17585,.T.);
#24599=ORIENTED_EDGE('',*,*,#17581,.T.);
#24600=ORIENTED_EDGE('',*,*,#17586,.T.);
#24601=ORIENTED_EDGE('',*,*,#17587,.F.);
#24602=ORIENTED_EDGE('',*,*,#17588,.T.);
#24603=ORIENTED_EDGE('',*,*,#17584,.T.);
#24604=ORIENTED_EDGE('',*,*,#17589,.T.);
#24605=ORIENTED_EDGE('',*,*,#17590,.F.);
#24606=ORIENTED_EDGE('',*,*,#17591,.T.);
#24607=ORIENTED_EDGE('',*,*,#17587,.T.);
#24608=ORIENTED_EDGE('',*,*,#17592,.T.);
#24609=ORIENTED_EDGE('',*,*,#17593,.F.);
#24610=ORIENTED_EDGE('',*,*,#17594,.T.);
#24611=ORIENTED_EDGE('',*,*,#17590,.T.);
#24612=ORIENTED_EDGE('',*,*,#17595,.T.);
#24613=ORIENTED_EDGE('',*,*,#17596,.F.);
#24614=ORIENTED_EDGE('',*,*,#17597,.T.);
#24615=ORIENTED_EDGE('',*,*,#17593,.T.);
#24616=ORIENTED_EDGE('',*,*,#17598,.T.);
#24617=ORIENTED_EDGE('',*,*,#17599,.F.);
#24618=ORIENTED_EDGE('',*,*,#17600,.T.);
#24619=ORIENTED_EDGE('',*,*,#17596,.T.);
#24620=ORIENTED_EDGE('',*,*,#17601,.T.);
#24621=ORIENTED_EDGE('',*,*,#17602,.F.);
#24622=ORIENTED_EDGE('',*,*,#17603,.T.);
#24623=ORIENTED_EDGE('',*,*,#17604,.F.);
#24624=ORIENTED_EDGE('',*,*,#17605,.F.);
#24625=ORIENTED_EDGE('',*,*,#17606,.F.);
#24626=ORIENTED_EDGE('',*,*,#17607,.T.);
#24627=ORIENTED_EDGE('',*,*,#17602,.T.);
#24628=ORIENTED_EDGE('',*,*,#17608,.F.);
#24629=ORIENTED_EDGE('',*,*,#17609,.F.);
#24630=ORIENTED_EDGE('',*,*,#17610,.T.);
#24631=ORIENTED_EDGE('',*,*,#17606,.T.);
#24632=ORIENTED_EDGE('',*,*,#17611,.F.);
#24633=ORIENTED_EDGE('',*,*,#17612,.F.);
#24634=ORIENTED_EDGE('',*,*,#17613,.T.);
#24635=ORIENTED_EDGE('',*,*,#17609,.T.);
#24636=ORIENTED_EDGE('',*,*,#17614,.F.);
#24637=ORIENTED_EDGE('',*,*,#17615,.F.);
#24638=ORIENTED_EDGE('',*,*,#17616,.T.);
#24639=ORIENTED_EDGE('',*,*,#17612,.T.);
#24640=ORIENTED_EDGE('',*,*,#17617,.F.);
#24641=ORIENTED_EDGE('',*,*,#17618,.F.);
#24642=ORIENTED_EDGE('',*,*,#17619,.T.);
#24643=ORIENTED_EDGE('',*,*,#17615,.T.);
#24644=ORIENTED_EDGE('',*,*,#17620,.F.);
#24645=ORIENTED_EDGE('',*,*,#17621,.F.);
#24646=ORIENTED_EDGE('',*,*,#17622,.T.);
#24647=ORIENTED_EDGE('',*,*,#17618,.T.);
#24648=ORIENTED_EDGE('',*,*,#17623,.F.);
#24649=ORIENTED_EDGE('',*,*,#17624,.F.);
#24650=ORIENTED_EDGE('',*,*,#17625,.T.);
#24651=ORIENTED_EDGE('',*,*,#17621,.T.);
#24652=ORIENTED_EDGE('',*,*,#17626,.F.);
#24653=ORIENTED_EDGE('',*,*,#17627,.F.);
#24654=ORIENTED_EDGE('',*,*,#17628,.T.);
#24655=ORIENTED_EDGE('',*,*,#17624,.T.);
#24656=ORIENTED_EDGE('',*,*,#17629,.F.);
#24657=ORIENTED_EDGE('',*,*,#17630,.F.);
#24658=ORIENTED_EDGE('',*,*,#17631,.T.);
#24659=ORIENTED_EDGE('',*,*,#17627,.T.);
#24660=ORIENTED_EDGE('',*,*,#17632,.F.);
#24661=ORIENTED_EDGE('',*,*,#17633,.F.);
#24662=ORIENTED_EDGE('',*,*,#17634,.T.);
#24663=ORIENTED_EDGE('',*,*,#17630,.T.);
#24664=ORIENTED_EDGE('',*,*,#17635,.F.);
#24665=ORIENTED_EDGE('',*,*,#17636,.F.);
#24666=ORIENTED_EDGE('',*,*,#17637,.T.);
#24667=ORIENTED_EDGE('',*,*,#17633,.T.);
#24668=ORIENTED_EDGE('',*,*,#17638,.F.);
#24669=ORIENTED_EDGE('',*,*,#17639,.F.);
#24670=ORIENTED_EDGE('',*,*,#17640,.T.);
#24671=ORIENTED_EDGE('',*,*,#17636,.T.);
#24672=ORIENTED_EDGE('',*,*,#17641,.F.);
#24673=ORIENTED_EDGE('',*,*,#17642,.F.);
#24674=ORIENTED_EDGE('',*,*,#17643,.T.);
#24675=ORIENTED_EDGE('',*,*,#17639,.T.);
#24676=ORIENTED_EDGE('',*,*,#17644,.F.);
#24677=ORIENTED_EDGE('',*,*,#17645,.F.);
#24678=ORIENTED_EDGE('',*,*,#17646,.T.);
#24679=ORIENTED_EDGE('',*,*,#17642,.T.);
#24680=ORIENTED_EDGE('',*,*,#17647,.F.);
#24681=ORIENTED_EDGE('',*,*,#17648,.F.);
#24682=ORIENTED_EDGE('',*,*,#17649,.T.);
#24683=ORIENTED_EDGE('',*,*,#17645,.T.);
#24684=ORIENTED_EDGE('',*,*,#17650,.F.);
#24685=ORIENTED_EDGE('',*,*,#17651,.F.);
#24686=ORIENTED_EDGE('',*,*,#17652,.T.);
#24687=ORIENTED_EDGE('',*,*,#17648,.T.);
#24688=ORIENTED_EDGE('',*,*,#17653,.F.);
#24689=ORIENTED_EDGE('',*,*,#17654,.F.);
#24690=ORIENTED_EDGE('',*,*,#17655,.T.);
#24691=ORIENTED_EDGE('',*,*,#17651,.T.);
#24692=ORIENTED_EDGE('',*,*,#17656,.F.);
#24693=ORIENTED_EDGE('',*,*,#17657,.F.);
#24694=ORIENTED_EDGE('',*,*,#17658,.T.);
#24695=ORIENTED_EDGE('',*,*,#17654,.T.);
#24696=ORIENTED_EDGE('',*,*,#17659,.F.);
#24697=ORIENTED_EDGE('',*,*,#17660,.F.);
#24698=ORIENTED_EDGE('',*,*,#17661,.T.);
#24699=ORIENTED_EDGE('',*,*,#17657,.T.);
#24700=ORIENTED_EDGE('',*,*,#17662,.F.);
#24701=ORIENTED_EDGE('',*,*,#17663,.F.);
#24702=ORIENTED_EDGE('',*,*,#17664,.T.);
#24703=ORIENTED_EDGE('',*,*,#17660,.T.);
#24704=ORIENTED_EDGE('',*,*,#17665,.F.);
#24705=ORIENTED_EDGE('',*,*,#17666,.F.);
#24706=ORIENTED_EDGE('',*,*,#17667,.T.);
#24707=ORIENTED_EDGE('',*,*,#17663,.T.);
#24708=ORIENTED_EDGE('',*,*,#17668,.F.);
#24709=ORIENTED_EDGE('',*,*,#17669,.F.);
#24710=ORIENTED_EDGE('',*,*,#17670,.T.);
#24711=ORIENTED_EDGE('',*,*,#17666,.T.);
#24712=ORIENTED_EDGE('',*,*,#17671,.F.);
#24713=ORIENTED_EDGE('',*,*,#17672,.F.);
#24714=ORIENTED_EDGE('',*,*,#17673,.T.);
#24715=ORIENTED_EDGE('',*,*,#17669,.T.);
#24716=ORIENTED_EDGE('',*,*,#17674,.F.);
#24717=ORIENTED_EDGE('',*,*,#17675,.F.);
#24718=ORIENTED_EDGE('',*,*,#17676,.T.);
#24719=ORIENTED_EDGE('',*,*,#17672,.T.);
#24720=ORIENTED_EDGE('',*,*,#17677,.F.);
#24721=ORIENTED_EDGE('',*,*,#17678,.F.);
#24722=ORIENTED_EDGE('',*,*,#17679,.T.);
#24723=ORIENTED_EDGE('',*,*,#17675,.T.);
#24724=ORIENTED_EDGE('',*,*,#17680,.F.);
#24725=ORIENTED_EDGE('',*,*,#17681,.F.);
#24726=ORIENTED_EDGE('',*,*,#17682,.T.);
#24727=ORIENTED_EDGE('',*,*,#17678,.T.);
#24728=ORIENTED_EDGE('',*,*,#17683,.F.);
#24729=ORIENTED_EDGE('',*,*,#17684,.F.);
#24730=ORIENTED_EDGE('',*,*,#17685,.T.);
#24731=ORIENTED_EDGE('',*,*,#17681,.T.);
#24732=ORIENTED_EDGE('',*,*,#17686,.F.);
#24733=ORIENTED_EDGE('',*,*,#17687,.F.);
#24734=ORIENTED_EDGE('',*,*,#17688,.T.);
#24735=ORIENTED_EDGE('',*,*,#17684,.T.);
#24736=ORIENTED_EDGE('',*,*,#17689,.F.);
#24737=ORIENTED_EDGE('',*,*,#17690,.F.);
#24738=ORIENTED_EDGE('',*,*,#17691,.T.);
#24739=ORIENTED_EDGE('',*,*,#17687,.T.);
#24740=ORIENTED_EDGE('',*,*,#17692,.F.);
#24741=ORIENTED_EDGE('',*,*,#17693,.F.);
#24742=ORIENTED_EDGE('',*,*,#17694,.T.);
#24743=ORIENTED_EDGE('',*,*,#17690,.T.);
#24744=ORIENTED_EDGE('',*,*,#17695,.F.);
#24745=ORIENTED_EDGE('',*,*,#17696,.F.);
#24746=ORIENTED_EDGE('',*,*,#17697,.T.);
#24747=ORIENTED_EDGE('',*,*,#17693,.T.);
#24748=ORIENTED_EDGE('',*,*,#17698,.F.);
#24749=ORIENTED_EDGE('',*,*,#17699,.F.);
#24750=ORIENTED_EDGE('',*,*,#17700,.T.);
#24751=ORIENTED_EDGE('',*,*,#17696,.T.);
#24752=ORIENTED_EDGE('',*,*,#17701,.F.);
#24753=ORIENTED_EDGE('',*,*,#17702,.F.);
#24754=ORIENTED_EDGE('',*,*,#17703,.T.);
#24755=ORIENTED_EDGE('',*,*,#17699,.T.);
#24756=ORIENTED_EDGE('',*,*,#17704,.F.);
#24757=ORIENTED_EDGE('',*,*,#17705,.F.);
#24758=ORIENTED_EDGE('',*,*,#17706,.T.);
#24759=ORIENTED_EDGE('',*,*,#17702,.T.);
#24760=ORIENTED_EDGE('',*,*,#17707,.F.);
#24761=ORIENTED_EDGE('',*,*,#17708,.F.);
#24762=ORIENTED_EDGE('',*,*,#17709,.T.);
#24763=ORIENTED_EDGE('',*,*,#17705,.T.);
#24764=ORIENTED_EDGE('',*,*,#17710,.F.);
#24765=ORIENTED_EDGE('',*,*,#17711,.F.);
#24766=ORIENTED_EDGE('',*,*,#17712,.T.);
#24767=ORIENTED_EDGE('',*,*,#17708,.T.);
#24768=ORIENTED_EDGE('',*,*,#17713,.F.);
#24769=ORIENTED_EDGE('',*,*,#17714,.F.);
#24770=ORIENTED_EDGE('',*,*,#17715,.T.);
#24771=ORIENTED_EDGE('',*,*,#17711,.T.);
#24772=ORIENTED_EDGE('',*,*,#17716,.F.);
#24773=ORIENTED_EDGE('',*,*,#17717,.F.);
#24774=ORIENTED_EDGE('',*,*,#17718,.T.);
#24775=ORIENTED_EDGE('',*,*,#17714,.T.);
#24776=ORIENTED_EDGE('',*,*,#17719,.F.);
#24777=ORIENTED_EDGE('',*,*,#17720,.F.);
#24778=ORIENTED_EDGE('',*,*,#17721,.T.);
#24779=ORIENTED_EDGE('',*,*,#17717,.T.);
#24780=ORIENTED_EDGE('',*,*,#17722,.F.);
#24781=ORIENTED_EDGE('',*,*,#17723,.F.);
#24782=ORIENTED_EDGE('',*,*,#17724,.T.);
#24783=ORIENTED_EDGE('',*,*,#17720,.T.);
#24784=ORIENTED_EDGE('',*,*,#17725,.F.);
#24785=ORIENTED_EDGE('',*,*,#17726,.F.);
#24786=ORIENTED_EDGE('',*,*,#17727,.T.);
#24787=ORIENTED_EDGE('',*,*,#17723,.T.);
#24788=ORIENTED_EDGE('',*,*,#17728,.F.);
#24789=ORIENTED_EDGE('',*,*,#17729,.F.);
#24790=ORIENTED_EDGE('',*,*,#17730,.T.);
#24791=ORIENTED_EDGE('',*,*,#17726,.T.);
#24792=ORIENTED_EDGE('',*,*,#17731,.F.);
#24793=ORIENTED_EDGE('',*,*,#17732,.F.);
#24794=ORIENTED_EDGE('',*,*,#17733,.T.);
#24795=ORIENTED_EDGE('',*,*,#17729,.T.);
#24796=ORIENTED_EDGE('',*,*,#17734,.F.);
#24797=ORIENTED_EDGE('',*,*,#17735,.F.);
#24798=ORIENTED_EDGE('',*,*,#17736,.T.);
#24799=ORIENTED_EDGE('',*,*,#17732,.T.);
#24800=ORIENTED_EDGE('',*,*,#17737,.F.);
#24801=ORIENTED_EDGE('',*,*,#17738,.F.);
#24802=ORIENTED_EDGE('',*,*,#17739,.T.);
#24803=ORIENTED_EDGE('',*,*,#17735,.T.);
#24804=ORIENTED_EDGE('',*,*,#17740,.F.);
#24805=ORIENTED_EDGE('',*,*,#17741,.F.);
#24806=ORIENTED_EDGE('',*,*,#17742,.T.);
#24807=ORIENTED_EDGE('',*,*,#17738,.T.);
#24808=ORIENTED_EDGE('',*,*,#17743,.F.);
#24809=ORIENTED_EDGE('',*,*,#17744,.F.);
#24810=ORIENTED_EDGE('',*,*,#17745,.T.);
#24811=ORIENTED_EDGE('',*,*,#17741,.T.);
#24812=ORIENTED_EDGE('',*,*,#17746,.F.);
#24813=ORIENTED_EDGE('',*,*,#17747,.F.);
#24814=ORIENTED_EDGE('',*,*,#17748,.T.);
#24815=ORIENTED_EDGE('',*,*,#17744,.T.);
#24816=ORIENTED_EDGE('',*,*,#17749,.F.);
#24817=ORIENTED_EDGE('',*,*,#17750,.F.);
#24818=ORIENTED_EDGE('',*,*,#17751,.T.);
#24819=ORIENTED_EDGE('',*,*,#17747,.T.);
#24820=ORIENTED_EDGE('',*,*,#17752,.F.);
#24821=ORIENTED_EDGE('',*,*,#17753,.F.);
#24822=ORIENTED_EDGE('',*,*,#17754,.T.);
#24823=ORIENTED_EDGE('',*,*,#17750,.T.);
#24824=ORIENTED_EDGE('',*,*,#17755,.F.);
#24825=ORIENTED_EDGE('',*,*,#17756,.F.);
#24826=ORIENTED_EDGE('',*,*,#17757,.T.);
#24827=ORIENTED_EDGE('',*,*,#17753,.T.);
#24828=ORIENTED_EDGE('',*,*,#17758,.F.);
#24829=ORIENTED_EDGE('',*,*,#17759,.F.);
#24830=ORIENTED_EDGE('',*,*,#17760,.T.);
#24831=ORIENTED_EDGE('',*,*,#17756,.T.);
#24832=ORIENTED_EDGE('',*,*,#17761,.F.);
#24833=ORIENTED_EDGE('',*,*,#17762,.F.);
#24834=ORIENTED_EDGE('',*,*,#17763,.T.);
#24835=ORIENTED_EDGE('',*,*,#17759,.T.);
#24836=ORIENTED_EDGE('',*,*,#17764,.F.);
#24837=ORIENTED_EDGE('',*,*,#17765,.F.);
#24838=ORIENTED_EDGE('',*,*,#17766,.T.);
#24839=ORIENTED_EDGE('',*,*,#17762,.T.);
#24840=ORIENTED_EDGE('',*,*,#17767,.F.);
#24841=ORIENTED_EDGE('',*,*,#17768,.F.);
#24842=ORIENTED_EDGE('',*,*,#17769,.T.);
#24843=ORIENTED_EDGE('',*,*,#17765,.T.);
#24844=ORIENTED_EDGE('',*,*,#17770,.F.);
#24845=ORIENTED_EDGE('',*,*,#17771,.F.);
#24846=ORIENTED_EDGE('',*,*,#17772,.T.);
#24847=ORIENTED_EDGE('',*,*,#17768,.T.);
#24848=ORIENTED_EDGE('',*,*,#17773,.F.);
#24849=ORIENTED_EDGE('',*,*,#17774,.F.);
#24850=ORIENTED_EDGE('',*,*,#17775,.T.);
#24851=ORIENTED_EDGE('',*,*,#17771,.T.);
#24852=ORIENTED_EDGE('',*,*,#17776,.F.);
#24853=ORIENTED_EDGE('',*,*,#17777,.F.);
#24854=ORIENTED_EDGE('',*,*,#17778,.T.);
#24855=ORIENTED_EDGE('',*,*,#17774,.T.);
#24856=ORIENTED_EDGE('',*,*,#17779,.F.);
#24857=ORIENTED_EDGE('',*,*,#17780,.F.);
#24858=ORIENTED_EDGE('',*,*,#17781,.T.);
#24859=ORIENTED_EDGE('',*,*,#17777,.T.);
#24860=ORIENTED_EDGE('',*,*,#17782,.F.);
#24861=ORIENTED_EDGE('',*,*,#17783,.F.);
#24862=ORIENTED_EDGE('',*,*,#17784,.T.);
#24863=ORIENTED_EDGE('',*,*,#17780,.T.);
#24864=ORIENTED_EDGE('',*,*,#17785,.F.);
#24865=ORIENTED_EDGE('',*,*,#17786,.F.);
#24866=ORIENTED_EDGE('',*,*,#17787,.T.);
#24867=ORIENTED_EDGE('',*,*,#17783,.T.);
#24868=ORIENTED_EDGE('',*,*,#17788,.F.);
#24869=ORIENTED_EDGE('',*,*,#17789,.F.);
#24870=ORIENTED_EDGE('',*,*,#17790,.T.);
#24871=ORIENTED_EDGE('',*,*,#17786,.T.);
#24872=ORIENTED_EDGE('',*,*,#17791,.F.);
#24873=ORIENTED_EDGE('',*,*,#17792,.F.);
#24874=ORIENTED_EDGE('',*,*,#17793,.T.);
#24875=ORIENTED_EDGE('',*,*,#17789,.T.);
#24876=ORIENTED_EDGE('',*,*,#17794,.F.);
#24877=ORIENTED_EDGE('',*,*,#17795,.F.);
#24878=ORIENTED_EDGE('',*,*,#17796,.T.);
#24879=ORIENTED_EDGE('',*,*,#17792,.T.);
#24880=ORIENTED_EDGE('',*,*,#17797,.F.);
#24881=ORIENTED_EDGE('',*,*,#17798,.F.);
#24882=ORIENTED_EDGE('',*,*,#17799,.T.);
#24883=ORIENTED_EDGE('',*,*,#17795,.T.);
#24884=ORIENTED_EDGE('',*,*,#17800,.F.);
#24885=ORIENTED_EDGE('',*,*,#17801,.F.);
#24886=ORIENTED_EDGE('',*,*,#17802,.T.);
#24887=ORIENTED_EDGE('',*,*,#17798,.T.);
#24888=ORIENTED_EDGE('',*,*,#17803,.F.);
#24889=ORIENTED_EDGE('',*,*,#17804,.F.);
#24890=ORIENTED_EDGE('',*,*,#17805,.T.);
#24891=ORIENTED_EDGE('',*,*,#17801,.T.);
#24892=ORIENTED_EDGE('',*,*,#17806,.F.);
#24893=ORIENTED_EDGE('',*,*,#17807,.F.);
#24894=ORIENTED_EDGE('',*,*,#17808,.T.);
#24895=ORIENTED_EDGE('',*,*,#17804,.T.);
#24896=ORIENTED_EDGE('',*,*,#17809,.F.);
#24897=ORIENTED_EDGE('',*,*,#17604,.T.);
#24898=ORIENTED_EDGE('',*,*,#17810,.T.);
#24899=ORIENTED_EDGE('',*,*,#17811,.F.);
#24900=ORIENTED_EDGE('',*,*,#17812,.F.);
#24901=ORIENTED_EDGE('',*,*,#17813,.T.);
#24902=ORIENTED_EDGE('',*,*,#17813,.F.);
#24903=ORIENTED_EDGE('',*,*,#17814,.F.);
#24904=ORIENTED_EDGE('',*,*,#17601,.F.);
#24905=ORIENTED_EDGE('',*,*,#17598,.F.);
#24906=ORIENTED_EDGE('',*,*,#17595,.F.);
#24907=ORIENTED_EDGE('',*,*,#17592,.F.);
#24908=ORIENTED_EDGE('',*,*,#17589,.F.);
#24909=ORIENTED_EDGE('',*,*,#17586,.F.);
#24910=ORIENTED_EDGE('',*,*,#17583,.F.);
#24911=ORIENTED_EDGE('',*,*,#17580,.F.);
#24912=ORIENTED_EDGE('',*,*,#17577,.F.);
#24913=ORIENTED_EDGE('',*,*,#17574,.F.);
#24914=ORIENTED_EDGE('',*,*,#17571,.F.);
#24915=ORIENTED_EDGE('',*,*,#17568,.F.);
#24916=ORIENTED_EDGE('',*,*,#17565,.F.);
#24917=ORIENTED_EDGE('',*,*,#17562,.F.);
#24918=ORIENTED_EDGE('',*,*,#17559,.F.);
#24919=ORIENTED_EDGE('',*,*,#17556,.F.);
#24920=ORIENTED_EDGE('',*,*,#17553,.F.);
#24921=ORIENTED_EDGE('',*,*,#17550,.F.);
#24922=ORIENTED_EDGE('',*,*,#17547,.F.);
#24923=ORIENTED_EDGE('',*,*,#17544,.F.);
#24924=ORIENTED_EDGE('',*,*,#17541,.F.);
#24925=ORIENTED_EDGE('',*,*,#17538,.F.);
#24926=ORIENTED_EDGE('',*,*,#17535,.F.);
#24927=ORIENTED_EDGE('',*,*,#17532,.F.);
#24928=ORIENTED_EDGE('',*,*,#17529,.F.);
#24929=ORIENTED_EDGE('',*,*,#17526,.F.);
#24930=ORIENTED_EDGE('',*,*,#17523,.F.);
#24931=ORIENTED_EDGE('',*,*,#17520,.F.);
#24932=ORIENTED_EDGE('',*,*,#17517,.F.);
#24933=ORIENTED_EDGE('',*,*,#17514,.F.);
#24934=ORIENTED_EDGE('',*,*,#17511,.F.);
#24935=ORIENTED_EDGE('',*,*,#17508,.F.);
#24936=ORIENTED_EDGE('',*,*,#17505,.F.);
#24937=ORIENTED_EDGE('',*,*,#17502,.F.);
#24938=ORIENTED_EDGE('',*,*,#17499,.F.);
#24939=ORIENTED_EDGE('',*,*,#17496,.F.);
#24940=ORIENTED_EDGE('',*,*,#17493,.F.);
#24941=ORIENTED_EDGE('',*,*,#17490,.F.);
#24942=ORIENTED_EDGE('',*,*,#17487,.F.);
#24943=ORIENTED_EDGE('',*,*,#17484,.F.);
#24944=ORIENTED_EDGE('',*,*,#17481,.F.);
#24945=ORIENTED_EDGE('',*,*,#17478,.F.);
#24946=ORIENTED_EDGE('',*,*,#17475,.F.);
#24947=ORIENTED_EDGE('',*,*,#17472,.F.);
#24948=ORIENTED_EDGE('',*,*,#17469,.F.);
#24949=ORIENTED_EDGE('',*,*,#17466,.F.);
#24950=ORIENTED_EDGE('',*,*,#17463,.F.);
#24951=ORIENTED_EDGE('',*,*,#17460,.F.);
#24952=ORIENTED_EDGE('',*,*,#17457,.F.);
#24953=ORIENTED_EDGE('',*,*,#17454,.F.);
#24954=ORIENTED_EDGE('',*,*,#17451,.F.);
#24955=ORIENTED_EDGE('',*,*,#17448,.F.);
#24956=ORIENTED_EDGE('',*,*,#17445,.F.);
#24957=ORIENTED_EDGE('',*,*,#17442,.F.);
#24958=ORIENTED_EDGE('',*,*,#17439,.F.);
#24959=ORIENTED_EDGE('',*,*,#17436,.F.);
#24960=ORIENTED_EDGE('',*,*,#17433,.F.);
#24961=ORIENTED_EDGE('',*,*,#17430,.F.);
#24962=ORIENTED_EDGE('',*,*,#17427,.F.);
#24963=ORIENTED_EDGE('',*,*,#17424,.F.);
#24964=ORIENTED_EDGE('',*,*,#17421,.F.);
#24965=ORIENTED_EDGE('',*,*,#17418,.F.);
#24966=ORIENTED_EDGE('',*,*,#17415,.F.);
#24967=ORIENTED_EDGE('',*,*,#17412,.F.);
#24968=ORIENTED_EDGE('',*,*,#17409,.F.);
#24969=ORIENTED_EDGE('',*,*,#17406,.F.);
#24970=ORIENTED_EDGE('',*,*,#17403,.F.);
#24971=ORIENTED_EDGE('',*,*,#17400,.F.);
#24972=ORIENTED_EDGE('',*,*,#17397,.F.);
#24973=ORIENTED_EDGE('',*,*,#17815,.F.);
#24974=ORIENTED_EDGE('',*,*,#17816,.T.);
#24975=ORIENTED_EDGE('',*,*,#17809,.T.);
#24976=ORIENTED_EDGE('',*,*,#17806,.T.);
#24977=ORIENTED_EDGE('',*,*,#17803,.T.);
#24978=ORIENTED_EDGE('',*,*,#17800,.T.);
#24979=ORIENTED_EDGE('',*,*,#17797,.T.);
#24980=ORIENTED_EDGE('',*,*,#17794,.T.);
#24981=ORIENTED_EDGE('',*,*,#17791,.T.);
#24982=ORIENTED_EDGE('',*,*,#17788,.T.);
#24983=ORIENTED_EDGE('',*,*,#17785,.T.);
#24984=ORIENTED_EDGE('',*,*,#17782,.T.);
#24985=ORIENTED_EDGE('',*,*,#17779,.T.);
#24986=ORIENTED_EDGE('',*,*,#17776,.T.);
#24987=ORIENTED_EDGE('',*,*,#17773,.T.);
#24988=ORIENTED_EDGE('',*,*,#17770,.T.);
#24989=ORIENTED_EDGE('',*,*,#17767,.T.);
#24990=ORIENTED_EDGE('',*,*,#17764,.T.);
#24991=ORIENTED_EDGE('',*,*,#17761,.T.);
#24992=ORIENTED_EDGE('',*,*,#17758,.T.);
#24993=ORIENTED_EDGE('',*,*,#17755,.T.);
#24994=ORIENTED_EDGE('',*,*,#17752,.T.);
#24995=ORIENTED_EDGE('',*,*,#17749,.T.);
#24996=ORIENTED_EDGE('',*,*,#17746,.T.);
#24997=ORIENTED_EDGE('',*,*,#17743,.T.);
#24998=ORIENTED_EDGE('',*,*,#17740,.T.);
#24999=ORIENTED_EDGE('',*,*,#17737,.T.);
#25000=ORIENTED_EDGE('',*,*,#17734,.T.);
#25001=ORIENTED_EDGE('',*,*,#17731,.T.);
#25002=ORIENTED_EDGE('',*,*,#17728,.T.);
#25003=ORIENTED_EDGE('',*,*,#17725,.T.);
#25004=ORIENTED_EDGE('',*,*,#17722,.T.);
#25005=ORIENTED_EDGE('',*,*,#17719,.T.);
#25006=ORIENTED_EDGE('',*,*,#17716,.T.);
#25007=ORIENTED_EDGE('',*,*,#17713,.T.);
#25008=ORIENTED_EDGE('',*,*,#17710,.T.);
#25009=ORIENTED_EDGE('',*,*,#17707,.T.);
#25010=ORIENTED_EDGE('',*,*,#17704,.T.);
#25011=ORIENTED_EDGE('',*,*,#17701,.T.);
#25012=ORIENTED_EDGE('',*,*,#17698,.T.);
#25013=ORIENTED_EDGE('',*,*,#17695,.T.);
#25014=ORIENTED_EDGE('',*,*,#17692,.T.);
#25015=ORIENTED_EDGE('',*,*,#17689,.T.);
#25016=ORIENTED_EDGE('',*,*,#17686,.T.);
#25017=ORIENTED_EDGE('',*,*,#17683,.T.);
#25018=ORIENTED_EDGE('',*,*,#17680,.T.);
#25019=ORIENTED_EDGE('',*,*,#17677,.T.);
#25020=ORIENTED_EDGE('',*,*,#17674,.T.);
#25021=ORIENTED_EDGE('',*,*,#17671,.T.);
#25022=ORIENTED_EDGE('',*,*,#17668,.T.);
#25023=ORIENTED_EDGE('',*,*,#17665,.T.);
#25024=ORIENTED_EDGE('',*,*,#17662,.T.);
#25025=ORIENTED_EDGE('',*,*,#17659,.T.);
#25026=ORIENTED_EDGE('',*,*,#17656,.T.);
#25027=ORIENTED_EDGE('',*,*,#17653,.T.);
#25028=ORIENTED_EDGE('',*,*,#17650,.T.);
#25029=ORIENTED_EDGE('',*,*,#17647,.T.);
#25030=ORIENTED_EDGE('',*,*,#17644,.T.);
#25031=ORIENTED_EDGE('',*,*,#17641,.T.);
#25032=ORIENTED_EDGE('',*,*,#17638,.T.);
#25033=ORIENTED_EDGE('',*,*,#17635,.T.);
#25034=ORIENTED_EDGE('',*,*,#17632,.T.);
#25035=ORIENTED_EDGE('',*,*,#17629,.T.);
#25036=ORIENTED_EDGE('',*,*,#17626,.T.);
#25037=ORIENTED_EDGE('',*,*,#17623,.T.);
#25038=ORIENTED_EDGE('',*,*,#17620,.T.);
#25039=ORIENTED_EDGE('',*,*,#17617,.T.);
#25040=ORIENTED_EDGE('',*,*,#17614,.T.);
#25041=ORIENTED_EDGE('',*,*,#17611,.T.);
#25042=ORIENTED_EDGE('',*,*,#17608,.T.);
#25043=ORIENTED_EDGE('',*,*,#17605,.T.);
#25044=ORIENTED_EDGE('',*,*,#17817,.T.);
#25045=ORIENTED_EDGE('',*,*,#17818,.T.);
#25046=ORIENTED_EDGE('',*,*,#17819,.T.);
#25047=ORIENTED_EDGE('',*,*,#17820,.T.);
#25048=ORIENTED_EDGE('',*,*,#17815,.T.);
#25049=ORIENTED_EDGE('',*,*,#17807,.T.);
#25050=ORIENTED_EDGE('',*,*,#17816,.F.);
#25051=ORIENTED_EDGE('',*,*,#17820,.F.);
#25052=ORIENTED_EDGE('',*,*,#17821,.T.);
#25053=ORIENTED_EDGE('',*,*,#17810,.F.);
#25054=ORIENTED_EDGE('',*,*,#17603,.F.);
#25055=ORIENTED_EDGE('',*,*,#17607,.F.);
#25056=ORIENTED_EDGE('',*,*,#17610,.F.);
#25057=ORIENTED_EDGE('',*,*,#17613,.F.);
#25058=ORIENTED_EDGE('',*,*,#17616,.F.);
#25059=ORIENTED_EDGE('',*,*,#17619,.F.);
#25060=ORIENTED_EDGE('',*,*,#17622,.F.);
#25061=ORIENTED_EDGE('',*,*,#17625,.F.);
#25062=ORIENTED_EDGE('',*,*,#17628,.F.);
#25063=ORIENTED_EDGE('',*,*,#17631,.F.);
#25064=ORIENTED_EDGE('',*,*,#17634,.F.);
#25065=ORIENTED_EDGE('',*,*,#17637,.F.);
#25066=ORIENTED_EDGE('',*,*,#17640,.F.);
#25067=ORIENTED_EDGE('',*,*,#17643,.F.);
#25068=ORIENTED_EDGE('',*,*,#17646,.F.);
#25069=ORIENTED_EDGE('',*,*,#17649,.F.);
#25070=ORIENTED_EDGE('',*,*,#17652,.F.);
#25071=ORIENTED_EDGE('',*,*,#17655,.F.);
#25072=ORIENTED_EDGE('',*,*,#17658,.F.);
#25073=ORIENTED_EDGE('',*,*,#17661,.F.);
#25074=ORIENTED_EDGE('',*,*,#17664,.F.);
#25075=ORIENTED_EDGE('',*,*,#17667,.F.);
#25076=ORIENTED_EDGE('',*,*,#17670,.F.);
#25077=ORIENTED_EDGE('',*,*,#17673,.F.);
#25078=ORIENTED_EDGE('',*,*,#17676,.F.);
#25079=ORIENTED_EDGE('',*,*,#17679,.F.);
#25080=ORIENTED_EDGE('',*,*,#17682,.F.);
#25081=ORIENTED_EDGE('',*,*,#17685,.F.);
#25082=ORIENTED_EDGE('',*,*,#17688,.F.);
#25083=ORIENTED_EDGE('',*,*,#17691,.F.);
#25084=ORIENTED_EDGE('',*,*,#17694,.F.);
#25085=ORIENTED_EDGE('',*,*,#17697,.F.);
#25086=ORIENTED_EDGE('',*,*,#17700,.F.);
#25087=ORIENTED_EDGE('',*,*,#17703,.F.);
#25088=ORIENTED_EDGE('',*,*,#17706,.F.);
#25089=ORIENTED_EDGE('',*,*,#17709,.F.);
#25090=ORIENTED_EDGE('',*,*,#17712,.F.);
#25091=ORIENTED_EDGE('',*,*,#17715,.F.);
#25092=ORIENTED_EDGE('',*,*,#17718,.F.);
#25093=ORIENTED_EDGE('',*,*,#17721,.F.);
#25094=ORIENTED_EDGE('',*,*,#17724,.F.);
#25095=ORIENTED_EDGE('',*,*,#17727,.F.);
#25096=ORIENTED_EDGE('',*,*,#17730,.F.);
#25097=ORIENTED_EDGE('',*,*,#17733,.F.);
#25098=ORIENTED_EDGE('',*,*,#17736,.F.);
#25099=ORIENTED_EDGE('',*,*,#17739,.F.);
#25100=ORIENTED_EDGE('',*,*,#17742,.F.);
#25101=ORIENTED_EDGE('',*,*,#17745,.F.);
#25102=ORIENTED_EDGE('',*,*,#17748,.F.);
#25103=ORIENTED_EDGE('',*,*,#17751,.F.);
#25104=ORIENTED_EDGE('',*,*,#17754,.F.);
#25105=ORIENTED_EDGE('',*,*,#17757,.F.);
#25106=ORIENTED_EDGE('',*,*,#17760,.F.);
#25107=ORIENTED_EDGE('',*,*,#17763,.F.);
#25108=ORIENTED_EDGE('',*,*,#17766,.F.);
#25109=ORIENTED_EDGE('',*,*,#17769,.F.);
#25110=ORIENTED_EDGE('',*,*,#17772,.F.);
#25111=ORIENTED_EDGE('',*,*,#17775,.F.);
#25112=ORIENTED_EDGE('',*,*,#17778,.F.);
#25113=ORIENTED_EDGE('',*,*,#17781,.F.);
#25114=ORIENTED_EDGE('',*,*,#17784,.F.);
#25115=ORIENTED_EDGE('',*,*,#17787,.F.);
#25116=ORIENTED_EDGE('',*,*,#17790,.F.);
#25117=ORIENTED_EDGE('',*,*,#17793,.F.);
#25118=ORIENTED_EDGE('',*,*,#17796,.F.);
#25119=ORIENTED_EDGE('',*,*,#17799,.F.);
#25120=ORIENTED_EDGE('',*,*,#17802,.F.);
#25121=ORIENTED_EDGE('',*,*,#17805,.F.);
#25122=ORIENTED_EDGE('',*,*,#17808,.F.);
#25123=ORIENTED_EDGE('',*,*,#17821,.F.);
#25124=ORIENTED_EDGE('',*,*,#17819,.F.);
#25125=ORIENTED_EDGE('',*,*,#17395,.F.);
#25126=ORIENTED_EDGE('',*,*,#17399,.F.);
#25127=ORIENTED_EDGE('',*,*,#17402,.F.);
#25128=ORIENTED_EDGE('',*,*,#17405,.F.);
#25129=ORIENTED_EDGE('',*,*,#17408,.F.);
#25130=ORIENTED_EDGE('',*,*,#17411,.F.);
#25131=ORIENTED_EDGE('',*,*,#17414,.F.);
#25132=ORIENTED_EDGE('',*,*,#17417,.F.);
#25133=ORIENTED_EDGE('',*,*,#17420,.F.);
#25134=ORIENTED_EDGE('',*,*,#17423,.F.);
#25135=ORIENTED_EDGE('',*,*,#17426,.F.);
#25136=ORIENTED_EDGE('',*,*,#17429,.F.);
#25137=ORIENTED_EDGE('',*,*,#17432,.F.);
#25138=ORIENTED_EDGE('',*,*,#17435,.F.);
#25139=ORIENTED_EDGE('',*,*,#17438,.F.);
#25140=ORIENTED_EDGE('',*,*,#17441,.F.);
#25141=ORIENTED_EDGE('',*,*,#17444,.F.);
#25142=ORIENTED_EDGE('',*,*,#17447,.F.);
#25143=ORIENTED_EDGE('',*,*,#17450,.F.);
#25144=ORIENTED_EDGE('',*,*,#17453,.F.);
#25145=ORIENTED_EDGE('',*,*,#17456,.F.);
#25146=ORIENTED_EDGE('',*,*,#17459,.F.);
#25147=ORIENTED_EDGE('',*,*,#17462,.F.);
#25148=ORIENTED_EDGE('',*,*,#17465,.F.);
#25149=ORIENTED_EDGE('',*,*,#17468,.F.);
#25150=ORIENTED_EDGE('',*,*,#17471,.F.);
#25151=ORIENTED_EDGE('',*,*,#17474,.F.);
#25152=ORIENTED_EDGE('',*,*,#17477,.F.);
#25153=ORIENTED_EDGE('',*,*,#17480,.F.);
#25154=ORIENTED_EDGE('',*,*,#17483,.F.);
#25155=ORIENTED_EDGE('',*,*,#17486,.F.);
#25156=ORIENTED_EDGE('',*,*,#17489,.F.);
#25157=ORIENTED_EDGE('',*,*,#17492,.F.);
#25158=ORIENTED_EDGE('',*,*,#17495,.F.);
#25159=ORIENTED_EDGE('',*,*,#17498,.F.);
#25160=ORIENTED_EDGE('',*,*,#17501,.F.);
#25161=ORIENTED_EDGE('',*,*,#17504,.F.);
#25162=ORIENTED_EDGE('',*,*,#17507,.F.);
#25163=ORIENTED_EDGE('',*,*,#17510,.F.);
#25164=ORIENTED_EDGE('',*,*,#17513,.F.);
#25165=ORIENTED_EDGE('',*,*,#17516,.F.);
#25166=ORIENTED_EDGE('',*,*,#17519,.F.);
#25167=ORIENTED_EDGE('',*,*,#17522,.F.);
#25168=ORIENTED_EDGE('',*,*,#17525,.F.);
#25169=ORIENTED_EDGE('',*,*,#17528,.F.);
#25170=ORIENTED_EDGE('',*,*,#17531,.F.);
#25171=ORIENTED_EDGE('',*,*,#17534,.F.);
#25172=ORIENTED_EDGE('',*,*,#17537,.F.);
#25173=ORIENTED_EDGE('',*,*,#17540,.F.);
#25174=ORIENTED_EDGE('',*,*,#17543,.F.);
#25175=ORIENTED_EDGE('',*,*,#17546,.F.);
#25176=ORIENTED_EDGE('',*,*,#17549,.F.);
#25177=ORIENTED_EDGE('',*,*,#17552,.F.);
#25178=ORIENTED_EDGE('',*,*,#17555,.F.);
#25179=ORIENTED_EDGE('',*,*,#17558,.F.);
#25180=ORIENTED_EDGE('',*,*,#17561,.F.);
#25181=ORIENTED_EDGE('',*,*,#17564,.F.);
#25182=ORIENTED_EDGE('',*,*,#17567,.F.);
#25183=ORIENTED_EDGE('',*,*,#17570,.F.);
#25184=ORIENTED_EDGE('',*,*,#17573,.F.);
#25185=ORIENTED_EDGE('',*,*,#17576,.F.);
#25186=ORIENTED_EDGE('',*,*,#17579,.F.);
#25187=ORIENTED_EDGE('',*,*,#17582,.F.);
#25188=ORIENTED_EDGE('',*,*,#17585,.F.);
#25189=ORIENTED_EDGE('',*,*,#17588,.F.);
#25190=ORIENTED_EDGE('',*,*,#17591,.F.);
#25191=ORIENTED_EDGE('',*,*,#17594,.F.);
#25192=ORIENTED_EDGE('',*,*,#17597,.F.);
#25193=ORIENTED_EDGE('',*,*,#17600,.F.);
#25194=ORIENTED_EDGE('',*,*,#17822,.F.);
#25195=ORIENTED_EDGE('',*,*,#17812,.T.);
#25196=ORIENTED_EDGE('',*,*,#17823,.T.);
#25197=ORIENTED_EDGE('',*,*,#17824,.T.);
#25198=ORIENTED_EDGE('',*,*,#17823,.F.);
#25199=ORIENTED_EDGE('',*,*,#17811,.T.);
#25200=ORIENTED_EDGE('',*,*,#17825,.T.);
#25201=ORIENTED_EDGE('',*,*,#17599,.T.);
#25202=ORIENTED_EDGE('',*,*,#17814,.T.);
#25203=ORIENTED_EDGE('',*,*,#17825,.F.);
#25204=ORIENTED_EDGE('',*,*,#17822,.T.);
#25205=ORIENTED_EDGE('',*,*,#17826,.F.);
#25206=ORIENTED_EDGE('',*,*,#17824,.F.);
#25207=ORIENTED_EDGE('',*,*,#17827,.F.);
#25208=ORIENTED_EDGE('',*,*,#17828,.T.);
#25209=ORIENTED_EDGE('',*,*,#17829,.F.);
#25210=ORIENTED_EDGE('',*,*,#17830,.F.);
#25211=ORIENTED_EDGE('',*,*,#17831,.F.);
#25212=ORIENTED_EDGE('',*,*,#17830,.T.);
#25213=ORIENTED_EDGE('',*,*,#17832,.T.);
#25214=ORIENTED_EDGE('',*,*,#17833,.F.);
#25215=ORIENTED_EDGE('',*,*,#17832,.F.);
#25216=ORIENTED_EDGE('',*,*,#17829,.T.);
#25217=ORIENTED_EDGE('',*,*,#17834,.T.);
#25218=ORIENTED_EDGE('',*,*,#17835,.F.);
#25219=ORIENTED_EDGE('',*,*,#17834,.F.);
#25220=ORIENTED_EDGE('',*,*,#17828,.F.);
#25221=ORIENTED_EDGE('',*,*,#17836,.F.);
#25222=ORIENTED_EDGE('',*,*,#17837,.T.);
#25223=ORIENTED_EDGE('',*,*,#17838,.F.);
#25224=ORIENTED_EDGE('',*,*,#17839,.F.);
#25225=ORIENTED_EDGE('',*,*,#17840,.F.);
#25226=ORIENTED_EDGE('',*,*,#17839,.T.);
#25227=ORIENTED_EDGE('',*,*,#17841,.T.);
#25228=ORIENTED_EDGE('',*,*,#17842,.F.);
#25229=ORIENTED_EDGE('',*,*,#17841,.F.);
#25230=ORIENTED_EDGE('',*,*,#17838,.T.);
#25231=ORIENTED_EDGE('',*,*,#17843,.T.);
#25232=ORIENTED_EDGE('',*,*,#17844,.F.);
#25233=ORIENTED_EDGE('',*,*,#17843,.F.);
#25234=ORIENTED_EDGE('',*,*,#17837,.F.);
#25235=ORIENTED_EDGE('',*,*,#17845,.F.);
#25236=ORIENTED_EDGE('',*,*,#17846,.T.);
#25237=ORIENTED_EDGE('',*,*,#17847,.F.);
#25238=ORIENTED_EDGE('',*,*,#17848,.F.);
#25239=ORIENTED_EDGE('',*,*,#17849,.F.);
#25240=ORIENTED_EDGE('',*,*,#17848,.T.);
#25241=ORIENTED_EDGE('',*,*,#17850,.T.);
#25242=ORIENTED_EDGE('',*,*,#17851,.F.);
#25243=ORIENTED_EDGE('',*,*,#17850,.F.);
#25244=ORIENTED_EDGE('',*,*,#17847,.T.);
#25245=ORIENTED_EDGE('',*,*,#17852,.T.);
#25246=ORIENTED_EDGE('',*,*,#17853,.F.);
#25247=ORIENTED_EDGE('',*,*,#17852,.F.);
#25248=ORIENTED_EDGE('',*,*,#17846,.F.);
#25249=ORIENTED_EDGE('',*,*,#17854,.F.);
#25250=ORIENTED_EDGE('',*,*,#17855,.T.);
#25251=ORIENTED_EDGE('',*,*,#17856,.F.);
#25252=ORIENTED_EDGE('',*,*,#17857,.F.);
#25253=ORIENTED_EDGE('',*,*,#17858,.F.);
#25254=ORIENTED_EDGE('',*,*,#17857,.T.);
#25255=ORIENTED_EDGE('',*,*,#17859,.T.);
#25256=ORIENTED_EDGE('',*,*,#17860,.F.);
#25257=ORIENTED_EDGE('',*,*,#17859,.F.);
#25258=ORIENTED_EDGE('',*,*,#17856,.T.);
#25259=ORIENTED_EDGE('',*,*,#17861,.T.);
#25260=ORIENTED_EDGE('',*,*,#17862,.F.);
#25261=ORIENTED_EDGE('',*,*,#17861,.F.);
#25262=ORIENTED_EDGE('',*,*,#17855,.F.);
#25263=ORIENTED_EDGE('',*,*,#17863,.F.);
#25264=ORIENTED_EDGE('',*,*,#17864,.T.);
#25265=ORIENTED_EDGE('',*,*,#17865,.F.);
#25266=ORIENTED_EDGE('',*,*,#17866,.F.);
#25267=ORIENTED_EDGE('',*,*,#17867,.F.);
#25268=ORIENTED_EDGE('',*,*,#17866,.T.);
#25269=ORIENTED_EDGE('',*,*,#17868,.T.);
#25270=ORIENTED_EDGE('',*,*,#17869,.F.);
#25271=ORIENTED_EDGE('',*,*,#17868,.F.);
#25272=ORIENTED_EDGE('',*,*,#17865,.T.);
#25273=ORIENTED_EDGE('',*,*,#17870,.T.);
#25274=ORIENTED_EDGE('',*,*,#17871,.F.);
#25275=ORIENTED_EDGE('',*,*,#17870,.F.);
#25276=ORIENTED_EDGE('',*,*,#17864,.F.);
#25277=ORIENTED_EDGE('',*,*,#17872,.F.);
#25278=ORIENTED_EDGE('',*,*,#17873,.T.);
#25279=ORIENTED_EDGE('',*,*,#17874,.F.);
#25280=ORIENTED_EDGE('',*,*,#17875,.F.);
#25281=ORIENTED_EDGE('',*,*,#17876,.F.);
#25282=ORIENTED_EDGE('',*,*,#17875,.T.);
#25283=ORIENTED_EDGE('',*,*,#17877,.T.);
#25284=ORIENTED_EDGE('',*,*,#17878,.F.);
#25285=ORIENTED_EDGE('',*,*,#17877,.F.);
#25286=ORIENTED_EDGE('',*,*,#17874,.T.);
#25287=ORIENTED_EDGE('',*,*,#17879,.T.);
#25288=ORIENTED_EDGE('',*,*,#17880,.F.);
#25289=ORIENTED_EDGE('',*,*,#17879,.F.);
#25290=ORIENTED_EDGE('',*,*,#17873,.F.);
#25291=ORIENTED_EDGE('',*,*,#17881,.F.);
#25292=ORIENTED_EDGE('',*,*,#17882,.T.);
#25293=ORIENTED_EDGE('',*,*,#17883,.F.);
#25294=ORIENTED_EDGE('',*,*,#17884,.F.);
#25295=ORIENTED_EDGE('',*,*,#17885,.F.);
#25296=ORIENTED_EDGE('',*,*,#17884,.T.);
#25297=ORIENTED_EDGE('',*,*,#17886,.T.);
#25298=ORIENTED_EDGE('',*,*,#17887,.F.);
#25299=ORIENTED_EDGE('',*,*,#17886,.F.);
#25300=ORIENTED_EDGE('',*,*,#17883,.T.);
#25301=ORIENTED_EDGE('',*,*,#17888,.T.);
#25302=ORIENTED_EDGE('',*,*,#17889,.F.);
#25303=ORIENTED_EDGE('',*,*,#17888,.F.);
#25304=ORIENTED_EDGE('',*,*,#17882,.F.);
#25305=ORIENTED_EDGE('',*,*,#17890,.F.);
#25306=ORIENTED_EDGE('',*,*,#17891,.T.);
#25307=ORIENTED_EDGE('',*,*,#17892,.F.);
#25308=ORIENTED_EDGE('',*,*,#17893,.F.);
#25309=ORIENTED_EDGE('',*,*,#17894,.F.);
#25310=ORIENTED_EDGE('',*,*,#17893,.T.);
#25311=ORIENTED_EDGE('',*,*,#17895,.T.);
#25312=ORIENTED_EDGE('',*,*,#17896,.F.);
#25313=ORIENTED_EDGE('',*,*,#17895,.F.);
#25314=ORIENTED_EDGE('',*,*,#17892,.T.);
#25315=ORIENTED_EDGE('',*,*,#17897,.T.);
#25316=ORIENTED_EDGE('',*,*,#17898,.F.);
#25317=ORIENTED_EDGE('',*,*,#17897,.F.);
#25318=ORIENTED_EDGE('',*,*,#17891,.F.);
#25319=ORIENTED_EDGE('',*,*,#17899,.F.);
#25320=ORIENTED_EDGE('',*,*,#17900,.T.);
#25321=ORIENTED_EDGE('',*,*,#17901,.F.);
#25322=ORIENTED_EDGE('',*,*,#17902,.F.);
#25323=ORIENTED_EDGE('',*,*,#17903,.F.);
#25324=ORIENTED_EDGE('',*,*,#17902,.T.);
#25325=ORIENTED_EDGE('',*,*,#17904,.T.);
#25326=ORIENTED_EDGE('',*,*,#17905,.F.);
#25327=ORIENTED_EDGE('',*,*,#17904,.F.);
#25328=ORIENTED_EDGE('',*,*,#17901,.T.);
#25329=ORIENTED_EDGE('',*,*,#17906,.T.);
#25330=ORIENTED_EDGE('',*,*,#17907,.F.);
#25331=ORIENTED_EDGE('',*,*,#17906,.F.);
#25332=ORIENTED_EDGE('',*,*,#17900,.F.);
#25333=ORIENTED_EDGE('',*,*,#17908,.F.);
#25334=ORIENTED_EDGE('',*,*,#17909,.T.);
#25335=ORIENTED_EDGE('',*,*,#17910,.F.);
#25336=ORIENTED_EDGE('',*,*,#17911,.F.);
#25337=ORIENTED_EDGE('',*,*,#17912,.F.);
#25338=ORIENTED_EDGE('',*,*,#17911,.T.);
#25339=ORIENTED_EDGE('',*,*,#17913,.T.);
#25340=ORIENTED_EDGE('',*,*,#17914,.F.);
#25341=ORIENTED_EDGE('',*,*,#17913,.F.);
#25342=ORIENTED_EDGE('',*,*,#17910,.T.);
#25343=ORIENTED_EDGE('',*,*,#17915,.T.);
#25344=ORIENTED_EDGE('',*,*,#17916,.F.);
#25345=ORIENTED_EDGE('',*,*,#17915,.F.);
#25346=ORIENTED_EDGE('',*,*,#17909,.F.);
#25347=ORIENTED_EDGE('',*,*,#17917,.F.);
#25348=ORIENTED_EDGE('',*,*,#17918,.T.);
#25349=ORIENTED_EDGE('',*,*,#17919,.F.);
#25350=ORIENTED_EDGE('',*,*,#17920,.F.);
#25351=ORIENTED_EDGE('',*,*,#17921,.F.);
#25352=ORIENTED_EDGE('',*,*,#17920,.T.);
#25353=ORIENTED_EDGE('',*,*,#17922,.T.);
#25354=ORIENTED_EDGE('',*,*,#17923,.F.);
#25355=ORIENTED_EDGE('',*,*,#17922,.F.);
#25356=ORIENTED_EDGE('',*,*,#17919,.T.);
#25357=ORIENTED_EDGE('',*,*,#17924,.T.);
#25358=ORIENTED_EDGE('',*,*,#17925,.F.);
#25359=ORIENTED_EDGE('',*,*,#17924,.F.);
#25360=ORIENTED_EDGE('',*,*,#17918,.F.);
#25361=ORIENTED_EDGE('',*,*,#17926,.F.);
#25362=ORIENTED_EDGE('',*,*,#17927,.T.);
#25363=ORIENTED_EDGE('',*,*,#17928,.F.);
#25364=ORIENTED_EDGE('',*,*,#17929,.F.);
#25365=ORIENTED_EDGE('',*,*,#17930,.F.);
#25366=ORIENTED_EDGE('',*,*,#17929,.T.);
#25367=ORIENTED_EDGE('',*,*,#17931,.T.);
#25368=ORIENTED_EDGE('',*,*,#17932,.F.);
#25369=ORIENTED_EDGE('',*,*,#17931,.F.);
#25370=ORIENTED_EDGE('',*,*,#17928,.T.);
#25371=ORIENTED_EDGE('',*,*,#17933,.T.);
#25372=ORIENTED_EDGE('',*,*,#17934,.F.);
#25373=ORIENTED_EDGE('',*,*,#17933,.F.);
#25374=ORIENTED_EDGE('',*,*,#17927,.F.);
#25375=ORIENTED_EDGE('',*,*,#17935,.F.);
#25376=ORIENTED_EDGE('',*,*,#17936,.T.);
#25377=ORIENTED_EDGE('',*,*,#17937,.F.);
#25378=ORIENTED_EDGE('',*,*,#17938,.F.);
#25379=ORIENTED_EDGE('',*,*,#17939,.F.);
#25380=ORIENTED_EDGE('',*,*,#17938,.T.);
#25381=ORIENTED_EDGE('',*,*,#17940,.T.);
#25382=ORIENTED_EDGE('',*,*,#17941,.F.);
#25383=ORIENTED_EDGE('',*,*,#17940,.F.);
#25384=ORIENTED_EDGE('',*,*,#17937,.T.);
#25385=ORIENTED_EDGE('',*,*,#17942,.T.);
#25386=ORIENTED_EDGE('',*,*,#17943,.F.);
#25387=ORIENTED_EDGE('',*,*,#17942,.F.);
#25388=ORIENTED_EDGE('',*,*,#17936,.F.);
#25389=ORIENTED_EDGE('',*,*,#17944,.F.);
#25390=ORIENTED_EDGE('',*,*,#17945,.T.);
#25391=ORIENTED_EDGE('',*,*,#17946,.F.);
#25392=ORIENTED_EDGE('',*,*,#17947,.F.);
#25393=ORIENTED_EDGE('',*,*,#17948,.F.);
#25394=ORIENTED_EDGE('',*,*,#17947,.T.);
#25395=ORIENTED_EDGE('',*,*,#17949,.T.);
#25396=ORIENTED_EDGE('',*,*,#17950,.F.);
#25397=ORIENTED_EDGE('',*,*,#17949,.F.);
#25398=ORIENTED_EDGE('',*,*,#17946,.T.);
#25399=ORIENTED_EDGE('',*,*,#17951,.T.);
#25400=ORIENTED_EDGE('',*,*,#17952,.F.);
#25401=ORIENTED_EDGE('',*,*,#17951,.F.);
#25402=ORIENTED_EDGE('',*,*,#17945,.F.);
#25403=ORIENTED_EDGE('',*,*,#17953,.F.);
#25404=ORIENTED_EDGE('',*,*,#17954,.T.);
#25405=ORIENTED_EDGE('',*,*,#17955,.F.);
#25406=ORIENTED_EDGE('',*,*,#17956,.F.);
#25407=ORIENTED_EDGE('',*,*,#17957,.F.);
#25408=ORIENTED_EDGE('',*,*,#17956,.T.);
#25409=ORIENTED_EDGE('',*,*,#17958,.T.);
#25410=ORIENTED_EDGE('',*,*,#17959,.F.);
#25411=ORIENTED_EDGE('',*,*,#17958,.F.);
#25412=ORIENTED_EDGE('',*,*,#17955,.T.);
#25413=ORIENTED_EDGE('',*,*,#17960,.T.);
#25414=ORIENTED_EDGE('',*,*,#17961,.F.);
#25415=ORIENTED_EDGE('',*,*,#17960,.F.);
#25416=ORIENTED_EDGE('',*,*,#17954,.F.);
#25417=ORIENTED_EDGE('',*,*,#17962,.F.);
#25418=ORIENTED_EDGE('',*,*,#17963,.T.);
#25419=ORIENTED_EDGE('',*,*,#17964,.F.);
#25420=ORIENTED_EDGE('',*,*,#17965,.F.);
#25421=ORIENTED_EDGE('',*,*,#17966,.F.);
#25422=ORIENTED_EDGE('',*,*,#17965,.T.);
#25423=ORIENTED_EDGE('',*,*,#17967,.T.);
#25424=ORIENTED_EDGE('',*,*,#17968,.F.);
#25425=ORIENTED_EDGE('',*,*,#17967,.F.);
#25426=ORIENTED_EDGE('',*,*,#17964,.T.);
#25427=ORIENTED_EDGE('',*,*,#17969,.T.);
#25428=ORIENTED_EDGE('',*,*,#17970,.F.);
#25429=ORIENTED_EDGE('',*,*,#17969,.F.);
#25430=ORIENTED_EDGE('',*,*,#17963,.F.);
#25431=ORIENTED_EDGE('',*,*,#17971,.F.);
#25432=ORIENTED_EDGE('',*,*,#17972,.T.);
#25433=ORIENTED_EDGE('',*,*,#17973,.F.);
#25434=ORIENTED_EDGE('',*,*,#17974,.F.);
#25435=ORIENTED_EDGE('',*,*,#17975,.F.);
#25436=ORIENTED_EDGE('',*,*,#17974,.T.);
#25437=ORIENTED_EDGE('',*,*,#17976,.T.);
#25438=ORIENTED_EDGE('',*,*,#17977,.F.);
#25439=ORIENTED_EDGE('',*,*,#17976,.F.);
#25440=ORIENTED_EDGE('',*,*,#17973,.T.);
#25441=ORIENTED_EDGE('',*,*,#17978,.T.);
#25442=ORIENTED_EDGE('',*,*,#17979,.F.);
#25443=ORIENTED_EDGE('',*,*,#17978,.F.);
#25444=ORIENTED_EDGE('',*,*,#17972,.F.);
#25445=ORIENTED_EDGE('',*,*,#17980,.F.);
#25446=ORIENTED_EDGE('',*,*,#17981,.T.);
#25447=ORIENTED_EDGE('',*,*,#17982,.F.);
#25448=ORIENTED_EDGE('',*,*,#17983,.F.);
#25449=ORIENTED_EDGE('',*,*,#17984,.F.);
#25450=ORIENTED_EDGE('',*,*,#17983,.T.);
#25451=ORIENTED_EDGE('',*,*,#17985,.T.);
#25452=ORIENTED_EDGE('',*,*,#17986,.F.);
#25453=ORIENTED_EDGE('',*,*,#17987,.F.);
#25454=ORIENTED_EDGE('',*,*,#17985,.F.);
#25455=ORIENTED_EDGE('',*,*,#17982,.T.);
#25456=ORIENTED_EDGE('',*,*,#17988,.T.);
#25457=ORIENTED_EDGE('',*,*,#17989,.F.);
#25458=ORIENTED_EDGE('',*,*,#17988,.F.);
#25459=ORIENTED_EDGE('',*,*,#17981,.F.);
#25460=ORIENTED_EDGE('',*,*,#17990,.F.);
#25461=ORIENTED_EDGE('',*,*,#17991,.F.);
#25462=ORIENTED_EDGE('',*,*,#17992,.T.);
#25463=ORIENTED_EDGE('',*,*,#17993,.F.);
#25464=ORIENTED_EDGE('',*,*,#17994,.F.);
#25465=ORIENTED_EDGE('',*,*,#17995,.F.);
#25466=ORIENTED_EDGE('',*,*,#17994,.T.);
#25467=ORIENTED_EDGE('',*,*,#17996,.T.);
#25468=ORIENTED_EDGE('',*,*,#17997,.F.);
#25469=ORIENTED_EDGE('',*,*,#17996,.F.);
#25470=ORIENTED_EDGE('',*,*,#17993,.T.);
#25471=ORIENTED_EDGE('',*,*,#17998,.T.);
#25472=ORIENTED_EDGE('',*,*,#17999,.F.);
#25473=ORIENTED_EDGE('',*,*,#17998,.F.);
#25474=ORIENTED_EDGE('',*,*,#17992,.F.);
#25475=ORIENTED_EDGE('',*,*,#18000,.F.);
#25476=ORIENTED_EDGE('',*,*,#18001,.T.);
#25477=ORIENTED_EDGE('',*,*,#18002,.F.);
#25478=ORIENTED_EDGE('',*,*,#18003,.F.);
#25479=ORIENTED_EDGE('',*,*,#18004,.F.);
#25480=ORIENTED_EDGE('',*,*,#18003,.T.);
#25481=ORIENTED_EDGE('',*,*,#18005,.T.);
#25482=ORIENTED_EDGE('',*,*,#18006,.F.);
#25483=ORIENTED_EDGE('',*,*,#18005,.F.);
#25484=ORIENTED_EDGE('',*,*,#18002,.T.);
#25485=ORIENTED_EDGE('',*,*,#18007,.T.);
#25486=ORIENTED_EDGE('',*,*,#18008,.F.);
#25487=ORIENTED_EDGE('',*,*,#18007,.F.);
#25488=ORIENTED_EDGE('',*,*,#18001,.F.);
#25489=ORIENTED_EDGE('',*,*,#18009,.F.);
#25490=ORIENTED_EDGE('',*,*,#18010,.T.);
#25491=ORIENTED_EDGE('',*,*,#18011,.F.);
#25492=ORIENTED_EDGE('',*,*,#18012,.F.);
#25493=ORIENTED_EDGE('',*,*,#18013,.F.);
#25494=ORIENTED_EDGE('',*,*,#18012,.T.);
#25495=ORIENTED_EDGE('',*,*,#18014,.T.);
#25496=ORIENTED_EDGE('',*,*,#18015,.F.);
#25497=ORIENTED_EDGE('',*,*,#18014,.F.);
#25498=ORIENTED_EDGE('',*,*,#18011,.T.);
#25499=ORIENTED_EDGE('',*,*,#18016,.T.);
#25500=ORIENTED_EDGE('',*,*,#18017,.F.);
#25501=ORIENTED_EDGE('',*,*,#18016,.F.);
#25502=ORIENTED_EDGE('',*,*,#18010,.F.);
#25503=ORIENTED_EDGE('',*,*,#18018,.F.);
#25504=ORIENTED_EDGE('',*,*,#18019,.T.);
#25505=ORIENTED_EDGE('',*,*,#18020,.F.);
#25506=ORIENTED_EDGE('',*,*,#18021,.F.);
#25507=ORIENTED_EDGE('',*,*,#18022,.F.);
#25508=ORIENTED_EDGE('',*,*,#18021,.T.);
#25509=ORIENTED_EDGE('',*,*,#18023,.T.);
#25510=ORIENTED_EDGE('',*,*,#18024,.F.);
#25511=ORIENTED_EDGE('',*,*,#18023,.F.);
#25512=ORIENTED_EDGE('',*,*,#18020,.T.);
#25513=ORIENTED_EDGE('',*,*,#18025,.T.);
#25514=ORIENTED_EDGE('',*,*,#18026,.F.);
#25515=ORIENTED_EDGE('',*,*,#18025,.F.);
#25516=ORIENTED_EDGE('',*,*,#18019,.F.);
#25517=ORIENTED_EDGE('',*,*,#18027,.F.);
#25518=ORIENTED_EDGE('',*,*,#18028,.T.);
#25519=ORIENTED_EDGE('',*,*,#18029,.F.);
#25520=ORIENTED_EDGE('',*,*,#18030,.F.);
#25521=ORIENTED_EDGE('',*,*,#18031,.F.);
#25522=ORIENTED_EDGE('',*,*,#18030,.T.);
#25523=ORIENTED_EDGE('',*,*,#18032,.T.);
#25524=ORIENTED_EDGE('',*,*,#18033,.F.);
#25525=ORIENTED_EDGE('',*,*,#18032,.F.);
#25526=ORIENTED_EDGE('',*,*,#18029,.T.);
#25527=ORIENTED_EDGE('',*,*,#18034,.T.);
#25528=ORIENTED_EDGE('',*,*,#18035,.F.);
#25529=ORIENTED_EDGE('',*,*,#18034,.F.);
#25530=ORIENTED_EDGE('',*,*,#18028,.F.);
#25531=ORIENTED_EDGE('',*,*,#18036,.F.);
#25532=ORIENTED_EDGE('',*,*,#18037,.T.);
#25533=ORIENTED_EDGE('',*,*,#18038,.F.);
#25534=ORIENTED_EDGE('',*,*,#18039,.F.);
#25535=ORIENTED_EDGE('',*,*,#18040,.F.);
#25536=ORIENTED_EDGE('',*,*,#18039,.T.);
#25537=ORIENTED_EDGE('',*,*,#18041,.T.);
#25538=ORIENTED_EDGE('',*,*,#18042,.F.);
#25539=ORIENTED_EDGE('',*,*,#18041,.F.);
#25540=ORIENTED_EDGE('',*,*,#18038,.T.);
#25541=ORIENTED_EDGE('',*,*,#18043,.T.);
#25542=ORIENTED_EDGE('',*,*,#18044,.F.);
#25543=ORIENTED_EDGE('',*,*,#18043,.F.);
#25544=ORIENTED_EDGE('',*,*,#18037,.F.);
#25545=ORIENTED_EDGE('',*,*,#18045,.F.);
#25546=ORIENTED_EDGE('',*,*,#18046,.T.);
#25547=ORIENTED_EDGE('',*,*,#18047,.F.);
#25548=ORIENTED_EDGE('',*,*,#18048,.F.);
#25549=ORIENTED_EDGE('',*,*,#18049,.F.);
#25550=ORIENTED_EDGE('',*,*,#18048,.T.);
#25551=ORIENTED_EDGE('',*,*,#18050,.T.);
#25552=ORIENTED_EDGE('',*,*,#18051,.F.);
#25553=ORIENTED_EDGE('',*,*,#18050,.F.);
#25554=ORIENTED_EDGE('',*,*,#18047,.T.);
#25555=ORIENTED_EDGE('',*,*,#18052,.T.);
#25556=ORIENTED_EDGE('',*,*,#18053,.F.);
#25557=ORIENTED_EDGE('',*,*,#18052,.F.);
#25558=ORIENTED_EDGE('',*,*,#18046,.F.);
#25559=ORIENTED_EDGE('',*,*,#18054,.F.);
#25560=ORIENTED_EDGE('',*,*,#18055,.T.);
#25561=ORIENTED_EDGE('',*,*,#18056,.F.);
#25562=ORIENTED_EDGE('',*,*,#18057,.F.);
#25563=ORIENTED_EDGE('',*,*,#18058,.F.);
#25564=ORIENTED_EDGE('',*,*,#18057,.T.);
#25565=ORIENTED_EDGE('',*,*,#18059,.T.);
#25566=ORIENTED_EDGE('',*,*,#18060,.F.);
#25567=ORIENTED_EDGE('',*,*,#18059,.F.);
#25568=ORIENTED_EDGE('',*,*,#18056,.T.);
#25569=ORIENTED_EDGE('',*,*,#18061,.T.);
#25570=ORIENTED_EDGE('',*,*,#18062,.F.);
#25571=ORIENTED_EDGE('',*,*,#18061,.F.);
#25572=ORIENTED_EDGE('',*,*,#18055,.F.);
#25573=ORIENTED_EDGE('',*,*,#18063,.F.);
#25574=ORIENTED_EDGE('',*,*,#18064,.T.);
#25575=ORIENTED_EDGE('',*,*,#18065,.F.);
#25576=ORIENTED_EDGE('',*,*,#18066,.F.);
#25577=ORIENTED_EDGE('',*,*,#18067,.F.);
#25578=ORIENTED_EDGE('',*,*,#18066,.T.);
#25579=ORIENTED_EDGE('',*,*,#18068,.T.);
#25580=ORIENTED_EDGE('',*,*,#18069,.F.);
#25581=ORIENTED_EDGE('',*,*,#18068,.F.);
#25582=ORIENTED_EDGE('',*,*,#18065,.T.);
#25583=ORIENTED_EDGE('',*,*,#18070,.T.);
#25584=ORIENTED_EDGE('',*,*,#18071,.F.);
#25585=ORIENTED_EDGE('',*,*,#18070,.F.);
#25586=ORIENTED_EDGE('',*,*,#18064,.F.);
#25587=ORIENTED_EDGE('',*,*,#18072,.F.);
#25588=ORIENTED_EDGE('',*,*,#18073,.T.);
#25589=ORIENTED_EDGE('',*,*,#18074,.F.);
#25590=ORIENTED_EDGE('',*,*,#18075,.F.);
#25591=ORIENTED_EDGE('',*,*,#18076,.F.);
#25592=ORIENTED_EDGE('',*,*,#18075,.T.);
#25593=ORIENTED_EDGE('',*,*,#18077,.T.);
#25594=ORIENTED_EDGE('',*,*,#18078,.F.);
#25595=ORIENTED_EDGE('',*,*,#18077,.F.);
#25596=ORIENTED_EDGE('',*,*,#18074,.T.);
#25597=ORIENTED_EDGE('',*,*,#18079,.T.);
#25598=ORIENTED_EDGE('',*,*,#18080,.F.);
#25599=ORIENTED_EDGE('',*,*,#18079,.F.);
#25600=ORIENTED_EDGE('',*,*,#18073,.F.);
#25601=ORIENTED_EDGE('',*,*,#18081,.F.);
#25602=ORIENTED_EDGE('',*,*,#18082,.T.);
#25603=ORIENTED_EDGE('',*,*,#18083,.F.);
#25604=ORIENTED_EDGE('',*,*,#18084,.F.);
#25605=ORIENTED_EDGE('',*,*,#18085,.F.);
#25606=ORIENTED_EDGE('',*,*,#18084,.T.);
#25607=ORIENTED_EDGE('',*,*,#18086,.T.);
#25608=ORIENTED_EDGE('',*,*,#18087,.F.);
#25609=ORIENTED_EDGE('',*,*,#18086,.F.);
#25610=ORIENTED_EDGE('',*,*,#18083,.T.);
#25611=ORIENTED_EDGE('',*,*,#18088,.T.);
#25612=ORIENTED_EDGE('',*,*,#18089,.F.);
#25613=ORIENTED_EDGE('',*,*,#18088,.F.);
#25614=ORIENTED_EDGE('',*,*,#18082,.F.);
#25615=ORIENTED_EDGE('',*,*,#18090,.F.);
#25616=ORIENTED_EDGE('',*,*,#18091,.T.);
#25617=ORIENTED_EDGE('',*,*,#18092,.F.);
#25618=ORIENTED_EDGE('',*,*,#18093,.F.);
#25619=ORIENTED_EDGE('',*,*,#18094,.F.);
#25620=ORIENTED_EDGE('',*,*,#18093,.T.);
#25621=ORIENTED_EDGE('',*,*,#18095,.T.);
#25622=ORIENTED_EDGE('',*,*,#18096,.F.);
#25623=ORIENTED_EDGE('',*,*,#18095,.F.);
#25624=ORIENTED_EDGE('',*,*,#18092,.T.);
#25625=ORIENTED_EDGE('',*,*,#18097,.T.);
#25626=ORIENTED_EDGE('',*,*,#18098,.F.);
#25627=ORIENTED_EDGE('',*,*,#18097,.F.);
#25628=ORIENTED_EDGE('',*,*,#18091,.F.);
#25629=ORIENTED_EDGE('',*,*,#18099,.F.);
#25630=ORIENTED_EDGE('',*,*,#18100,.T.);
#25631=ORIENTED_EDGE('',*,*,#18101,.F.);
#25632=ORIENTED_EDGE('',*,*,#18102,.F.);
#25633=ORIENTED_EDGE('',*,*,#18103,.F.);
#25634=ORIENTED_EDGE('',*,*,#18102,.T.);
#25635=ORIENTED_EDGE('',*,*,#18104,.T.);
#25636=ORIENTED_EDGE('',*,*,#18105,.F.);
#25637=ORIENTED_EDGE('',*,*,#18104,.F.);
#25638=ORIENTED_EDGE('',*,*,#18101,.T.);
#25639=ORIENTED_EDGE('',*,*,#18106,.T.);
#25640=ORIENTED_EDGE('',*,*,#18107,.F.);
#25641=ORIENTED_EDGE('',*,*,#18106,.F.);
#25642=ORIENTED_EDGE('',*,*,#18100,.F.);
#25643=ORIENTED_EDGE('',*,*,#18108,.F.);
#25644=ORIENTED_EDGE('',*,*,#18109,.T.);
#25645=ORIENTED_EDGE('',*,*,#18110,.F.);
#25646=ORIENTED_EDGE('',*,*,#18111,.F.);
#25647=ORIENTED_EDGE('',*,*,#18112,.F.);
#25648=ORIENTED_EDGE('',*,*,#18111,.T.);
#25649=ORIENTED_EDGE('',*,*,#18113,.T.);
#25650=ORIENTED_EDGE('',*,*,#18114,.F.);
#25651=ORIENTED_EDGE('',*,*,#18113,.F.);
#25652=ORIENTED_EDGE('',*,*,#18110,.T.);
#25653=ORIENTED_EDGE('',*,*,#18115,.T.);
#25654=ORIENTED_EDGE('',*,*,#18116,.F.);
#25655=ORIENTED_EDGE('',*,*,#18115,.F.);
#25656=ORIENTED_EDGE('',*,*,#18109,.F.);
#25657=ORIENTED_EDGE('',*,*,#18117,.F.);
#25658=ORIENTED_EDGE('',*,*,#18118,.T.);
#25659=ORIENTED_EDGE('',*,*,#18119,.F.);
#25660=ORIENTED_EDGE('',*,*,#18120,.F.);
#25661=ORIENTED_EDGE('',*,*,#18121,.F.);
#25662=ORIENTED_EDGE('',*,*,#18120,.T.);
#25663=ORIENTED_EDGE('',*,*,#18122,.T.);
#25664=ORIENTED_EDGE('',*,*,#18123,.F.);
#25665=ORIENTED_EDGE('',*,*,#18122,.F.);
#25666=ORIENTED_EDGE('',*,*,#18119,.T.);
#25667=ORIENTED_EDGE('',*,*,#18124,.T.);
#25668=ORIENTED_EDGE('',*,*,#18125,.F.);
#25669=ORIENTED_EDGE('',*,*,#18124,.F.);
#25670=ORIENTED_EDGE('',*,*,#18118,.F.);
#25671=ORIENTED_EDGE('',*,*,#18126,.F.);
#25672=ORIENTED_EDGE('',*,*,#18127,.T.);
#25673=ORIENTED_EDGE('',*,*,#18128,.F.);
#25674=ORIENTED_EDGE('',*,*,#18129,.F.);
#25675=ORIENTED_EDGE('',*,*,#18130,.F.);
#25676=ORIENTED_EDGE('',*,*,#18129,.T.);
#25677=ORIENTED_EDGE('',*,*,#18131,.T.);
#25678=ORIENTED_EDGE('',*,*,#18132,.F.);
#25679=ORIENTED_EDGE('',*,*,#18131,.F.);
#25680=ORIENTED_EDGE('',*,*,#18128,.T.);
#25681=ORIENTED_EDGE('',*,*,#18133,.T.);
#25682=ORIENTED_EDGE('',*,*,#18134,.F.);
#25683=ORIENTED_EDGE('',*,*,#18133,.F.);
#25684=ORIENTED_EDGE('',*,*,#18127,.F.);
#25685=ORIENTED_EDGE('',*,*,#18135,.F.);
#25686=ORIENTED_EDGE('',*,*,#18136,.T.);
#25687=ORIENTED_EDGE('',*,*,#18137,.F.);
#25688=ORIENTED_EDGE('',*,*,#18138,.F.);
#25689=ORIENTED_EDGE('',*,*,#18139,.F.);
#25690=ORIENTED_EDGE('',*,*,#18138,.T.);
#25691=ORIENTED_EDGE('',*,*,#18140,.T.);
#25692=ORIENTED_EDGE('',*,*,#18141,.F.);
#25693=ORIENTED_EDGE('',*,*,#18140,.F.);
#25694=ORIENTED_EDGE('',*,*,#18137,.T.);
#25695=ORIENTED_EDGE('',*,*,#18142,.T.);
#25696=ORIENTED_EDGE('',*,*,#18143,.F.);
#25697=ORIENTED_EDGE('',*,*,#18142,.F.);
#25698=ORIENTED_EDGE('',*,*,#18136,.F.);
#25699=ORIENTED_EDGE('',*,*,#18144,.F.);
#25700=ORIENTED_EDGE('',*,*,#18145,.T.);
#25701=ORIENTED_EDGE('',*,*,#18146,.F.);
#25702=ORIENTED_EDGE('',*,*,#18147,.F.);
#25703=ORIENTED_EDGE('',*,*,#18148,.F.);
#25704=ORIENTED_EDGE('',*,*,#18147,.T.);
#25705=ORIENTED_EDGE('',*,*,#18149,.T.);
#25706=ORIENTED_EDGE('',*,*,#18150,.F.);
#25707=ORIENTED_EDGE('',*,*,#18149,.F.);
#25708=ORIENTED_EDGE('',*,*,#18146,.T.);
#25709=ORIENTED_EDGE('',*,*,#18151,.T.);
#25710=ORIENTED_EDGE('',*,*,#18152,.F.);
#25711=ORIENTED_EDGE('',*,*,#18151,.F.);
#25712=ORIENTED_EDGE('',*,*,#18145,.F.);
#25713=ORIENTED_EDGE('',*,*,#18153,.T.);
#25714=ORIENTED_EDGE('',*,*,#18154,.F.);
#25715=ORIENTED_EDGE('',*,*,#18153,.F.);
#25716=ORIENTED_EDGE('',*,*,#18155,.F.);
#25717=ORIENTED_EDGE('',*,*,#18156,.T.);
#25718=ORIENTED_EDGE('',*,*,#18157,.T.);
#25719=ORIENTED_EDGE('',*,*,#18158,.F.);
#25720=ORIENTED_EDGE('',*,*,#18159,.F.);
#25721=ORIENTED_EDGE('',*,*,#18160,.T.);
#25722=ORIENTED_EDGE('',*,*,#18161,.T.);
#25723=ORIENTED_EDGE('',*,*,#18156,.F.);
#25724=ORIENTED_EDGE('',*,*,#18162,.F.);
#25725=ORIENTED_EDGE('',*,*,#18163,.T.);
#25726=ORIENTED_EDGE('',*,*,#18164,.T.);
#25727=ORIENTED_EDGE('',*,*,#18160,.F.);
#25728=ORIENTED_EDGE('',*,*,#18165,.F.);
#25729=ORIENTED_EDGE('',*,*,#18166,.T.);
#25730=ORIENTED_EDGE('',*,*,#18167,.T.);
#25731=ORIENTED_EDGE('',*,*,#18163,.F.);
#25732=ORIENTED_EDGE('',*,*,#18168,.F.);
#25733=ORIENTED_EDGE('',*,*,#18169,.T.);
#25734=ORIENTED_EDGE('',*,*,#18170,.T.);
#25735=ORIENTED_EDGE('',*,*,#18166,.F.);
#25736=ORIENTED_EDGE('',*,*,#18171,.F.);
#25737=ORIENTED_EDGE('',*,*,#18158,.T.);
#25738=ORIENTED_EDGE('',*,*,#18172,.T.);
#25739=ORIENTED_EDGE('',*,*,#18169,.F.);
#25740=ORIENTED_EDGE('',*,*,#18172,.F.);
#25741=ORIENTED_EDGE('',*,*,#18157,.F.);
#25742=ORIENTED_EDGE('',*,*,#18161,.F.);
#25743=ORIENTED_EDGE('',*,*,#18164,.F.);
#25744=ORIENTED_EDGE('',*,*,#18167,.F.);
#25745=ORIENTED_EDGE('',*,*,#18170,.F.);
#25746=ORIENTED_EDGE('',*,*,#18154,.T.);
#25747=ORIENTED_EDGE('',*,*,#18173,.F.);
#25748=ORIENTED_EDGE('',*,*,#17817,.F.);
#25749=ORIENTED_EDGE('',*,*,#17396,.F.);
#25750=ORIENTED_EDGE('',*,*,#17818,.F.);
#25751=ORIENTED_EDGE('',*,*,#18174,.T.);
#25752=ORIENTED_EDGE('',*,*,#18173,.T.);
#25753=ORIENTED_EDGE('',*,*,#18174,.F.);
#25754=ORIENTED_EDGE('',*,*,#18175,.F.);
#25755=ORIENTED_EDGE('',*,*,#18176,.T.);
#25756=ORIENTED_EDGE('',*,*,#17990,.T.);
#25757=ORIENTED_EDGE('',*,*,#17980,.T.);
#25758=ORIENTED_EDGE('',*,*,#17984,.T.);
#25759=ORIENTED_EDGE('',*,*,#18177,.T.);
#25760=ORIENTED_EDGE('',*,*,#17826,.T.);
#25761=ORIENTED_EDGE('',*,*,#18177,.F.);
#25762=ORIENTED_EDGE('',*,*,#17986,.T.);
#25763=ORIENTED_EDGE('',*,*,#17987,.T.);
#25764=ORIENTED_EDGE('',*,*,#17989,.T.);
#25765=ORIENTED_EDGE('',*,*,#18176,.F.);
#25766=ORIENTED_EDGE('',*,*,#17833,.T.);
#25767=ORIENTED_EDGE('',*,*,#17835,.T.);
#25768=ORIENTED_EDGE('',*,*,#17827,.T.);
#25769=ORIENTED_EDGE('',*,*,#17831,.T.);
#25770=ORIENTED_EDGE('',*,*,#17842,.T.);
#25771=ORIENTED_EDGE('',*,*,#17844,.T.);
#25772=ORIENTED_EDGE('',*,*,#17836,.T.);
#25773=ORIENTED_EDGE('',*,*,#17840,.T.);
#25774=ORIENTED_EDGE('',*,*,#17851,.T.);
#25775=ORIENTED_EDGE('',*,*,#17853,.T.);
#25776=ORIENTED_EDGE('',*,*,#17845,.T.);
#25777=ORIENTED_EDGE('',*,*,#17849,.T.);
#25778=ORIENTED_EDGE('',*,*,#17860,.T.);
#25779=ORIENTED_EDGE('',*,*,#17862,.T.);
#25780=ORIENTED_EDGE('',*,*,#17854,.T.);
#25781=ORIENTED_EDGE('',*,*,#17858,.T.);
#25782=ORIENTED_EDGE('',*,*,#17869,.T.);
#25783=ORIENTED_EDGE('',*,*,#17871,.T.);
#25784=ORIENTED_EDGE('',*,*,#17863,.T.);
#25785=ORIENTED_EDGE('',*,*,#17867,.T.);
#25786=ORIENTED_EDGE('',*,*,#17878,.T.);
#25787=ORIENTED_EDGE('',*,*,#17880,.T.);
#25788=ORIENTED_EDGE('',*,*,#17872,.T.);
#25789=ORIENTED_EDGE('',*,*,#17876,.T.);
#25790=ORIENTED_EDGE('',*,*,#17887,.T.);
#25791=ORIENTED_EDGE('',*,*,#17889,.T.);
#25792=ORIENTED_EDGE('',*,*,#17881,.T.);
#25793=ORIENTED_EDGE('',*,*,#17885,.T.);
#25794=ORIENTED_EDGE('',*,*,#17896,.T.);
#25795=ORIENTED_EDGE('',*,*,#17898,.T.);
#25796=ORIENTED_EDGE('',*,*,#17890,.T.);
#25797=ORIENTED_EDGE('',*,*,#17894,.T.);
#25798=ORIENTED_EDGE('',*,*,#17905,.T.);
#25799=ORIENTED_EDGE('',*,*,#17907,.T.);
#25800=ORIENTED_EDGE('',*,*,#17899,.T.);
#25801=ORIENTED_EDGE('',*,*,#17903,.T.);
#25802=ORIENTED_EDGE('',*,*,#17914,.T.);
#25803=ORIENTED_EDGE('',*,*,#17916,.T.);
#25804=ORIENTED_EDGE('',*,*,#17908,.T.);
#25805=ORIENTED_EDGE('',*,*,#17912,.T.);
#25806=ORIENTED_EDGE('',*,*,#17923,.T.);
#25807=ORIENTED_EDGE('',*,*,#17925,.T.);
#25808=ORIENTED_EDGE('',*,*,#17917,.T.);
#25809=ORIENTED_EDGE('',*,*,#17921,.T.);
#25810=ORIENTED_EDGE('',*,*,#17932,.T.);
#25811=ORIENTED_EDGE('',*,*,#17934,.T.);
#25812=ORIENTED_EDGE('',*,*,#17926,.T.);
#25813=ORIENTED_EDGE('',*,*,#17930,.T.);
#25814=ORIENTED_EDGE('',*,*,#17941,.T.);
#25815=ORIENTED_EDGE('',*,*,#17943,.T.);
#25816=ORIENTED_EDGE('',*,*,#17935,.T.);
#25817=ORIENTED_EDGE('',*,*,#17939,.T.);
#25818=ORIENTED_EDGE('',*,*,#17950,.T.);
#25819=ORIENTED_EDGE('',*,*,#17952,.T.);
#25820=ORIENTED_EDGE('',*,*,#17944,.T.);
#25821=ORIENTED_EDGE('',*,*,#17948,.T.);
#25822=ORIENTED_EDGE('',*,*,#17959,.T.);
#25823=ORIENTED_EDGE('',*,*,#17961,.T.);
#25824=ORIENTED_EDGE('',*,*,#17953,.T.);
#25825=ORIENTED_EDGE('',*,*,#17957,.T.);
#25826=ORIENTED_EDGE('',*,*,#17968,.T.);
#25827=ORIENTED_EDGE('',*,*,#17970,.T.);
#25828=ORIENTED_EDGE('',*,*,#17962,.T.);
#25829=ORIENTED_EDGE('',*,*,#17966,.T.);
#25830=ORIENTED_EDGE('',*,*,#17977,.T.);
#25831=ORIENTED_EDGE('',*,*,#17979,.T.);
#25832=ORIENTED_EDGE('',*,*,#17971,.T.);
#25833=ORIENTED_EDGE('',*,*,#17975,.T.);
#25834=ORIENTED_EDGE('',*,*,#17997,.T.);
#25835=ORIENTED_EDGE('',*,*,#17999,.T.);
#25836=ORIENTED_EDGE('',*,*,#17991,.T.);
#25837=ORIENTED_EDGE('',*,*,#17995,.T.);
#25838=ORIENTED_EDGE('',*,*,#18006,.T.);
#25839=ORIENTED_EDGE('',*,*,#18008,.T.);
#25840=ORIENTED_EDGE('',*,*,#18000,.T.);
#25841=ORIENTED_EDGE('',*,*,#18004,.T.);
#25842=ORIENTED_EDGE('',*,*,#18015,.T.);
#25843=ORIENTED_EDGE('',*,*,#18017,.T.);
#25844=ORIENTED_EDGE('',*,*,#18009,.T.);
#25845=ORIENTED_EDGE('',*,*,#18013,.T.);
#25846=ORIENTED_EDGE('',*,*,#18024,.T.);
#25847=ORIENTED_EDGE('',*,*,#18026,.T.);
#25848=ORIENTED_EDGE('',*,*,#18018,.T.);
#25849=ORIENTED_EDGE('',*,*,#18022,.T.);
#25850=ORIENTED_EDGE('',*,*,#18033,.T.);
#25851=ORIENTED_EDGE('',*,*,#18035,.T.);
#25852=ORIENTED_EDGE('',*,*,#18027,.T.);
#25853=ORIENTED_EDGE('',*,*,#18031,.T.);
#25854=ORIENTED_EDGE('',*,*,#18042,.T.);
#25855=ORIENTED_EDGE('',*,*,#18044,.T.);
#25856=ORIENTED_EDGE('',*,*,#18036,.T.);
#25857=ORIENTED_EDGE('',*,*,#18040,.T.);
#25858=ORIENTED_EDGE('',*,*,#18051,.T.);
#25859=ORIENTED_EDGE('',*,*,#18053,.T.);
#25860=ORIENTED_EDGE('',*,*,#18045,.T.);
#25861=ORIENTED_EDGE('',*,*,#18049,.T.);
#25862=ORIENTED_EDGE('',*,*,#18060,.T.);
#25863=ORIENTED_EDGE('',*,*,#18062,.T.);
#25864=ORIENTED_EDGE('',*,*,#18054,.T.);
#25865=ORIENTED_EDGE('',*,*,#18058,.T.);
#25866=ORIENTED_EDGE('',*,*,#18069,.T.);
#25867=ORIENTED_EDGE('',*,*,#18071,.T.);
#25868=ORIENTED_EDGE('',*,*,#18063,.T.);
#25869=ORIENTED_EDGE('',*,*,#18067,.T.);
#25870=ORIENTED_EDGE('',*,*,#18078,.T.);
#25871=ORIENTED_EDGE('',*,*,#18080,.T.);
#25872=ORIENTED_EDGE('',*,*,#18072,.T.);
#25873=ORIENTED_EDGE('',*,*,#18076,.T.);
#25874=ORIENTED_EDGE('',*,*,#18087,.T.);
#25875=ORIENTED_EDGE('',*,*,#18089,.T.);
#25876=ORIENTED_EDGE('',*,*,#18081,.T.);
#25877=ORIENTED_EDGE('',*,*,#18085,.T.);
#25878=ORIENTED_EDGE('',*,*,#18096,.T.);
#25879=ORIENTED_EDGE('',*,*,#18098,.T.);
#25880=ORIENTED_EDGE('',*,*,#18090,.T.);
#25881=ORIENTED_EDGE('',*,*,#18094,.T.);
#25882=ORIENTED_EDGE('',*,*,#18105,.T.);
#25883=ORIENTED_EDGE('',*,*,#18107,.T.);
#25884=ORIENTED_EDGE('',*,*,#18099,.T.);
#25885=ORIENTED_EDGE('',*,*,#18103,.T.);
#25886=ORIENTED_EDGE('',*,*,#18114,.T.);
#25887=ORIENTED_EDGE('',*,*,#18116,.T.);
#25888=ORIENTED_EDGE('',*,*,#18108,.T.);
#25889=ORIENTED_EDGE('',*,*,#18112,.T.);
#25890=ORIENTED_EDGE('',*,*,#18123,.T.);
#25891=ORIENTED_EDGE('',*,*,#18125,.T.);
#25892=ORIENTED_EDGE('',*,*,#18117,.T.);
#25893=ORIENTED_EDGE('',*,*,#18121,.T.);
#25894=ORIENTED_EDGE('',*,*,#18132,.T.);
#25895=ORIENTED_EDGE('',*,*,#18134,.T.);
#25896=ORIENTED_EDGE('',*,*,#18126,.T.);
#25897=ORIENTED_EDGE('',*,*,#18130,.T.);
#25898=ORIENTED_EDGE('',*,*,#18141,.T.);
#25899=ORIENTED_EDGE('',*,*,#18143,.T.);
#25900=ORIENTED_EDGE('',*,*,#18135,.T.);
#25901=ORIENTED_EDGE('',*,*,#18139,.T.);
#25902=ORIENTED_EDGE('',*,*,#18150,.T.);
#25903=ORIENTED_EDGE('',*,*,#18152,.T.);
#25904=ORIENTED_EDGE('',*,*,#18144,.T.);
#25905=ORIENTED_EDGE('',*,*,#18148,.T.);
#25906=ORIENTED_EDGE('',*,*,#18178,.F.);
#25907=ORIENTED_EDGE('',*,*,#18179,.T.);
#25908=ORIENTED_EDGE('',*,*,#18175,.T.);
#25909=ORIENTED_EDGE('',*,*,#18179,.F.);
#25910=ORIENTED_EDGE('',*,*,#18178,.T.);
#25911=ORIENTED_EDGE('',*,*,#18155,.T.);
#25912=ORIENTED_EDGE('',*,*,#18171,.T.);
#25913=ORIENTED_EDGE('',*,*,#18168,.T.);
#25914=ORIENTED_EDGE('',*,*,#18165,.T.);
#25915=ORIENTED_EDGE('',*,*,#18162,.T.);
#25916=ORIENTED_EDGE('',*,*,#18159,.T.);
#28636=PLANE('',#32595);
#28637=PLANE('',#32598);
#28638=PLANE('',#32608);
#28639=PLANE('',#32610);
#28640=PLANE('',#32611);
#28641=PLANE('',#32613);
#28642=PLANE('',#32614);
#28643=PLANE('',#32616);
#28644=PLANE('',#32617);
#28645=PLANE('',#32619);
#28646=PLANE('',#32620);
#28647=PLANE('',#32622);
#28648=PLANE('',#32623);
#28649=PLANE('',#32625);
#28650=PLANE('',#32626);
#28651=PLANE('',#32628);
#28652=PLANE('',#32629);
#28653=PLANE('',#32631);
#28654=PLANE('',#32632);
#28655=PLANE('',#32634);
#28656=PLANE('',#32635);
#28657=PLANE('',#32637);
#28658=PLANE('',#32638);
#28659=PLANE('',#32640);
#28660=PLANE('',#32641);
#28661=PLANE('',#32643);
#28662=PLANE('',#32644);
#28663=PLANE('',#32646);
#28664=PLANE('',#32647);
#28665=PLANE('',#32649);
#28666=PLANE('',#32650);
#28667=PLANE('',#32652);
#28668=PLANE('',#32653);
#28669=PLANE('',#32655);
#28670=PLANE('',#32656);
#28671=PLANE('',#32658);
#28672=PLANE('',#32659);
#28673=PLANE('',#32661);
#28674=PLANE('',#32662);
#28675=PLANE('',#32664);
#28676=PLANE('',#32665);
#28677=PLANE('',#32667);
#28678=PLANE('',#32668);
#28679=PLANE('',#32670);
#28680=PLANE('',#32671);
#28681=PLANE('',#32673);
#28682=PLANE('',#32674);
#28683=PLANE('',#32676);
#28684=PLANE('',#32677);
#28685=PLANE('',#32679);
#28686=PLANE('',#32680);
#28687=PLANE('',#32682);
#28688=PLANE('',#32683);
#28689=PLANE('',#32685);
#28690=PLANE('',#32686);
#28691=PLANE('',#32688);
#28692=PLANE('',#32689);
#28693=PLANE('',#32691);
#28694=PLANE('',#32692);
#28695=PLANE('',#32694);
#28696=PLANE('',#32695);
#28697=PLANE('',#32697);
#28698=PLANE('',#32698);
#28699=PLANE('',#32700);
#28700=PLANE('',#32701);
#28701=PLANE('',#32703);
#28702=PLANE('',#32704);
#28703=PLANE('',#32706);
#28704=PLANE('',#32707);
#28705=PLANE('',#32709);
#28706=PLANE('',#32710);
#28707=PLANE('',#32712);
#28708=PLANE('',#32713);
#28709=PLANE('',#32716);
#28710=PLANE('',#32717);
#28711=PLANE('',#32720);
#28712=PLANE('',#32721);
#28713=PLANE('',#32723);
#28714=PLANE('',#32724);
#28715=PLANE('',#32726);
#28716=PLANE('',#32727);
#28717=PLANE('',#32729);
#28718=PLANE('',#32730);
#28719=PLANE('',#32732);
#28720=PLANE('',#32733);
#28721=PLANE('',#32735);
#28722=PLANE('',#32736);
#28723=PLANE('',#32738);
#28724=PLANE('',#32739);
#28725=PLANE('',#32741);
#28726=PLANE('',#32742);
#28727=PLANE('',#32744);
#28728=PLANE('',#32745);
#28729=PLANE('',#32747);
#28730=PLANE('',#32748);
#28731=PLANE('',#32750);
#28732=PLANE('',#32751);
#28733=PLANE('',#32753);
#28734=PLANE('',#32754);
#28735=PLANE('',#32756);
#28736=PLANE('',#32757);
#28737=PLANE('',#32759);
#28738=PLANE('',#32760);
#28739=PLANE('',#32762);
#28740=PLANE('',#32763);
#28741=PLANE('',#32765);
#28742=PLANE('',#32766);
#28743=PLANE('',#32768);
#28744=PLANE('',#32769);
#28745=PLANE('',#32771);
#28746=PLANE('',#32772);
#28747=PLANE('',#32774);
#28748=PLANE('',#32775);
#28749=PLANE('',#32777);
#28750=PLANE('',#32778);
#28751=PLANE('',#32780);
#28752=PLANE('',#32781);
#28753=PLANE('',#32783);
#28754=PLANE('',#32784);
#28755=PLANE('',#32786);
#28756=PLANE('',#32787);
#28757=PLANE('',#32789);
#28758=PLANE('',#32790);
#28759=PLANE('',#32792);
#28760=PLANE('',#32793);
#28761=PLANE('',#32795);
#28762=PLANE('',#32796);
#28763=PLANE('',#32798);
#28764=PLANE('',#32799);
#28765=PLANE('',#32801);
#28766=PLANE('',#32802);
#28767=PLANE('',#32804);
#28768=PLANE('',#32805);
#28769=PLANE('',#32807);
#28770=PLANE('',#32808);
#28771=PLANE('',#32810);
#28772=PLANE('',#32811);
#28773=PLANE('',#32813);
#28774=PLANE('',#32814);
#28775=PLANE('',#32816);
#28776=PLANE('',#32817);
#28777=PLANE('',#32819);
#28778=PLANE('',#32820);
#28779=PLANE('',#32822);
#28780=PLANE('',#32823);
#28781=PLANE('',#32825);
#28782=PLANE('',#32826);
#28783=PLANE('',#32830);
#28784=PLANE('',#32831);
#28785=PLANE('',#32832);
#28786=PLANE('',#32833);
#28787=PLANE('',#32834);
#28788=PLANE('',#32835);
#28789=PLANE('',#32836);
#28790=PLANE('',#32837);
#28791=PLANE('',#32844);
#29972=ADVANCED_FACE('',(#4644),#666,.T.);
#29973=ADVANCED_FACE('',(#4645),#667,.T.);
#29974=ADVANCED_FACE('',(#4646),#668,.T.);
#29975=ADVANCED_FACE('',(#4647),#669,.T.);
#29976=ADVANCED_FACE('',(#4648),#670,.T.);
#29977=ADVANCED_FACE('',(#4649),#671,.T.);
#29978=ADVANCED_FACE('',(#4650),#672,.T.);
#29979=ADVANCED_FACE('',(#4651),#673,.T.);
#29980=ADVANCED_FACE('',(#4652),#674,.T.);
#29981=ADVANCED_FACE('',(#4653),#675,.T.);
#29982=ADVANCED_FACE('',(#4654),#676,.T.);
#29983=ADVANCED_FACE('',(#4655),#677,.T.);
#29984=ADVANCED_FACE('',(#4656),#678,.T.);
#29985=ADVANCED_FACE('',(#4657),#679,.T.);
#29986=ADVANCED_FACE('',(#4658),#680,.T.);
#29987=ADVANCED_FACE('',(#4659),#681,.T.);
#29988=ADVANCED_FACE('',(#4660),#682,.T.);
#29989=ADVANCED_FACE('',(#4661),#683,.T.);
#29990=ADVANCED_FACE('',(#4662),#684,.T.);
#29991=ADVANCED_FACE('',(#4663),#685,.T.);
#29992=ADVANCED_FACE('',(#4664),#686,.T.);
#29993=ADVANCED_FACE('',(#4665),#687,.T.);
#29994=ADVANCED_FACE('',(#4666),#688,.T.);
#29995=ADVANCED_FACE('',(#4667),#689,.T.);
#29996=ADVANCED_FACE('',(#4668),#690,.T.);
#29997=ADVANCED_FACE('',(#4669),#691,.T.);
#29998=ADVANCED_FACE('',(#4670),#692,.T.);
#29999=ADVANCED_FACE('',(#4671),#693,.T.);
#30000=ADVANCED_FACE('',(#4672),#694,.T.);
#30001=ADVANCED_FACE('',(#4673),#695,.T.);
#30002=ADVANCED_FACE('',(#4674),#696,.T.);
#30003=ADVANCED_FACE('',(#4675),#697,.T.);
#30004=ADVANCED_FACE('',(#4676),#698,.T.);
#30005=ADVANCED_FACE('',(#4677),#699,.T.);
#30006=ADVANCED_FACE('',(#4678),#700,.T.);
#30007=ADVANCED_FACE('',(#4679),#701,.T.);
#30008=ADVANCED_FACE('',(#4680),#702,.T.);
#30009=ADVANCED_FACE('',(#4681),#703,.T.);
#30010=ADVANCED_FACE('',(#4682),#704,.T.);
#30011=ADVANCED_FACE('',(#4683),#705,.T.);
#30012=ADVANCED_FACE('',(#4684),#706,.T.);
#30013=ADVANCED_FACE('',(#4685),#707,.T.);
#30014=ADVANCED_FACE('',(#4686),#708,.T.);
#30015=ADVANCED_FACE('',(#4687),#709,.T.);
#30016=ADVANCED_FACE('',(#4688),#710,.T.);
#30017=ADVANCED_FACE('',(#4689),#711,.T.);
#30018=ADVANCED_FACE('',(#4690),#712,.T.);
#30019=ADVANCED_FACE('',(#4691),#713,.T.);
#30020=ADVANCED_FACE('',(#4692),#714,.T.);
#30021=ADVANCED_FACE('',(#4693),#715,.T.);
#30022=ADVANCED_FACE('',(#4694),#716,.T.);
#30023=ADVANCED_FACE('',(#4695),#717,.T.);
#30024=ADVANCED_FACE('',(#4696),#718,.T.);
#30025=ADVANCED_FACE('',(#4697),#719,.T.);
#30026=ADVANCED_FACE('',(#4698),#720,.T.);
#30027=ADVANCED_FACE('',(#4699),#721,.T.);
#30028=ADVANCED_FACE('',(#4700),#722,.T.);
#30029=ADVANCED_FACE('',(#4701),#723,.T.);
#30030=ADVANCED_FACE('',(#4702),#724,.T.);
#30031=ADVANCED_FACE('',(#4703),#725,.T.);
#30032=ADVANCED_FACE('',(#4704),#726,.T.);
#30033=ADVANCED_FACE('',(#4705),#727,.T.);
#30034=ADVANCED_FACE('',(#4706),#728,.T.);
#30035=ADVANCED_FACE('',(#4707),#729,.T.);
#30036=ADVANCED_FACE('',(#4708),#730,.T.);
#30037=ADVANCED_FACE('',(#4709),#731,.T.);
#30038=ADVANCED_FACE('',(#4710),#732,.T.);
#30039=ADVANCED_FACE('',(#4711),#733,.T.);
#30040=ADVANCED_FACE('',(#4712),#734,.T.);
#30041=ADVANCED_FACE('',(#4713),#735,.T.);
#30042=ADVANCED_FACE('',(#4714),#736,.T.);
#30043=ADVANCED_FACE('',(#4715),#737,.T.);
#30044=ADVANCED_FACE('',(#4716),#738,.T.);
#30045=ADVANCED_FACE('',(#4717),#739,.T.);
#30046=ADVANCED_FACE('',(#4718),#740,.T.);
#30047=ADVANCED_FACE('',(#4719),#741,.T.);
#30048=ADVANCED_FACE('',(#4720),#742,.T.);
#30049=ADVANCED_FACE('',(#4721),#743,.T.);
#30050=ADVANCED_FACE('',(#4722),#744,.T.);
#30051=ADVANCED_FACE('',(#4723),#745,.T.);
#30052=ADVANCED_FACE('',(#4724),#746,.T.);
#30053=ADVANCED_FACE('',(#4725),#747,.T.);
#30054=ADVANCED_FACE('',(#4726),#748,.T.);
#30055=ADVANCED_FACE('',(#4727),#749,.T.);
#30056=ADVANCED_FACE('',(#4728),#750,.T.);
#30057=ADVANCED_FACE('',(#4729),#751,.T.);
#30058=ADVANCED_FACE('',(#4730),#752,.T.);
#30059=ADVANCED_FACE('',(#4731),#753,.T.);
#30060=ADVANCED_FACE('',(#4732),#754,.T.);
#30061=ADVANCED_FACE('',(#4733),#755,.T.);
#30062=ADVANCED_FACE('',(#4734),#756,.T.);
#30063=ADVANCED_FACE('',(#4735),#757,.T.);
#30064=ADVANCED_FACE('',(#4736),#758,.T.);
#30065=ADVANCED_FACE('',(#4737),#759,.T.);
#30066=ADVANCED_FACE('',(#4738),#760,.T.);
#30067=ADVANCED_FACE('',(#4739),#761,.T.);
#30068=ADVANCED_FACE('',(#4740),#762,.T.);
#30069=ADVANCED_FACE('',(#4741),#763,.T.);
#30070=ADVANCED_FACE('',(#4742),#764,.T.);
#30071=ADVANCED_FACE('',(#4743),#765,.T.);
#30072=ADVANCED_FACE('',(#4744),#766,.T.);
#30073=ADVANCED_FACE('',(#4745),#767,.T.);
#30074=ADVANCED_FACE('',(#4746),#768,.T.);
#30075=ADVANCED_FACE('',(#4747),#769,.T.);
#30076=ADVANCED_FACE('',(#4748),#770,.T.);
#30077=ADVANCED_FACE('',(#4749),#771,.T.);
#30078=ADVANCED_FACE('',(#4750),#772,.T.);
#30079=ADVANCED_FACE('',(#4751),#773,.T.);
#30080=ADVANCED_FACE('',(#4752),#774,.T.);
#30081=ADVANCED_FACE('',(#4753),#775,.T.);
#30082=ADVANCED_FACE('',(#4754),#776,.T.);
#30083=ADVANCED_FACE('',(#4755),#777,.T.);
#30084=ADVANCED_FACE('',(#4756),#778,.T.);
#30085=ADVANCED_FACE('',(#4757),#779,.T.);
#30086=ADVANCED_FACE('',(#4758),#780,.T.);
#30087=ADVANCED_FACE('',(#4759),#781,.T.);
#30088=ADVANCED_FACE('',(#4760),#782,.T.);
#30089=ADVANCED_FACE('',(#4761),#783,.T.);
#30090=ADVANCED_FACE('',(#4762),#784,.T.);
#30091=ADVANCED_FACE('',(#4763),#785,.T.);
#30092=ADVANCED_FACE('',(#4764),#786,.T.);
#30093=ADVANCED_FACE('',(#4765),#787,.T.);
#30094=ADVANCED_FACE('',(#4766),#788,.T.);
#30095=ADVANCED_FACE('',(#4767),#789,.T.);
#30096=ADVANCED_FACE('',(#4768),#790,.T.);
#30097=ADVANCED_FACE('',(#4769),#791,.T.);
#30098=ADVANCED_FACE('',(#4770),#792,.T.);
#30099=ADVANCED_FACE('',(#4771),#793,.T.);
#30100=ADVANCED_FACE('',(#4772),#794,.T.);
#30101=ADVANCED_FACE('',(#4773),#795,.T.);
#30102=ADVANCED_FACE('',(#4774),#796,.T.);
#30103=ADVANCED_FACE('',(#4775),#797,.T.);
#30104=ADVANCED_FACE('',(#4776),#798,.T.);
#30105=ADVANCED_FACE('',(#4777),#799,.T.);
#30106=ADVANCED_FACE('',(#4778),#800,.T.);
#30107=ADVANCED_FACE('',(#4779),#801,.T.);
#30108=ADVANCED_FACE('',(#4780),#802,.T.);
#30109=ADVANCED_FACE('',(#4781),#803,.T.);
#30110=ADVANCED_FACE('',(#4782),#28636,.F.);
#30111=ADVANCED_FACE('',(#4783),#424,.F.);
#30112=ADVANCED_FACE('',(#4784),#28637,.T.);
#30113=ADVANCED_FACE('',(#4785),#804,.T.);
#30114=ADVANCED_FACE('',(#4786),#425,.F.);
#30115=ADVANCED_FACE('',(#4787),#161,.F.);
#30116=ADVANCED_FACE('',(#4788),#805,.T.);
#30117=ADVANCED_FACE('',(#4789,#3526),#28638,.T.);
#30118=ADVANCED_FACE('',(#4790),#28639,.F.);
#30119=ADVANCED_FACE('',(#4791),#28640,.T.);
#30120=ADVANCED_FACE('',(#4792),#28641,.F.);
#30121=ADVANCED_FACE('',(#4793),#28642,.F.);
#30122=ADVANCED_FACE('',(#4794),#28643,.F.);
#30123=ADVANCED_FACE('',(#4795),#28644,.T.);
#30124=ADVANCED_FACE('',(#4796),#28645,.F.);
#30125=ADVANCED_FACE('',(#4797),#28646,.F.);
#30126=ADVANCED_FACE('',(#4798),#28647,.F.);
#30127=ADVANCED_FACE('',(#4799),#28648,.T.);
#30128=ADVANCED_FACE('',(#4800),#28649,.F.);
#30129=ADVANCED_FACE('',(#4801),#28650,.F.);
#30130=ADVANCED_FACE('',(#4802),#28651,.F.);
#30131=ADVANCED_FACE('',(#4803),#28652,.T.);
#30132=ADVANCED_FACE('',(#4804),#28653,.F.);
#30133=ADVANCED_FACE('',(#4805),#28654,.F.);
#30134=ADVANCED_FACE('',(#4806),#28655,.F.);
#30135=ADVANCED_FACE('',(#4807),#28656,.T.);
#30136=ADVANCED_FACE('',(#4808),#28657,.F.);
#30137=ADVANCED_FACE('',(#4809),#28658,.F.);
#30138=ADVANCED_FACE('',(#4810),#28659,.F.);
#30139=ADVANCED_FACE('',(#4811),#28660,.T.);
#30140=ADVANCED_FACE('',(#4812),#28661,.F.);
#30141=ADVANCED_FACE('',(#4813),#28662,.F.);
#30142=ADVANCED_FACE('',(#4814),#28663,.F.);
#30143=ADVANCED_FACE('',(#4815),#28664,.T.);
#30144=ADVANCED_FACE('',(#4816),#28665,.F.);
#30145=ADVANCED_FACE('',(#4817),#28666,.F.);
#30146=ADVANCED_FACE('',(#4818),#28667,.F.);
#30147=ADVANCED_FACE('',(#4819),#28668,.T.);
#30148=ADVANCED_FACE('',(#4820),#28669,.F.);
#30149=ADVANCED_FACE('',(#4821),#28670,.F.);
#30150=ADVANCED_FACE('',(#4822),#28671,.F.);
#30151=ADVANCED_FACE('',(#4823),#28672,.T.);
#30152=ADVANCED_FACE('',(#4824),#28673,.F.);
#30153=ADVANCED_FACE('',(#4825),#28674,.F.);
#30154=ADVANCED_FACE('',(#4826),#28675,.F.);
#30155=ADVANCED_FACE('',(#4827),#28676,.T.);
#30156=ADVANCED_FACE('',(#4828),#28677,.F.);
#30157=ADVANCED_FACE('',(#4829),#28678,.F.);
#30158=ADVANCED_FACE('',(#4830),#28679,.F.);
#30159=ADVANCED_FACE('',(#4831),#28680,.T.);
#30160=ADVANCED_FACE('',(#4832),#28681,.F.);
#30161=ADVANCED_FACE('',(#4833),#28682,.F.);
#30162=ADVANCED_FACE('',(#4834),#28683,.F.);
#30163=ADVANCED_FACE('',(#4835),#28684,.T.);
#30164=ADVANCED_FACE('',(#4836),#28685,.F.);
#30165=ADVANCED_FACE('',(#4837),#28686,.F.);
#30166=ADVANCED_FACE('',(#4838),#28687,.F.);
#30167=ADVANCED_FACE('',(#4839),#28688,.T.);
#30168=ADVANCED_FACE('',(#4840),#28689,.F.);
#30169=ADVANCED_FACE('',(#4841),#28690,.F.);
#30170=ADVANCED_FACE('',(#4842),#28691,.F.);
#30171=ADVANCED_FACE('',(#4843),#28692,.T.);
#30172=ADVANCED_FACE('',(#4844),#28693,.F.);
#30173=ADVANCED_FACE('',(#4845),#28694,.F.);
#30174=ADVANCED_FACE('',(#4846),#28695,.F.);
#30175=ADVANCED_FACE('',(#4847),#28696,.T.);
#30176=ADVANCED_FACE('',(#4848),#28697,.F.);
#30177=ADVANCED_FACE('',(#4849),#28698,.F.);
#30178=ADVANCED_FACE('',(#4850),#28699,.F.);
#30179=ADVANCED_FACE('',(#4851),#28700,.T.);
#30180=ADVANCED_FACE('',(#4852),#28701,.F.);
#30181=ADVANCED_FACE('',(#4853),#28702,.F.);
#30182=ADVANCED_FACE('',(#4854),#28703,.F.);
#30183=ADVANCED_FACE('',(#4855),#28704,.T.);
#30184=ADVANCED_FACE('',(#4856),#28705,.F.);
#30185=ADVANCED_FACE('',(#4857),#28706,.F.);
#30186=ADVANCED_FACE('',(#4858),#28707,.F.);
#30187=ADVANCED_FACE('',(#4859),#28708,.T.);
#30188=ADVANCED_FACE('',(#4860),#28709,.F.);
#30189=ADVANCED_FACE('',(#4861),#28710,.F.);
#30190=ADVANCED_FACE('',(#4862),#28711,.F.);
#30191=ADVANCED_FACE('',(#4863),#28712,.T.);
#30192=ADVANCED_FACE('',(#4864),#28713,.F.);
#30193=ADVANCED_FACE('',(#4865),#28714,.F.);
#30194=ADVANCED_FACE('',(#4866),#28715,.F.);
#30195=ADVANCED_FACE('',(#4867),#28716,.T.);
#30196=ADVANCED_FACE('',(#4868),#28717,.F.);
#30197=ADVANCED_FACE('',(#4869),#28718,.F.);
#30198=ADVANCED_FACE('',(#4870),#28719,.F.);
#30199=ADVANCED_FACE('',(#4871),#28720,.T.);
#30200=ADVANCED_FACE('',(#4872),#28721,.F.);
#30201=ADVANCED_FACE('',(#4873),#28722,.F.);
#30202=ADVANCED_FACE('',(#4874),#28723,.F.);
#30203=ADVANCED_FACE('',(#4875),#28724,.T.);
#30204=ADVANCED_FACE('',(#4876),#28725,.F.);
#30205=ADVANCED_FACE('',(#4877),#28726,.F.);
#30206=ADVANCED_FACE('',(#4878),#28727,.F.);
#30207=ADVANCED_FACE('',(#4879),#28728,.T.);
#30208=ADVANCED_FACE('',(#4880),#28729,.F.);
#30209=ADVANCED_FACE('',(#4881),#28730,.F.);
#30210=ADVANCED_FACE('',(#4882),#28731,.F.);
#30211=ADVANCED_FACE('',(#4883),#28732,.T.);
#30212=ADVANCED_FACE('',(#4884),#28733,.F.);
#30213=ADVANCED_FACE('',(#4885),#28734,.F.);
#30214=ADVANCED_FACE('',(#4886),#28735,.F.);
#30215=ADVANCED_FACE('',(#4887),#28736,.T.);
#30216=ADVANCED_FACE('',(#4888),#28737,.F.);
#30217=ADVANCED_FACE('',(#4889),#28738,.F.);
#30218=ADVANCED_FACE('',(#4890),#28739,.F.);
#30219=ADVANCED_FACE('',(#4891),#28740,.T.);
#30220=ADVANCED_FACE('',(#4892),#28741,.F.);
#30221=ADVANCED_FACE('',(#4893),#28742,.F.);
#30222=ADVANCED_FACE('',(#4894),#28743,.F.);
#30223=ADVANCED_FACE('',(#4895),#28744,.T.);
#30224=ADVANCED_FACE('',(#4896),#28745,.F.);
#30225=ADVANCED_FACE('',(#4897),#28746,.F.);
#30226=ADVANCED_FACE('',(#4898),#28747,.F.);
#30227=ADVANCED_FACE('',(#4899),#28748,.T.);
#30228=ADVANCED_FACE('',(#4900),#28749,.F.);
#30229=ADVANCED_FACE('',(#4901),#28750,.F.);
#30230=ADVANCED_FACE('',(#4902),#28751,.F.);
#30231=ADVANCED_FACE('',(#4903),#28752,.T.);
#30232=ADVANCED_FACE('',(#4904),#28753,.F.);
#30233=ADVANCED_FACE('',(#4905),#28754,.F.);
#30234=ADVANCED_FACE('',(#4906),#28755,.F.);
#30235=ADVANCED_FACE('',(#4907),#28756,.T.);
#30236=ADVANCED_FACE('',(#4908),#28757,.F.);
#30237=ADVANCED_FACE('',(#4909),#28758,.F.);
#30238=ADVANCED_FACE('',(#4910),#28759,.F.);
#30239=ADVANCED_FACE('',(#4911),#28760,.T.);
#30240=ADVANCED_FACE('',(#4912),#28761,.F.);
#30241=ADVANCED_FACE('',(#4913),#28762,.F.);
#30242=ADVANCED_FACE('',(#4914),#28763,.F.);
#30243=ADVANCED_FACE('',(#4915),#28764,.T.);
#30244=ADVANCED_FACE('',(#4916),#28765,.F.);
#30245=ADVANCED_FACE('',(#4917),#28766,.F.);
#30246=ADVANCED_FACE('',(#4918),#28767,.F.);
#30247=ADVANCED_FACE('',(#4919),#28768,.T.);
#30248=ADVANCED_FACE('',(#4920),#28769,.F.);
#30249=ADVANCED_FACE('',(#4921),#28770,.F.);
#30250=ADVANCED_FACE('',(#4922),#28771,.F.);
#30251=ADVANCED_FACE('',(#4923),#28772,.T.);
#30252=ADVANCED_FACE('',(#4924),#28773,.F.);
#30253=ADVANCED_FACE('',(#4925),#28774,.F.);
#30254=ADVANCED_FACE('',(#4926),#28775,.F.);
#30255=ADVANCED_FACE('',(#4927),#28776,.T.);
#30256=ADVANCED_FACE('',(#4928),#28777,.F.);
#30257=ADVANCED_FACE('',(#4929),#28778,.F.);
#30258=ADVANCED_FACE('',(#4930),#28779,.F.);
#30259=ADVANCED_FACE('',(#4931),#28780,.T.);
#30260=ADVANCED_FACE('',(#4932),#28781,.F.);
#30261=ADVANCED_FACE('',(#4933),#28782,.F.);
#30262=ADVANCED_FACE('',(#4934),#2044,.F.);
#30263=ADVANCED_FACE('',(#4935),#28783,.F.);
#30264=ADVANCED_FACE('',(#4936),#28784,.F.);
#30265=ADVANCED_FACE('',(#4937),#28785,.F.);
#30266=ADVANCED_FACE('',(#4938),#28786,.F.);
#30267=ADVANCED_FACE('',(#4939),#28787,.F.);
#30268=ADVANCED_FACE('',(#4940),#28788,.F.);
#30269=ADVANCED_FACE('',(#4941,#3527),#28789,.F.);
#30270=ADVANCED_FACE('',(#4942),#28790,.T.);
#30271=ADVANCED_FACE('',(#4943),#2045,.T.);
#30272=ADVANCED_FACE('',(#4944,#3528,#3529,#3530,#3531,#3532,#3533,#3534,
#3535,#3536,#3537,#3538,#3539,#3540,#3541,#3542,#3543,#3544,#3545,#3546,
#3547,#3548,#3549,#3550,#3551,#3552,#3553,#3554,#3555,#3556,#3557,#3558,
#3559,#3560,#3561,#3562),#806,.T.);
#30273=ADVANCED_FACE('',(#4945),#2046,.T.);
#30274=ADVANCED_FACE('',(#4946,#3563),#28791,.T.);
#30674=CLOSED_SHELL('',(#29972,#29973,#29974,#29975,#29976,#29977,#29978,
#29979,#29980,#29981,#29982,#29983,#29984,#29985,#29986,#29987,#29988,#29989,
#29990,#29991,#29992,#29993,#29994,#29995,#29996,#29997,#29998,#29999,#30000,
#30001,#30002,#30003,#30004,#30005,#30006,#30007,#30008,#30009,#30010,#30011,
#30012,#30013,#30014,#30015,#30016,#30017,#30018,#30019,#30020,#30021,#30022,
#30023,#30024,#30025,#30026,#30027,#30028,#30029,#30030,#30031,#30032,#30033,
#30034,#30035,#30036,#30037,#30038,#30039,#30040,#30041,#30042,#30043,#30044,
#30045,#30046,#30047,#30048,#30049,#30050,#30051,#30052,#30053,#30054,#30055,
#30056,#30057,#30058,#30059,#30060,#30061,#30062,#30063,#30064,#30065,#30066,
#30067,#30068,#30069,#30070,#30071,#30072,#30073,#30074,#30075,#30076,#30077,
#30078,#30079,#30080,#30081,#30082,#30083,#30084,#30085,#30086,#30087,#30088,
#30089,#30090,#30091,#30092,#30093,#30094,#30095,#30096,#30097,#30098,#30099,
#30100,#30101,#30102,#30103,#30104,#30105,#30106,#30107,#30108,#30109,#30110,
#30111,#30112,#30113,#30114,#30115,#30116,#30117,#30118,#30119,#30120,#30121,
#30122,#30123,#30124,#30125,#30126,#30127,#30128,#30129,#30130,#30131,#30132,
#30133,#30134,#30135,#30136,#30137,#30138,#30139,#30140,#30141,#30142,#30143,
#30144,#30145,#30146,#30147,#30148,#30149,#30150,#30151,#30152,#30153,#30154,
#30155,#30156,#30157,#30158,#30159,#30160,#30161,#30162,#30163,#30164,#30165,
#30166,#30167,#30168,#30169,#30170,#30171,#30172,#30173,#30174,#30175,#30176,
#30177,#30178,#30179,#30180,#30181,#30182,#30183,#30184,#30185,#30186,#30187,
#30188,#30189,#30190,#30191,#30192,#30193,#30194,#30195,#30196,#30197,#30198,
#30199,#30200,#30201,#30202,#30203,#30204,#30205,#30206,#30207,#30208,#30209,
#30210,#30211,#30212,#30213,#30214,#30215,#30216,#30217,#30218,#30219,#30220,
#30221,#30222,#30223,#30224,#30225,#30226,#30227,#30228,#30229,#30230,#30231,
#30232,#30233,#30234,#30235,#30236,#30237,#30238,#30239,#30240,#30241,#30242,
#30243,#30244,#30245,#30246,#30247,#30248,#30249,#30250,#30251,#30252,#30253,
#30254,#30255,#30256,#30257,#30258,#30259,#30260,#30261,#30262,#30263,#30264,
#30265,#30266,#30267,#30268,#30269,#30270,#30271,#30272,#30273,#30274));
#32454=AXIS2_PLACEMENT_3D('',#55997,#38004,#38005);
#32455=AXIS2_PLACEMENT_3D('',#55998,#38006,#38007);
#32456=AXIS2_PLACEMENT_3D('',#56014,#38009,#38010);
#32457=AXIS2_PLACEMENT_3D('',#56022,#38011,#38012);
#32458=AXIS2_PLACEMENT_3D('',#56070,#38014,#38015);
#32459=AXIS2_PLACEMENT_3D('',#56118,#38017,#38018);
#32460=AXIS2_PLACEMENT_3D('',#56166,#38020,#38021);
#32461=AXIS2_PLACEMENT_3D('',#56220,#38023,#38024);
#32462=AXIS2_PLACEMENT_3D('',#56268,#38026,#38027);
#32463=AXIS2_PLACEMENT_3D('',#56316,#38029,#38030);
#32464=AXIS2_PLACEMENT_3D('',#56370,#38032,#38033);
#32465=AXIS2_PLACEMENT_3D('',#56418,#38035,#38036);
#32466=AXIS2_PLACEMENT_3D('',#56466,#38038,#38039);
#32467=AXIS2_PLACEMENT_3D('',#56514,#38041,#38042);
#32468=AXIS2_PLACEMENT_3D('',#56568,#38044,#38045);
#32469=AXIS2_PLACEMENT_3D('',#56616,#38047,#38048);
#32470=AXIS2_PLACEMENT_3D('',#56664,#38050,#38051);
#32471=AXIS2_PLACEMENT_3D('',#56718,#38053,#38054);
#32472=AXIS2_PLACEMENT_3D('',#56766,#38056,#38057);
#32473=AXIS2_PLACEMENT_3D('',#56814,#38059,#38060);
#32474=AXIS2_PLACEMENT_3D('',#56862,#38062,#38063);
#32475=AXIS2_PLACEMENT_3D('',#56916,#38065,#38066);
#32476=AXIS2_PLACEMENT_3D('',#56964,#38068,#38069);
#32477=AXIS2_PLACEMENT_3D('',#57012,#38071,#38072);
#32478=AXIS2_PLACEMENT_3D('',#57066,#38074,#38075);
#32479=AXIS2_PLACEMENT_3D('',#57114,#38077,#38078);
#32480=AXIS2_PLACEMENT_3D('',#57162,#38080,#38081);
#32481=AXIS2_PLACEMENT_3D('',#57210,#38083,#38084);
#32482=AXIS2_PLACEMENT_3D('',#57264,#38086,#38087);
#32483=AXIS2_PLACEMENT_3D('',#57312,#38089,#38090);
#32484=AXIS2_PLACEMENT_3D('',#57360,#38092,#38093);
#32485=AXIS2_PLACEMENT_3D('',#57414,#38095,#38096);
#32486=AXIS2_PLACEMENT_3D('',#57462,#38098,#38099);
#32487=AXIS2_PLACEMENT_3D('',#57510,#38101,#38102);
#32488=AXIS2_PLACEMENT_3D('',#57558,#38104,#38105);
#32489=AXIS2_PLACEMENT_3D('',#57612,#38107,#38108);
#32490=AXIS2_PLACEMENT_3D('',#57660,#38110,#38111);
#32491=AXIS2_PLACEMENT_3D('',#57708,#38113,#38114);
#32492=AXIS2_PLACEMENT_3D('',#57762,#38116,#38117);
#32493=AXIS2_PLACEMENT_3D('',#57810,#38119,#38120);
#32494=AXIS2_PLACEMENT_3D('',#57858,#38122,#38123);
#32495=AXIS2_PLACEMENT_3D('',#57906,#38125,#38126);
#32496=AXIS2_PLACEMENT_3D('',#57960,#38128,#38129);
#32497=AXIS2_PLACEMENT_3D('',#58008,#38131,#38132);
#32498=AXIS2_PLACEMENT_3D('',#58056,#38134,#38135);
#32499=AXIS2_PLACEMENT_3D('',#58110,#38137,#38138);
#32500=AXIS2_PLACEMENT_3D('',#58158,#38140,#38141);
#32501=AXIS2_PLACEMENT_3D('',#58206,#38143,#38144);
#32502=AXIS2_PLACEMENT_3D('',#58254,#38146,#38147);
#32503=AXIS2_PLACEMENT_3D('',#58308,#38149,#38150);
#32504=AXIS2_PLACEMENT_3D('',#58356,#38152,#38153);
#32505=AXIS2_PLACEMENT_3D('',#58404,#38155,#38156);
#32506=AXIS2_PLACEMENT_3D('',#58458,#38158,#38159);
#32507=AXIS2_PLACEMENT_3D('',#58506,#38161,#38162);
#32508=AXIS2_PLACEMENT_3D('',#58554,#38164,#38165);
#32509=AXIS2_PLACEMENT_3D('',#58602,#38167,#38168);
#32510=AXIS2_PLACEMENT_3D('',#58656,#38170,#38171);
#32511=AXIS2_PLACEMENT_3D('',#58704,#38173,#38174);
#32512=AXIS2_PLACEMENT_3D('',#58752,#38176,#38177);
#32513=AXIS2_PLACEMENT_3D('',#58806,#38179,#38180);
#32514=AXIS2_PLACEMENT_3D('',#58854,#38182,#38183);
#32515=AXIS2_PLACEMENT_3D('',#58902,#38185,#38186);
#32516=AXIS2_PLACEMENT_3D('',#58950,#38188,#38189);
#32517=AXIS2_PLACEMENT_3D('',#59004,#38191,#38192);
#32518=AXIS2_PLACEMENT_3D('',#59052,#38194,#38195);
#32519=AXIS2_PLACEMENT_3D('',#59100,#38197,#38198);
#32520=AXIS2_PLACEMENT_3D('',#59154,#38200,#38201);
#32521=AXIS2_PLACEMENT_3D('',#59202,#38203,#38204);
#32522=AXIS2_PLACEMENT_3D('',#59250,#38206,#38207);
#32523=AXIS2_PLACEMENT_3D('',#59298,#38209,#38210);
#32524=AXIS2_PLACEMENT_3D('',#59352,#38212,#38213);
#32525=AXIS2_PLACEMENT_3D('',#59400,#38215,#38216);
#32526=AXIS2_PLACEMENT_3D('',#59411,#38218,#38219);
#32527=AXIS2_PLACEMENT_3D('',#59416,#38220,#38221);
#32528=AXIS2_PLACEMENT_3D('',#59440,#38223,#38224);
#32529=AXIS2_PLACEMENT_3D('',#59465,#38226,#38227);
#32530=AXIS2_PLACEMENT_3D('',#59490,#38229,#38230);
#32531=AXIS2_PLACEMENT_3D('',#59514,#38232,#38233);
#32532=AXIS2_PLACEMENT_3D('',#59538,#38235,#38236);
#32533=AXIS2_PLACEMENT_3D('',#59563,#38238,#38239);
#32534=AXIS2_PLACEMENT_3D('',#59588,#38241,#38242);
#32535=AXIS2_PLACEMENT_3D('',#59612,#38244,#38245);
#32536=AXIS2_PLACEMENT_3D('',#59637,#38247,#38248);
#32537=AXIS2_PLACEMENT_3D('',#59662,#38250,#38251);
#32538=AXIS2_PLACEMENT_3D('',#59686,#38253,#38254);
#32539=AXIS2_PLACEMENT_3D('',#59710,#38256,#38257);
#32540=AXIS2_PLACEMENT_3D('',#59735,#38259,#38260);
#32541=AXIS2_PLACEMENT_3D('',#59760,#38262,#38263);
#32542=AXIS2_PLACEMENT_3D('',#59784,#38265,#38266);
#32543=AXIS2_PLACEMENT_3D('',#59809,#38268,#38269);
#32544=AXIS2_PLACEMENT_3D('',#59834,#38271,#38272);
#32545=AXIS2_PLACEMENT_3D('',#59858,#38274,#38275);
#32546=AXIS2_PLACEMENT_3D('',#59882,#38277,#38278);
#32547=AXIS2_PLACEMENT_3D('',#59907,#38280,#38281);
#32548=AXIS2_PLACEMENT_3D('',#59932,#38283,#38284);
#32549=AXIS2_PLACEMENT_3D('',#59956,#38286,#38287);
#32550=AXIS2_PLACEMENT_3D('',#59981,#38289,#38290);
#32551=AXIS2_PLACEMENT_3D('',#60006,#38292,#38293);
#32552=AXIS2_PLACEMENT_3D('',#60030,#38295,#38296);
#32553=AXIS2_PLACEMENT_3D('',#60054,#38298,#38299);
#32554=AXIS2_PLACEMENT_3D('',#60079,#38301,#38302);
#32555=AXIS2_PLACEMENT_3D('',#60104,#38304,#38305);
#32556=AXIS2_PLACEMENT_3D('',#60128,#38307,#38308);
#32557=AXIS2_PLACEMENT_3D('',#60153,#38310,#38311);
#32558=AXIS2_PLACEMENT_3D('',#60178,#38313,#38314);
#32559=AXIS2_PLACEMENT_3D('',#60202,#38316,#38317);
#32560=AXIS2_PLACEMENT_3D('',#60226,#38319,#38320);
#32561=AXIS2_PLACEMENT_3D('',#60251,#38322,#38323);
#32562=AXIS2_PLACEMENT_3D('',#60276,#38325,#38326);
#32563=AXIS2_PLACEMENT_3D('',#60300,#38328,#38329);
#32564=AXIS2_PLACEMENT_3D('',#60325,#38331,#38332);
#32565=AXIS2_PLACEMENT_3D('',#60350,#38334,#38335);
#32566=AXIS2_PLACEMENT_3D('',#60374,#38337,#38338);
#32567=AXIS2_PLACEMENT_3D('',#60398,#38340,#38341);
#32568=AXIS2_PLACEMENT_3D('',#60423,#38343,#38344);
#32569=AXIS2_PLACEMENT_3D('',#60448,#38346,#38347);
#32570=AXIS2_PLACEMENT_3D('',#60472,#38349,#38350);
#32571=AXIS2_PLACEMENT_3D('',#60497,#38352,#38353);
#32572=AXIS2_PLACEMENT_3D('',#60522,#38355,#38356);
#32573=AXIS2_PLACEMENT_3D('',#60546,#38358,#38359);
#32574=AXIS2_PLACEMENT_3D('',#60570,#38361,#38362);
#32575=AXIS2_PLACEMENT_3D('',#60595,#38364,#38365);
#32576=AXIS2_PLACEMENT_3D('',#60620,#38367,#38368);
#32577=AXIS2_PLACEMENT_3D('',#60644,#38370,#38371);
#32578=AXIS2_PLACEMENT_3D('',#60669,#38373,#38374);
#32579=AXIS2_PLACEMENT_3D('',#60694,#38376,#38377);
#32580=AXIS2_PLACEMENT_3D('',#60718,#38379,#38380);
#32581=AXIS2_PLACEMENT_3D('',#60742,#38382,#38383);
#32582=AXIS2_PLACEMENT_3D('',#60767,#38385,#38386);
#32583=AXIS2_PLACEMENT_3D('',#60792,#38388,#38389);
#32584=AXIS2_PLACEMENT_3D('',#60816,#38391,#38392);
#32585=AXIS2_PLACEMENT_3D('',#60841,#38394,#38395);
#32586=AXIS2_PLACEMENT_3D('',#60866,#38397,#38398);
#32587=AXIS2_PLACEMENT_3D('',#60890,#38400,#38401);
#32588=AXIS2_PLACEMENT_3D('',#60914,#38403,#38404);
#32589=AXIS2_PLACEMENT_3D('',#60939,#38406,#38407);
#32590=AXIS2_PLACEMENT_3D('',#60964,#38409,#38410);
#32591=AXIS2_PLACEMENT_3D('',#60988,#38412,#38413);
#32592=AXIS2_PLACEMENT_3D('',#61013,#38415,#38416);
#32593=AXIS2_PLACEMENT_3D('',#61038,#38418,#38419);
#32594=AXIS2_PLACEMENT_3D('',#61062,#38421,#38422);
#32595=AXIS2_PLACEMENT_3D('',#61086,#38424,#38425);
#32596=AXIS2_PLACEMENT_3D('',#61174,#38426,#38427);
#32597=AXIS2_PLACEMENT_3D('',#61176,#38428,#38429);
#32598=AXIS2_PLACEMENT_3D('',#63122,#38430,#38431);
#32599=AXIS2_PLACEMENT_3D('',#63124,#38432,#38433);
#32600=AXIS2_PLACEMENT_3D('',#63125,#38434,#38435);
#32601=AXIS2_PLACEMENT_3D('',#63209,#38436,#38437);
#32602=AXIS2_PLACEMENT_3D('',#63210,#38438,#38439);
#32603=AXIS2_PLACEMENT_3D('',#64984,#38440,#38441);
#32604=AXIS2_PLACEMENT_3D('',#64986,#38442,#38443);
#32605=AXIS2_PLACEMENT_3D('',#64987,#38444,#38445);
#32606=AXIS2_PLACEMENT_3D('',#64988,#38446,#38447);
#32607=AXIS2_PLACEMENT_3D('',#64989,#38448,#38449);
#32608=AXIS2_PLACEMENT_3D('',#64990,#38450,#38451);
#32609=AXIS2_PLACEMENT_3D('',#64992,#38452,#38453);
#32610=AXIS2_PLACEMENT_3D('',#64993,#38454,#38455);
#32611=AXIS2_PLACEMENT_3D('',#65002,#38460,#38461);
#32612=AXIS2_PLACEMENT_3D('',#65004,#38462,#38463);
#32613=AXIS2_PLACEMENT_3D('',#65006,#38465,#38466);
#32614=AXIS2_PLACEMENT_3D('',#65010,#38469,#38470);
#32615=AXIS2_PLACEMENT_3D('',#65011,#38471,#38472);
#32616=AXIS2_PLACEMENT_3D('',#65012,#38473,#38474);
#32617=AXIS2_PLACEMENT_3D('',#65021,#38479,#38480);
#32618=AXIS2_PLACEMENT_3D('',#65023,#38481,#38482);
#32619=AXIS2_PLACEMENT_3D('',#65025,#38484,#38485);
#32620=AXIS2_PLACEMENT_3D('',#65029,#38488,#38489);
#32621=AXIS2_PLACEMENT_3D('',#65030,#38490,#38491);
#32622=AXIS2_PLACEMENT_3D('',#65031,#38492,#38493);
#32623=AXIS2_PLACEMENT_3D('',#65040,#38498,#38499);
#32624=AXIS2_PLACEMENT_3D('',#65042,#38500,#38501);
#32625=AXIS2_PLACEMENT_3D('',#65044,#38503,#38504);
#32626=AXIS2_PLACEMENT_3D('',#65048,#38507,#38508);
#32627=AXIS2_PLACEMENT_3D('',#65049,#38509,#38510);
#32628=AXIS2_PLACEMENT_3D('',#65050,#38511,#38512);
#32629=AXIS2_PLACEMENT_3D('',#65059,#38517,#38518);
#32630=AXIS2_PLACEMENT_3D('',#65061,#38519,#38520);
#32631=AXIS2_PLACEMENT_3D('',#65063,#38522,#38523);
#32632=AXIS2_PLACEMENT_3D('',#65067,#38526,#38527);
#32633=AXIS2_PLACEMENT_3D('',#65068,#38528,#38529);
#32634=AXIS2_PLACEMENT_3D('',#65069,#38530,#38531);
#32635=AXIS2_PLACEMENT_3D('',#65078,#38536,#38537);
#32636=AXIS2_PLACEMENT_3D('',#65080,#38538,#38539);
#32637=AXIS2_PLACEMENT_3D('',#65082,#38541,#38542);
#32638=AXIS2_PLACEMENT_3D('',#65086,#38545,#38546);
#32639=AXIS2_PLACEMENT_3D('',#65087,#38547,#38548);
#32640=AXIS2_PLACEMENT_3D('',#65088,#38549,#38550);
#32641=AXIS2_PLACEMENT_3D('',#65097,#38555,#38556);
#32642=AXIS2_PLACEMENT_3D('',#65099,#38557,#38558);
#32643=AXIS2_PLACEMENT_3D('',#65101,#38560,#38561);
#32644=AXIS2_PLACEMENT_3D('',#65105,#38564,#38565);
#32645=AXIS2_PLACEMENT_3D('',#65106,#38566,#38567);
#32646=AXIS2_PLACEMENT_3D('',#65107,#38568,#38569);
#32647=AXIS2_PLACEMENT_3D('',#65116,#38574,#38575);
#32648=AXIS2_PLACEMENT_3D('',#65118,#38576,#38577);
#32649=AXIS2_PLACEMENT_3D('',#65120,#38579,#38580);
#32650=AXIS2_PLACEMENT_3D('',#65124,#38583,#38584);
#32651=AXIS2_PLACEMENT_3D('',#65125,#38585,#38586);
#32652=AXIS2_PLACEMENT_3D('',#65126,#38587,#38588);
#32653=AXIS2_PLACEMENT_3D('',#65135,#38593,#38594);
#32654=AXIS2_PLACEMENT_3D('',#65137,#38595,#38596);
#32655=AXIS2_PLACEMENT_3D('',#65139,#38598,#38599);
#32656=AXIS2_PLACEMENT_3D('',#65143,#38602,#38603);
#32657=AXIS2_PLACEMENT_3D('',#65144,#38604,#38605);
#32658=AXIS2_PLACEMENT_3D('',#65145,#38606,#38607);
#32659=AXIS2_PLACEMENT_3D('',#65154,#38612,#38613);
#32660=AXIS2_PLACEMENT_3D('',#65156,#38614,#38615);
#32661=AXIS2_PLACEMENT_3D('',#65158,#38617,#38618);
#32662=AXIS2_PLACEMENT_3D('',#65162,#38621,#38622);
#32663=AXIS2_PLACEMENT_3D('',#65163,#38623,#38624);
#32664=AXIS2_PLACEMENT_3D('',#65164,#38625,#38626);
#32665=AXIS2_PLACEMENT_3D('',#65173,#38631,#38632);
#32666=AXIS2_PLACEMENT_3D('',#65175,#38633,#38634);
#32667=AXIS2_PLACEMENT_3D('',#65177,#38636,#38637);
#32668=AXIS2_PLACEMENT_3D('',#65181,#38640,#38641);
#32669=AXIS2_PLACEMENT_3D('',#65182,#38642,#38643);
#32670=AXIS2_PLACEMENT_3D('',#65183,#38644,#38645);
#32671=AXIS2_PLACEMENT_3D('',#65192,#38650,#38651);
#32672=AXIS2_PLACEMENT_3D('',#65194,#38652,#38653);
#32673=AXIS2_PLACEMENT_3D('',#65196,#38655,#38656);
#32674=AXIS2_PLACEMENT_3D('',#65200,#38659,#38660);
#32675=AXIS2_PLACEMENT_3D('',#65201,#38661,#38662);
#32676=AXIS2_PLACEMENT_3D('',#65202,#38663,#38664);
#32677=AXIS2_PLACEMENT_3D('',#65211,#38669,#38670);
#32678=AXIS2_PLACEMENT_3D('',#65213,#38671,#38672);
#32679=AXIS2_PLACEMENT_3D('',#65215,#38674,#38675);
#32680=AXIS2_PLACEMENT_3D('',#65219,#38678,#38679);
#32681=AXIS2_PLACEMENT_3D('',#65220,#38680,#38681);
#32682=AXIS2_PLACEMENT_3D('',#65221,#38682,#38683);
#32683=AXIS2_PLACEMENT_3D('',#65230,#38688,#38689);
#32684=AXIS2_PLACEMENT_3D('',#65232,#38690,#38691);
#32685=AXIS2_PLACEMENT_3D('',#65234,#38693,#38694);
#32686=AXIS2_PLACEMENT_3D('',#65238,#38697,#38698);
#32687=AXIS2_PLACEMENT_3D('',#65239,#38699,#38700);
#32688=AXIS2_PLACEMENT_3D('',#65240,#38701,#38702);
#32689=AXIS2_PLACEMENT_3D('',#65249,#38707,#38708);
#32690=AXIS2_PLACEMENT_3D('',#65251,#38709,#38710);
#32691=AXIS2_PLACEMENT_3D('',#65253,#38712,#38713);
#32692=AXIS2_PLACEMENT_3D('',#65257,#38716,#38717);
#32693=AXIS2_PLACEMENT_3D('',#65258,#38718,#38719);
#32694=AXIS2_PLACEMENT_3D('',#65259,#38720,#38721);
#32695=AXIS2_PLACEMENT_3D('',#65268,#38726,#38727);
#32696=AXIS2_PLACEMENT_3D('',#65270,#38728,#38729);
#32697=AXIS2_PLACEMENT_3D('',#65272,#38731,#38732);
#32698=AXIS2_PLACEMENT_3D('',#65276,#38735,#38736);
#32699=AXIS2_PLACEMENT_3D('',#65277,#38737,#38738);
#32700=AXIS2_PLACEMENT_3D('',#65278,#38739,#38740);
#32701=AXIS2_PLACEMENT_3D('',#65287,#38745,#38746);
#32702=AXIS2_PLACEMENT_3D('',#65289,#38747,#38748);
#32703=AXIS2_PLACEMENT_3D('',#65291,#38750,#38751);
#32704=AXIS2_PLACEMENT_3D('',#65295,#38754,#38755);
#32705=AXIS2_PLACEMENT_3D('',#65296,#38756,#38757);
#32706=AXIS2_PLACEMENT_3D('',#65297,#38758,#38759);
#32707=AXIS2_PLACEMENT_3D('',#65306,#38764,#38765);
#32708=AXIS2_PLACEMENT_3D('',#65308,#38766,#38767);
#32709=AXIS2_PLACEMENT_3D('',#65310,#38769,#38770);
#32710=AXIS2_PLACEMENT_3D('',#65314,#38773,#38774);
#32711=AXIS2_PLACEMENT_3D('',#65315,#38775,#38776);
#32712=AXIS2_PLACEMENT_3D('',#65316,#38777,#38778);
#32713=AXIS2_PLACEMENT_3D('',#65325,#38783,#38784);
#32714=AXIS2_PLACEMENT_3D('',#65327,#38785,#38786);
#32715=AXIS2_PLACEMENT_3D('',#65330,#38788,#38789);
#32716=AXIS2_PLACEMENT_3D('',#65331,#38790,#38791);
#32717=AXIS2_PLACEMENT_3D('',#65335,#38794,#38795);
#32718=AXIS2_PLACEMENT_3D('',#65337,#38796,#38797);
#32719=AXIS2_PLACEMENT_3D('',#65338,#38798,#38799);
#32720=AXIS2_PLACEMENT_3D('',#65339,#38800,#38801);
#32721=AXIS2_PLACEMENT_3D('',#65348,#38806,#38807);
#32722=AXIS2_PLACEMENT_3D('',#65350,#38808,#38809);
#32723=AXIS2_PLACEMENT_3D('',#65352,#38811,#38812);
#32724=AXIS2_PLACEMENT_3D('',#65356,#38815,#38816);
#32725=AXIS2_PLACEMENT_3D('',#65357,#38817,#38818);
#32726=AXIS2_PLACEMENT_3D('',#65358,#38819,#38820);
#32727=AXIS2_PLACEMENT_3D('',#65367,#38825,#38826);
#32728=AXIS2_PLACEMENT_3D('',#65369,#38827,#38828);
#32729=AXIS2_PLACEMENT_3D('',#65371,#38830,#38831);
#32730=AXIS2_PLACEMENT_3D('',#65375,#38834,#38835);
#32731=AXIS2_PLACEMENT_3D('',#65376,#38836,#38837);
#32732=AXIS2_PLACEMENT_3D('',#65377,#38838,#38839);
#32733=AXIS2_PLACEMENT_3D('',#65386,#38844,#38845);
#32734=AXIS2_PLACEMENT_3D('',#65388,#38846,#38847);
#32735=AXIS2_PLACEMENT_3D('',#65390,#38849,#38850);
#32736=AXIS2_PLACEMENT_3D('',#65394,#38853,#38854);
#32737=AXIS2_PLACEMENT_3D('',#65395,#38855,#38856);
#32738=AXIS2_PLACEMENT_3D('',#65396,#38857,#38858);
#32739=AXIS2_PLACEMENT_3D('',#65405,#38863,#38864);
#32740=AXIS2_PLACEMENT_3D('',#65407,#38865,#38866);
#32741=AXIS2_PLACEMENT_3D('',#65409,#38868,#38869);
#32742=AXIS2_PLACEMENT_3D('',#65413,#38872,#38873);
#32743=AXIS2_PLACEMENT_3D('',#65414,#38874,#38875);
#32744=AXIS2_PLACEMENT_3D('',#65415,#38876,#38877);
#32745=AXIS2_PLACEMENT_3D('',#65424,#38882,#38883);
#32746=AXIS2_PLACEMENT_3D('',#65426,#38884,#38885);
#32747=AXIS2_PLACEMENT_3D('',#65428,#38887,#38888);
#32748=AXIS2_PLACEMENT_3D('',#65432,#38891,#38892);
#32749=AXIS2_PLACEMENT_3D('',#65433,#38893,#38894);
#32750=AXIS2_PLACEMENT_3D('',#65434,#38895,#38896);
#32751=AXIS2_PLACEMENT_3D('',#65443,#38901,#38902);
#32752=AXIS2_PLACEMENT_3D('',#65445,#38903,#38904);
#32753=AXIS2_PLACEMENT_3D('',#65447,#38906,#38907);
#32754=AXIS2_PLACEMENT_3D('',#65451,#38910,#38911);
#32755=AXIS2_PLACEMENT_3D('',#65452,#38912,#38913);
#32756=AXIS2_PLACEMENT_3D('',#65453,#38914,#38915);
#32757=AXIS2_PLACEMENT_3D('',#65462,#38920,#38921);
#32758=AXIS2_PLACEMENT_3D('',#65464,#38922,#38923);
#32759=AXIS2_PLACEMENT_3D('',#65466,#38925,#38926);
#32760=AXIS2_PLACEMENT_3D('',#65470,#38929,#38930);
#32761=AXIS2_PLACEMENT_3D('',#65471,#38931,#38932);
#32762=AXIS2_PLACEMENT_3D('',#65472,#38933,#38934);
#32763=AXIS2_PLACEMENT_3D('',#65481,#38939,#38940);
#32764=AXIS2_PLACEMENT_3D('',#65483,#38941,#38942);
#32765=AXIS2_PLACEMENT_3D('',#65485,#38944,#38945);
#32766=AXIS2_PLACEMENT_3D('',#65489,#38948,#38949);
#32767=AXIS2_PLACEMENT_3D('',#65490,#38950,#38951);
#32768=AXIS2_PLACEMENT_3D('',#65491,#38952,#38953);
#32769=AXIS2_PLACEMENT_3D('',#65500,#38958,#38959);
#32770=AXIS2_PLACEMENT_3D('',#65502,#38960,#38961);
#32771=AXIS2_PLACEMENT_3D('',#65504,#38963,#38964);
#32772=AXIS2_PLACEMENT_3D('',#65508,#38967,#38968);
#32773=AXIS2_PLACEMENT_3D('',#65509,#38969,#38970);
#32774=AXIS2_PLACEMENT_3D('',#65510,#38971,#38972);
#32775=AXIS2_PLACEMENT_3D('',#65519,#38977,#38978);
#32776=AXIS2_PLACEMENT_3D('',#65521,#38979,#38980);
#32777=AXIS2_PLACEMENT_3D('',#65523,#38982,#38983);
#32778=AXIS2_PLACEMENT_3D('',#65527,#38986,#38987);
#32779=AXIS2_PLACEMENT_3D('',#65528,#38988,#38989);
#32780=AXIS2_PLACEMENT_3D('',#65529,#38990,#38991);
#32781=AXIS2_PLACEMENT_3D('',#65538,#38996,#38997);
#32782=AXIS2_PLACEMENT_3D('',#65540,#38998,#38999);
#32783=AXIS2_PLACEMENT_3D('',#65542,#39001,#39002);
#32784=AXIS2_PLACEMENT_3D('',#65546,#39005,#39006);
#32785=AXIS2_PLACEMENT_3D('',#65547,#39007,#39008);
#32786=AXIS2_PLACEMENT_3D('',#65548,#39009,#39010);
#32787=AXIS2_PLACEMENT_3D('',#65557,#39015,#39016);
#32788=AXIS2_PLACEMENT_3D('',#65559,#39017,#39018);
#32789=AXIS2_PLACEMENT_3D('',#65561,#39020,#39021);
#32790=AXIS2_PLACEMENT_3D('',#65565,#39024,#39025);
#32791=AXIS2_PLACEMENT_3D('',#65566,#39026,#39027);
#32792=AXIS2_PLACEMENT_3D('',#65567,#39028,#39029);
#32793=AXIS2_PLACEMENT_3D('',#65576,#39034,#39035);
#32794=AXIS2_PLACEMENT_3D('',#65578,#39036,#39037);
#32795=AXIS2_PLACEMENT_3D('',#65580,#39039,#39040);
#32796=AXIS2_PLACEMENT_3D('',#65584,#39043,#39044);
#32797=AXIS2_PLACEMENT_3D('',#65585,#39045,#39046);
#32798=AXIS2_PLACEMENT_3D('',#65586,#39047,#39048);
#32799=AXIS2_PLACEMENT_3D('',#65595,#39053,#39054);
#32800=AXIS2_PLACEMENT_3D('',#65597,#39055,#39056);
#32801=AXIS2_PLACEMENT_3D('',#65599,#39058,#39059);
#32802=AXIS2_PLACEMENT_3D('',#65603,#39062,#39063);
#32803=AXIS2_PLACEMENT_3D('',#65604,#39064,#39065);
#32804=AXIS2_PLACEMENT_3D('',#65605,#39066,#39067);
#32805=AXIS2_PLACEMENT_3D('',#65614,#39072,#39073);
#32806=AXIS2_PLACEMENT_3D('',#65616,#39074,#39075);
#32807=AXIS2_PLACEMENT_3D('',#65618,#39077,#39078);
#32808=AXIS2_PLACEMENT_3D('',#65622,#39081,#39082);
#32809=AXIS2_PLACEMENT_3D('',#65623,#39083,#39084);
#32810=AXIS2_PLACEMENT_3D('',#65624,#39085,#39086);
#32811=AXIS2_PLACEMENT_3D('',#65633,#39091,#39092);
#32812=AXIS2_PLACEMENT_3D('',#65635,#39093,#39094);
#32813=AXIS2_PLACEMENT_3D('',#65637,#39096,#39097);
#32814=AXIS2_PLACEMENT_3D('',#65641,#39100,#39101);
#32815=AXIS2_PLACEMENT_3D('',#65642,#39102,#39103);
#32816=AXIS2_PLACEMENT_3D('',#65643,#39104,#39105);
#32817=AXIS2_PLACEMENT_3D('',#65652,#39110,#39111);
#32818=AXIS2_PLACEMENT_3D('',#65654,#39112,#39113);
#32819=AXIS2_PLACEMENT_3D('',#65656,#39115,#39116);
#32820=AXIS2_PLACEMENT_3D('',#65660,#39119,#39120);
#32821=AXIS2_PLACEMENT_3D('',#65661,#39121,#39122);
#32822=AXIS2_PLACEMENT_3D('',#65662,#39123,#39124);
#32823=AXIS2_PLACEMENT_3D('',#65671,#39129,#39130);
#32824=AXIS2_PLACEMENT_3D('',#65673,#39131,#39132);
#32825=AXIS2_PLACEMENT_3D('',#65675,#39134,#39135);
#32826=AXIS2_PLACEMENT_3D('',#65679,#39138,#39139);
#32827=AXIS2_PLACEMENT_3D('',#65680,#39140,#39141);
#32828=AXIS2_PLACEMENT_3D('',#65681,#39142,#39143);
#32829=AXIS2_PLACEMENT_3D('',#65685,#39145,#39146);
#32830=AXIS2_PLACEMENT_3D('',#65686,#39147,#39148);
#32831=AXIS2_PLACEMENT_3D('',#65695,#39153,#39154);
#32832=AXIS2_PLACEMENT_3D('',#65701,#39158,#39159);
#32833=AXIS2_PLACEMENT_3D('',#65707,#39163,#39164);
#32834=AXIS2_PLACEMENT_3D('',#65713,#39168,#39169);
#32835=AXIS2_PLACEMENT_3D('',#65719,#39173,#39174);
#32836=AXIS2_PLACEMENT_3D('',#65722,#39177,#39178);
#32837=AXIS2_PLACEMENT_3D('',#65723,#39179,#39180);
#32838=AXIS2_PLACEMENT_3D('',#65725,#39181,#39182);
#32839=AXIS2_PLACEMENT_3D('',#65726,#39183,#39184);
#32840=AXIS2_PLACEMENT_3D('',#65728,#39186,#39187);
#32841=AXIS2_PLACEMENT_3D('',#65730,#39188,#39189);
#32842=AXIS2_PLACEMENT_3D('',#65733,#39192,#39193);
#32843=AXIS2_PLACEMENT_3D('',#65735,#39194,#39195);
#32844=AXIS2_PLACEMENT_3D('',#65737,#39197,#39198);
#38004=DIRECTION('axis',(0.,0.,1.));
#38005=DIRECTION('refdir',(1.,0.,0.));
#38006=DIRECTION('center_axis',(1.,0.,0.));
#38007=DIRECTION('ref_axis',(0.,1.,0.));
#38008=DIRECTION('',(-1.,0.,0.));
#38009=DIRECTION('center_axis',(1.,0.,0.));
#38010=DIRECTION('ref_axis',(0.,1.,0.));
#38011=DIRECTION('center_axis',(1.,0.,0.));
#38012=DIRECTION('ref_axis',(0.,1.,0.));
#38013=DIRECTION('',(-1.,0.,0.));
#38014=DIRECTION('center_axis',(1.,0.,0.));
#38015=DIRECTION('ref_axis',(0.,1.,0.));
#38016=DIRECTION('',(-1.,0.,0.));
#38017=DIRECTION('center_axis',(1.,0.,0.));
#38018=DIRECTION('ref_axis',(0.,1.,0.));
#38019=DIRECTION('',(-1.,0.,0.));
#38020=DIRECTION('center_axis',(1.,0.,0.));
#38021=DIRECTION('ref_axis',(0.,1.,0.));
#38022=DIRECTION('',(-1.,0.,0.));
#38023=DIRECTION('center_axis',(1.,0.,0.));
#38024=DIRECTION('ref_axis',(0.,1.,0.));
#38025=DIRECTION('',(-1.,0.,0.));
#38026=DIRECTION('center_axis',(1.,0.,0.));
#38027=DIRECTION('ref_axis',(0.,1.,0.));
#38028=DIRECTION('',(-1.,0.,0.));
#38029=DIRECTION('center_axis',(1.,0.,0.));
#38030=DIRECTION('ref_axis',(0.,1.,0.));
#38031=DIRECTION('',(-1.,0.,0.));
#38032=DIRECTION('center_axis',(1.,0.,0.));
#38033=DIRECTION('ref_axis',(0.,1.,0.));
#38034=DIRECTION('',(-1.,0.,0.));
#38035=DIRECTION('center_axis',(1.,0.,0.));
#38036=DIRECTION('ref_axis',(0.,1.,0.));
#38037=DIRECTION('',(-1.,0.,0.));
#38038=DIRECTION('center_axis',(1.,0.,0.));
#38039=DIRECTION('ref_axis',(0.,1.,0.));
#38040=DIRECTION('',(-1.,0.,0.));
#38041=DIRECTION('center_axis',(1.,0.,0.));
#38042=DIRECTION('ref_axis',(0.,1.,0.));
#38043=DIRECTION('',(-1.,0.,0.));
#38044=DIRECTION('center_axis',(1.,0.,0.));
#38045=DIRECTION('ref_axis',(0.,1.,0.));
#38046=DIRECTION('',(-1.,0.,0.));
#38047=DIRECTION('center_axis',(1.,0.,0.));
#38048=DIRECTION('ref_axis',(0.,1.,0.));
#38049=DIRECTION('',(-1.,0.,0.));
#38050=DIRECTION('center_axis',(1.,0.,0.));
#38051=DIRECTION('ref_axis',(0.,1.,0.));
#38052=DIRECTION('',(-1.,0.,0.));
#38053=DIRECTION('center_axis',(1.,0.,0.));
#38054=DIRECTION('ref_axis',(0.,1.,0.));
#38055=DIRECTION('',(-1.,0.,0.));
#38056=DIRECTION('center_axis',(1.,0.,0.));
#38057=DIRECTION('ref_axis',(0.,1.,0.));
#38058=DIRECTION('',(-1.,0.,0.));
#38059=DIRECTION('center_axis',(1.,0.,0.));
#38060=DIRECTION('ref_axis',(0.,1.,0.));
#38061=DIRECTION('',(-1.,0.,0.));
#38062=DIRECTION('center_axis',(1.,0.,0.));
#38063=DIRECTION('ref_axis',(0.,1.,0.));
#38064=DIRECTION('',(-1.,0.,0.));
#38065=DIRECTION('center_axis',(1.,0.,0.));
#38066=DIRECTION('ref_axis',(0.,1.,0.));
#38067=DIRECTION('',(-1.,0.,0.));
#38068=DIRECTION('center_axis',(1.,0.,0.));
#38069=DIRECTION('ref_axis',(0.,1.,0.));
#38070=DIRECTION('',(-1.,0.,0.));
#38071=DIRECTION('center_axis',(1.,0.,0.));
#38072=DIRECTION('ref_axis',(0.,1.,0.));
#38073=DIRECTION('',(-1.,0.,0.));
#38074=DIRECTION('center_axis',(1.,0.,0.));
#38075=DIRECTION('ref_axis',(0.,1.,0.));
#38076=DIRECTION('',(-1.,0.,0.));
#38077=DIRECTION('center_axis',(1.,0.,0.));
#38078=DIRECTION('ref_axis',(0.,1.,0.));
#38079=DIRECTION('',(-1.,0.,0.));
#38080=DIRECTION('center_axis',(1.,0.,0.));
#38081=DIRECTION('ref_axis',(0.,1.,0.));
#38082=DIRECTION('',(-1.,0.,0.));
#38083=DIRECTION('center_axis',(1.,0.,0.));
#38084=DIRECTION('ref_axis',(0.,1.,0.));
#38085=DIRECTION('',(-1.,0.,0.));
#38086=DIRECTION('center_axis',(1.,0.,0.));
#38087=DIRECTION('ref_axis',(0.,1.,0.));
#38088=DIRECTION('',(-1.,0.,0.));
#38089=DIRECTION('center_axis',(1.,0.,0.));
#38090=DIRECTION('ref_axis',(0.,1.,0.));
#38091=DIRECTION('',(-1.,0.,0.));
#38092=DIRECTION('center_axis',(1.,0.,0.));
#38093=DIRECTION('ref_axis',(0.,1.,0.));
#38094=DIRECTION('',(-1.,0.,0.));
#38095=DIRECTION('center_axis',(1.,0.,0.));
#38096=DIRECTION('ref_axis',(0.,1.,0.));
#38097=DIRECTION('',(-1.,0.,0.));
#38098=DIRECTION('center_axis',(1.,0.,0.));
#38099=DIRECTION('ref_axis',(0.,1.,0.));
#38100=DIRECTION('',(-1.,0.,0.));
#38101=DIRECTION('center_axis',(1.,0.,0.));
#38102=DIRECTION('ref_axis',(0.,1.,0.));
#38103=DIRECTION('',(-1.,0.,0.));
#38104=DIRECTION('center_axis',(1.,0.,0.));
#38105=DIRECTION('ref_axis',(0.,1.,0.));
#38106=DIRECTION('',(-1.,0.,0.));
#38107=DIRECTION('center_axis',(1.,0.,0.));
#38108=DIRECTION('ref_axis',(0.,1.,0.));
#38109=DIRECTION('',(-1.,0.,0.));
#38110=DIRECTION('center_axis',(1.,0.,0.));
#38111=DIRECTION('ref_axis',(0.,1.,0.));
#38112=DIRECTION('',(-1.,0.,0.));
#38113=DIRECTION('center_axis',(1.,0.,0.));
#38114=DIRECTION('ref_axis',(0.,1.,0.));
#38115=DIRECTION('',(-1.,0.,0.));
#38116=DIRECTION('center_axis',(1.,0.,0.));
#38117=DIRECTION('ref_axis',(0.,1.,0.));
#38118=DIRECTION('',(-1.,0.,0.));
#38119=DIRECTION('center_axis',(1.,0.,0.));
#38120=DIRECTION('ref_axis',(0.,1.,0.));
#38121=DIRECTION('',(-1.,0.,0.));
#38122=DIRECTION('center_axis',(1.,0.,0.));
#38123=DIRECTION('ref_axis',(0.,1.,0.));
#38124=DIRECTION('',(-1.,0.,0.));
#38125=DIRECTION('center_axis',(1.,0.,0.));
#38126=DIRECTION('ref_axis',(0.,1.,0.));
#38127=DIRECTION('',(-1.,0.,0.));
#38128=DIRECTION('center_axis',(1.,0.,0.));
#38129=DIRECTION('ref_axis',(0.,1.,0.));
#38130=DIRECTION('',(-1.,0.,0.));
#38131=DIRECTION('center_axis',(1.,0.,0.));
#38132=DIRECTION('ref_axis',(0.,1.,0.));
#38133=DIRECTION('',(-1.,0.,0.));
#38134=DIRECTION('center_axis',(1.,0.,0.));
#38135=DIRECTION('ref_axis',(0.,1.,0.));
#38136=DIRECTION('',(-1.,0.,0.));
#38137=DIRECTION('center_axis',(1.,0.,0.));
#38138=DIRECTION('ref_axis',(0.,1.,0.));
#38139=DIRECTION('',(-1.,0.,0.));
#38140=DIRECTION('center_axis',(1.,0.,0.));
#38141=DIRECTION('ref_axis',(0.,1.,0.));
#38142=DIRECTION('',(-1.,0.,0.));
#38143=DIRECTION('center_axis',(1.,0.,0.));
#38144=DIRECTION('ref_axis',(0.,1.,0.));
#38145=DIRECTION('',(-1.,0.,0.));
#38146=DIRECTION('center_axis',(1.,0.,0.));
#38147=DIRECTION('ref_axis',(0.,1.,0.));
#38148=DIRECTION('',(-1.,0.,0.));
#38149=DIRECTION('center_axis',(1.,0.,0.));
#38150=DIRECTION('ref_axis',(0.,1.,0.));
#38151=DIRECTION('',(-1.,0.,0.));
#38152=DIRECTION('center_axis',(1.,0.,0.));
#38153=DIRECTION('ref_axis',(0.,1.,0.));
#38154=DIRECTION('',(-1.,0.,0.));
#38155=DIRECTION('center_axis',(1.,0.,0.));
#38156=DIRECTION('ref_axis',(0.,1.,0.));
#38157=DIRECTION('',(-1.,0.,0.));
#38158=DIRECTION('center_axis',(1.,0.,0.));
#38159=DIRECTION('ref_axis',(0.,1.,0.));
#38160=DIRECTION('',(-1.,0.,0.));
#38161=DIRECTION('center_axis',(1.,0.,0.));
#38162=DIRECTION('ref_axis',(0.,1.,0.));
#38163=DIRECTION('',(-1.,0.,0.));
#38164=DIRECTION('center_axis',(1.,0.,0.));
#38165=DIRECTION('ref_axis',(0.,1.,0.));
#38166=DIRECTION('',(-1.,0.,0.));
#38167=DIRECTION('center_axis',(1.,0.,0.));
#38168=DIRECTION('ref_axis',(0.,1.,0.));
#38169=DIRECTION('',(-1.,0.,0.));
#38170=DIRECTION('center_axis',(1.,0.,0.));
#38171=DIRECTION('ref_axis',(0.,1.,0.));
#38172=DIRECTION('',(-1.,0.,0.));
#38173=DIRECTION('center_axis',(1.,0.,0.));
#38174=DIRECTION('ref_axis',(0.,1.,0.));
#38175=DIRECTION('',(-1.,0.,0.));
#38176=DIRECTION('center_axis',(1.,0.,0.));
#38177=DIRECTION('ref_axis',(0.,1.,0.));
#38178=DIRECTION('',(-1.,0.,0.));
#38179=DIRECTION('center_axis',(1.,0.,0.));
#38180=DIRECTION('ref_axis',(0.,1.,0.));
#38181=DIRECTION('',(-1.,0.,0.));
#38182=DIRECTION('center_axis',(1.,0.,0.));
#38183=DIRECTION('ref_axis',(0.,1.,0.));
#38184=DIRECTION('',(-1.,0.,0.));
#38185=DIRECTION('center_axis',(1.,0.,0.));
#38186=DIRECTION('ref_axis',(0.,1.,0.));
#38187=DIRECTION('',(-1.,0.,0.));
#38188=DIRECTION('center_axis',(1.,0.,0.));
#38189=DIRECTION('ref_axis',(0.,1.,0.));
#38190=DIRECTION('',(-1.,0.,0.));
#38191=DIRECTION('center_axis',(1.,0.,0.));
#38192=DIRECTION('ref_axis',(0.,1.,0.));
#38193=DIRECTION('',(-1.,0.,0.));
#38194=DIRECTION('center_axis',(1.,0.,0.));
#38195=DIRECTION('ref_axis',(0.,1.,0.));
#38196=DIRECTION('',(-1.,0.,0.));
#38197=DIRECTION('center_axis',(1.,0.,0.));
#38198=DIRECTION('ref_axis',(0.,1.,0.));
#38199=DIRECTION('',(-1.,0.,0.));
#38200=DIRECTION('center_axis',(1.,0.,0.));
#38201=DIRECTION('ref_axis',(0.,1.,0.));
#38202=DIRECTION('',(-1.,0.,0.));
#38203=DIRECTION('center_axis',(1.,0.,0.));
#38204=DIRECTION('ref_axis',(0.,1.,0.));
#38205=DIRECTION('',(-1.,0.,0.));
#38206=DIRECTION('center_axis',(1.,0.,0.));
#38207=DIRECTION('ref_axis',(0.,1.,0.));
#38208=DIRECTION('',(-1.,0.,0.));
#38209=DIRECTION('center_axis',(1.,0.,0.));
#38210=DIRECTION('ref_axis',(0.,1.,0.));
#38211=DIRECTION('',(-1.,0.,0.));
#38212=DIRECTION('center_axis',(1.,0.,0.));
#38213=DIRECTION('ref_axis',(0.,1.,0.));
#38214=DIRECTION('',(-1.,0.,0.));
#38215=DIRECTION('center_axis',(1.,0.,0.));
#38216=DIRECTION('ref_axis',(0.,1.,-1.17400212830891E-12));
#38217=DIRECTION('',(1.,0.,0.));
#38218=DIRECTION('center_axis',(1.,0.,0.));
#38219=DIRECTION('ref_axis',(0.,1.,-1.17400212830891E-12));
#38220=DIRECTION('center_axis',(1.,0.,0.));
#38221=DIRECTION('ref_axis',(0.,1.,-1.17400212830891E-12));
#38222=DIRECTION('',(1.,0.,0.));
#38223=DIRECTION('center_axis',(1.,0.,0.));
#38224=DIRECTION('ref_axis',(0.,1.,-1.17400212830891E-12));
#38225=DIRECTION('',(1.,0.,0.));
#38226=DIRECTION('center_axis',(1.,0.,0.));
#38227=DIRECTION('ref_axis',(0.,1.,-1.17400212830891E-12));
#38228=DIRECTION('',(1.,0.,0.));
#38229=DIRECTION('center_axis',(1.,0.,0.));
#38230=DIRECTION('ref_axis',(0.,1.,-1.17400212830891E-12));
#38231=DIRECTION('',(1.,0.,0.));
#38232=DIRECTION('center_axis',(1.,0.,0.));
#38233=DIRECTION('ref_axis',(0.,1.,-1.17400212830891E-12));
#38234=DIRECTION('',(1.,0.,0.));
#38235=DIRECTION('center_axis',(1.,0.,0.));
#38236=DIRECTION('ref_axis',(0.,1.,-1.17400212830891E-12));
#38237=DIRECTION('',(1.,0.,0.));
#38238=DIRECTION('center_axis',(1.,0.,0.));
#38239=DIRECTION('ref_axis',(0.,1.,-1.17400212830891E-12));
#38240=DIRECTION('',(1.,0.,0.));
#38241=DIRECTION('center_axis',(1.,0.,0.));
#38242=DIRECTION('ref_axis',(0.,1.,-1.17400212830891E-12));
#38243=DIRECTION('',(1.,0.,0.));
#38244=DIRECTION('center_axis',(1.,0.,0.));
#38245=DIRECTION('ref_axis',(0.,1.,-1.17400212830891E-12));
#38246=DIRECTION('',(1.,0.,0.));
#38247=DIRECTION('center_axis',(1.,0.,0.));
#38248=DIRECTION('ref_axis',(0.,1.,-1.17400212830891E-12));
#38249=DIRECTION('',(1.,0.,0.));
#38250=DIRECTION('center_axis',(1.,0.,0.));
#38251=DIRECTION('ref_axis',(0.,1.,-1.17400212830891E-12));
#38252=DIRECTION('',(1.,0.,0.));
#38253=DIRECTION('center_axis',(1.,0.,0.));
#38254=DIRECTION('ref_axis',(0.,1.,-1.17400212830891E-12));
#38255=DIRECTION('',(1.,0.,0.));
#38256=DIRECTION('center_axis',(1.,0.,0.));
#38257=DIRECTION('ref_axis',(0.,1.,-1.17400212830891E-12));
#38258=DIRECTION('',(1.,0.,0.));
#38259=DIRECTION('center_axis',(1.,0.,0.));
#38260=DIRECTION('ref_axis',(0.,1.,-1.17400212830891E-12));
#38261=DIRECTION('',(1.,0.,0.));
#38262=DIRECTION('center_axis',(1.,0.,0.));
#38263=DIRECTION('ref_axis',(0.,1.,-1.17400212830891E-12));
#38264=DIRECTION('',(1.,0.,0.));
#38265=DIRECTION('center_axis',(1.,0.,0.));
#38266=DIRECTION('ref_axis',(0.,1.,-1.17400212830891E-12));
#38267=DIRECTION('',(1.,0.,0.));
#38268=DIRECTION('center_axis',(1.,0.,0.));
#38269=DIRECTION('ref_axis',(0.,1.,-1.17400212830891E-12));
#38270=DIRECTION('',(1.,0.,0.));
#38271=DIRECTION('center_axis',(1.,0.,0.));
#38272=DIRECTION('ref_axis',(0.,1.,-1.17400212830891E-12));
#38273=DIRECTION('',(1.,0.,0.));
#38274=DIRECTION('center_axis',(1.,0.,0.));
#38275=DIRECTION('ref_axis',(0.,1.,-1.17400212830891E-12));
#38276=DIRECTION('',(1.,0.,0.));
#38277=DIRECTION('center_axis',(1.,0.,0.));
#38278=DIRECTION('ref_axis',(0.,1.,-1.17400212830891E-12));
#38279=DIRECTION('',(1.,0.,0.));
#38280=DIRECTION('center_axis',(1.,0.,0.));
#38281=DIRECTION('ref_axis',(0.,1.,-1.17400212830891E-12));
#38282=DIRECTION('',(1.,0.,0.));
#38283=DIRECTION('center_axis',(1.,0.,0.));
#38284=DIRECTION('ref_axis',(0.,1.,-1.17400212830891E-12));
#38285=DIRECTION('',(1.,0.,0.));
#38286=DIRECTION('center_axis',(1.,0.,0.));
#38287=DIRECTION('ref_axis',(0.,1.,-1.17400212830891E-12));
#38288=DIRECTION('',(1.,0.,0.));
#38289=DIRECTION('center_axis',(1.,0.,0.));
#38290=DIRECTION('ref_axis',(0.,1.,-1.17400212830891E-12));
#38291=DIRECTION('',(1.,0.,0.));
#38292=DIRECTION('center_axis',(1.,0.,0.));
#38293=DIRECTION('ref_axis',(0.,1.,-1.17400212830891E-12));
#38294=DIRECTION('',(1.,0.,0.));
#38295=DIRECTION('center_axis',(1.,0.,0.));
#38296=DIRECTION('ref_axis',(0.,1.,-1.17400212830891E-12));
#38297=DIRECTION('',(1.,0.,0.));
#38298=DIRECTION('center_axis',(1.,0.,0.));
#38299=DIRECTION('ref_axis',(0.,1.,-1.17400212830891E-12));
#38300=DIRECTION('',(1.,0.,0.));
#38301=DIRECTION('center_axis',(1.,0.,0.));
#38302=DIRECTION('ref_axis',(0.,1.,-1.17400212830891E-12));
#38303=DIRECTION('',(1.,0.,0.));
#38304=DIRECTION('center_axis',(1.,0.,0.));
#38305=DIRECTION('ref_axis',(0.,1.,-1.17400212830891E-12));
#38306=DIRECTION('',(1.,0.,0.));
#38307=DIRECTION('center_axis',(1.,0.,0.));
#38308=DIRECTION('ref_axis',(0.,1.,-1.17400212830891E-12));
#38309=DIRECTION('',(1.,0.,0.));
#38310=DIRECTION('center_axis',(1.,0.,0.));
#38311=DIRECTION('ref_axis',(0.,1.,-1.17400212830891E-12));
#38312=DIRECTION('',(1.,0.,0.));
#38313=DIRECTION('center_axis',(1.,0.,0.));
#38314=DIRECTION('ref_axis',(0.,1.,-1.17400212830891E-12));
#38315=DIRECTION('',(1.,0.,0.));
#38316=DIRECTION('center_axis',(1.,0.,0.));
#38317=DIRECTION('ref_axis',(0.,1.,-1.17400212830891E-12));
#38318=DIRECTION('',(1.,0.,0.));
#38319=DIRECTION('center_axis',(1.,0.,0.));
#38320=DIRECTION('ref_axis',(0.,1.,-1.17400212830891E-12));
#38321=DIRECTION('',(1.,0.,0.));
#38322=DIRECTION('center_axis',(1.,0.,0.));
#38323=DIRECTION('ref_axis',(0.,1.,-1.17400212830891E-12));
#38324=DIRECTION('',(1.,0.,0.));
#38325=DIRECTION('center_axis',(1.,0.,0.));
#38326=DIRECTION('ref_axis',(0.,1.,-1.17400212830891E-12));
#38327=DIRECTION('',(1.,0.,0.));
#38328=DIRECTION('center_axis',(1.,0.,0.));
#38329=DIRECTION('ref_axis',(0.,1.,-1.17400212830891E-12));
#38330=DIRECTION('',(1.,0.,0.));
#38331=DIRECTION('center_axis',(1.,0.,0.));
#38332=DIRECTION('ref_axis',(0.,1.,-1.17400212830891E-12));
#38333=DIRECTION('',(1.,0.,0.));
#38334=DIRECTION('center_axis',(1.,0.,0.));
#38335=DIRECTION('ref_axis',(0.,1.,-1.17400212830891E-12));
#38336=DIRECTION('',(1.,0.,0.));
#38337=DIRECTION('center_axis',(1.,0.,0.));
#38338=DIRECTION('ref_axis',(0.,1.,-1.17400212830891E-12));
#38339=DIRECTION('',(1.,0.,0.));
#38340=DIRECTION('center_axis',(1.,0.,0.));
#38341=DIRECTION('ref_axis',(0.,1.,-1.17400212830891E-12));
#38342=DIRECTION('',(1.,0.,0.));
#38343=DIRECTION('center_axis',(1.,0.,0.));
#38344=DIRECTION('ref_axis',(0.,1.,-1.17400212830891E-12));
#38345=DIRECTION('',(1.,0.,0.));
#38346=DIRECTION('center_axis',(1.,0.,0.));
#38347=DIRECTION('ref_axis',(0.,1.,-1.17400212830891E-12));
#38348=DIRECTION('',(1.,0.,0.));
#38349=DIRECTION('center_axis',(1.,0.,0.));
#38350=DIRECTION('ref_axis',(0.,1.,-1.17400212830891E-12));
#38351=DIRECTION('',(1.,0.,0.));
#38352=DIRECTION('center_axis',(1.,0.,0.));
#38353=DIRECTION('ref_axis',(0.,1.,-1.17400212830891E-12));
#38354=DIRECTION('',(1.,0.,0.));
#38355=DIRECTION('center_axis',(1.,0.,0.));
#38356=DIRECTION('ref_axis',(0.,1.,-1.17400212830891E-12));
#38357=DIRECTION('',(1.,0.,0.));
#38358=DIRECTION('center_axis',(1.,0.,0.));
#38359=DIRECTION('ref_axis',(0.,1.,-1.17400212830891E-12));
#38360=DIRECTION('',(1.,0.,0.));
#38361=DIRECTION('center_axis',(1.,0.,0.));
#38362=DIRECTION('ref_axis',(0.,1.,-1.17400212830891E-12));
#38363=DIRECTION('',(1.,0.,0.));
#38364=DIRECTION('center_axis',(1.,0.,0.));
#38365=DIRECTION('ref_axis',(0.,1.,-1.17400212830891E-12));
#38366=DIRECTION('',(1.,0.,0.));
#38367=DIRECTION('center_axis',(1.,0.,0.));
#38368=DIRECTION('ref_axis',(0.,1.,-1.17400212830891E-12));
#38369=DIRECTION('',(1.,0.,0.));
#38370=DIRECTION('center_axis',(1.,0.,0.));
#38371=DIRECTION('ref_axis',(0.,1.,-1.17400212830891E-12));
#38372=DIRECTION('',(1.,0.,0.));
#38373=DIRECTION('center_axis',(1.,0.,0.));
#38374=DIRECTION('ref_axis',(0.,1.,-1.17400212830891E-12));
#38375=DIRECTION('',(1.,0.,0.));
#38376=DIRECTION('center_axis',(1.,0.,0.));
#38377=DIRECTION('ref_axis',(0.,1.,-1.17400212830891E-12));
#38378=DIRECTION('',(1.,0.,0.));
#38379=DIRECTION('center_axis',(1.,0.,0.));
#38380=DIRECTION('ref_axis',(0.,1.,-1.17400212830891E-12));
#38381=DIRECTION('',(1.,0.,0.));
#38382=DIRECTION('center_axis',(1.,0.,0.));
#38383=DIRECTION('ref_axis',(0.,1.,-1.17400212830891E-12));
#38384=DIRECTION('',(1.,0.,0.));
#38385=DIRECTION('center_axis',(1.,0.,0.));
#38386=DIRECTION('ref_axis',(0.,1.,-1.17400212830891E-12));
#38387=DIRECTION('',(1.,0.,0.));
#38388=DIRECTION('center_axis',(1.,0.,0.));
#38389=DIRECTION('ref_axis',(0.,1.,-1.17400212830891E-12));
#38390=DIRECTION('',(1.,0.,0.));
#38391=DIRECTION('center_axis',(1.,0.,0.));
#38392=DIRECTION('ref_axis',(0.,1.,-1.17400212830891E-12));
#38393=DIRECTION('',(1.,0.,0.));
#38394=DIRECTION('center_axis',(1.,0.,0.));
#38395=DIRECTION('ref_axis',(0.,1.,-1.17400212830891E-12));
#38396=DIRECTION('',(1.,0.,0.));
#38397=DIRECTION('center_axis',(1.,0.,0.));
#38398=DIRECTION('ref_axis',(0.,1.,-1.17400212830891E-12));
#38399=DIRECTION('',(1.,0.,0.));
#38400=DIRECTION('center_axis',(1.,0.,0.));
#38401=DIRECTION('ref_axis',(0.,1.,-1.17400212830891E-12));
#38402=DIRECTION('',(1.,0.,0.));
#38403=DIRECTION('center_axis',(1.,0.,0.));
#38404=DIRECTION('ref_axis',(0.,1.,-1.17400212830891E-12));
#38405=DIRECTION('',(1.,0.,0.));
#38406=DIRECTION('center_axis',(1.,0.,0.));
#38407=DIRECTION('ref_axis',(0.,1.,-1.17400212830891E-12));
#38408=DIRECTION('',(1.,0.,0.));
#38409=DIRECTION('center_axis',(1.,0.,0.));
#38410=DIRECTION('ref_axis',(0.,1.,-1.17400212830891E-12));
#38411=DIRECTION('',(1.,0.,0.));
#38412=DIRECTION('center_axis',(1.,0.,0.));
#38413=DIRECTION('ref_axis',(0.,1.,-1.17400212830891E-12));
#38414=DIRECTION('',(1.,0.,0.));
#38415=DIRECTION('center_axis',(1.,0.,0.));
#38416=DIRECTION('ref_axis',(0.,1.,-1.17400212830891E-12));
#38417=DIRECTION('',(1.,0.,0.));
#38418=DIRECTION('center_axis',(1.,0.,0.));
#38419=DIRECTION('ref_axis',(0.,1.,-1.17400212830891E-12));
#38420=DIRECTION('',(1.,0.,0.));
#38421=DIRECTION('center_axis',(1.,0.,0.));
#38422=DIRECTION('ref_axis',(0.,1.,-1.17400212830891E-12));
#38423=DIRECTION('',(1.,0.,0.));
#38424=DIRECTION('center_axis',(1.,0.,0.));
#38425=DIRECTION('ref_axis',(0.,0.,-1.));
#38426=DIRECTION('center_axis',(1.,0.,0.));
#38427=DIRECTION('ref_axis',(0.,1.,0.));
#38428=DIRECTION('center_axis',(1.,0.,0.));
#38429=DIRECTION('ref_axis',(0.,1.,0.));
#38430=DIRECTION('center_axis',(1.,0.,0.));
#38431=DIRECTION('ref_axis',(0.,0.,-1.));
#38432=DIRECTION('center_axis',(1.,0.,0.));
#38433=DIRECTION('ref_axis',(0.,1.,0.));
#38434=DIRECTION('center_axis',(1.,0.,0.));
#38435=DIRECTION('ref_axis',(0.,1.,0.));
#38436=DIRECTION('center_axis',(-1.,0.,0.));
#38437=DIRECTION('ref_axis',(0.,1.,-1.17400212830891E-12));
#38438=DIRECTION('center_axis',(1.,0.,0.));
#38439=DIRECTION('ref_axis',(0.,1.,-1.17400212830891E-12));
#38440=DIRECTION('center_axis',(1.,0.,0.));
#38441=DIRECTION('ref_axis',(0.,0.,-1.));
#38442=DIRECTION('center_axis',(0.,-1.,-1.22464679914735E-16));
#38443=DIRECTION('ref_axis',(0.,-1.22464679914735E-16,1.));
#38444=DIRECTION('center_axis',(-1.,0.,0.));
#38445=DIRECTION('ref_axis',(0.,1.,0.));
#38446=DIRECTION('center_axis',(1.,0.,0.));
#38447=DIRECTION('ref_axis',(0.,1.,0.));
#38448=DIRECTION('center_axis',(1.,0.,0.));
#38449=DIRECTION('ref_axis',(0.,1.,0.));
#38450=DIRECTION('center_axis',(-1.,0.,0.));
#38451=DIRECTION('ref_axis',(0.,0.,1.));
#38452=DIRECTION('center_axis',(1.,0.,0.));
#38453=DIRECTION('ref_axis',(0.,0.,-1.));
#38454=DIRECTION('center_axis',(0.,-0.443490878258566,0.896278885672002));
#38455=DIRECTION('ref_axis',(0.,-0.896278885672002,-0.443490878258566));
#38456=DIRECTION('',(-1.,0.,0.));
#38457=DIRECTION('',(0.,-0.896278885672002,-0.443490878258566));
#38458=DIRECTION('',(1.,0.,0.));
#38459=DIRECTION('',(0.,-0.896278885672002,-0.443490878258566));
#38460=DIRECTION('center_axis',(1.,0.,0.));
#38461=DIRECTION('ref_axis',(0.,-0.17364817766693,-0.984807753012208));
#38462=DIRECTION('center_axis',(-1.,0.,0.));
#38463=DIRECTION('ref_axis',(0.,1.,0.));
#38464=DIRECTION('',(0.,0.690543841286576,-0.723290538622745));
#38465=DIRECTION('center_axis',(0.,-0.723290538622745,-0.690543841286576));
#38466=DIRECTION('ref_axis',(0.,0.690543841286576,-0.723290538622745));
#38467=DIRECTION('',(1.,0.,0.));
#38468=DIRECTION('',(0.,0.690543841286576,-0.723290538622745));
#38469=DIRECTION('center_axis',(1.,0.,0.));
#38470=DIRECTION('ref_axis',(0.,-0.17364817766693,-0.984807753012208));
#38471=DIRECTION('center_axis',(1.,0.,0.));
#38472=DIRECTION('ref_axis',(0.,1.,0.));
#38473=DIRECTION('center_axis',(0.,-0.281116060120938,0.959673778292437));
#38474=DIRECTION('ref_axis',(0.,-0.959673778292437,-0.281116060120938));
#38475=DIRECTION('',(-1.,0.,0.));
#38476=DIRECTION('',(0.,-0.959673778292437,-0.281116060120938));
#38477=DIRECTION('',(1.,0.,0.));
#38478=DIRECTION('',(0.,-0.959673778292437,-0.281116060120938));
#38479=DIRECTION('center_axis',(1.,0.,0.));
#38480=DIRECTION('ref_axis',(0.,-0.342020143325669,-0.939692620785908));
#38481=DIRECTION('center_axis',(-1.,0.,0.));
#38482=DIRECTION('ref_axis',(0.,1.,0.));
#38483=DIRECTION('',(0.,0.554454844738279,-0.832213809754591));
#38484=DIRECTION('center_axis',(0.,-0.832213809754591,-0.554454844738279));
#38485=DIRECTION('ref_axis',(0.,0.554454844738279,-0.832213809754591));
#38486=DIRECTION('',(1.,0.,0.));
#38487=DIRECTION('',(0.,0.554454844738279,-0.832213809754591));
#38488=DIRECTION('center_axis',(1.,0.,0.));
#38489=DIRECTION('ref_axis',(0.,-0.342020143325669,-0.939692620785908));
#38490=DIRECTION('center_axis',(1.,0.,0.));
#38491=DIRECTION('ref_axis',(0.,1.,0.));
#38492=DIRECTION('center_axis',(0.,-0.110199672748126,0.993909468777819));
#38493=DIRECTION('ref_axis',(0.,-0.993909468777819,-0.110199672748126));
#38494=DIRECTION('',(-1.,0.,0.));
#38495=DIRECTION('',(0.,-0.993909468777819,-0.110199672748126));
#38496=DIRECTION('',(1.,0.,0.));
#38497=DIRECTION('',(0.,-0.993909468777819,-0.110199672748126));
#38498=DIRECTION('center_axis',(1.,0.,0.));
#38499=DIRECTION('ref_axis',(0.,-0.5,-0.866025403784438));
#38500=DIRECTION('center_axis',(-1.,0.,0.));
#38501=DIRECTION('ref_axis',(0.,1.,0.));
#38502=DIRECTION('',(0.,0.401519018300299,-0.915850685397551));
#38503=DIRECTION('center_axis',(0.,-0.915850685397551,-0.401519018300299));
#38504=DIRECTION('ref_axis',(0.,0.401519018300299,-0.915850685397551));
#38505=DIRECTION('',(1.,0.,0.));
#38506=DIRECTION('',(0.,0.401519018300299,-0.915850685397551));
#38507=DIRECTION('center_axis',(1.,0.,0.));
#38508=DIRECTION('ref_axis',(0.,-0.5,-0.866025403784438));
#38509=DIRECTION('center_axis',(1.,0.,0.));
#38510=DIRECTION('ref_axis',(0.,1.,0.));
#38511=DIRECTION('center_axis',(0.,0.0640650759174117,0.997945722996845));
#38512=DIRECTION('ref_axis',(0.,-0.997945722996845,0.0640650759174117));
#38513=DIRECTION('',(-1.,0.,0.));
#38514=DIRECTION('',(0.,-0.997945722996845,0.0640650759174117));
#38515=DIRECTION('',(1.,0.,0.));
#38516=DIRECTION('',(0.,-0.997945722996845,0.0640650759174117));
#38517=DIRECTION('center_axis',(1.,0.,0.));
#38518=DIRECTION('ref_axis',(0.,-0.64278760968654,-0.766044443118978));
#38519=DIRECTION('center_axis',(-1.,0.,0.));
#38520=DIRECTION('ref_axis',(0.,1.,0.));
#38521=DIRECTION('',(0.,0.236383239669692,-0.971659901407515));
#38522=DIRECTION('center_axis',(0.,-0.971659901407515,-0.236383239669692));
#38523=DIRECTION('ref_axis',(0.,0.236383239669692,-0.971659901407515));
#38524=DIRECTION('',(1.,0.,0.));
#38525=DIRECTION('',(0.,0.236383239669692,-0.971659901407515));
#38526=DIRECTION('center_axis',(1.,0.,0.));
#38527=DIRECTION('ref_axis',(0.,-0.64278760968654,-0.766044443118978));
#38528=DIRECTION('center_axis',(1.,0.,0.));
#38529=DIRECTION('ref_axis',(0.,1.,0.));
#38530=DIRECTION('center_axis',(0.,0.236383239669692,0.971659901407515));
#38531=DIRECTION('ref_axis',(0.,-0.971659901407515,0.236383239669692));
#38532=DIRECTION('',(-1.,0.,0.));
#38533=DIRECTION('',(0.,-0.971659901407515,0.236383239669692));
#38534=DIRECTION('',(1.,0.,0.));
#38535=DIRECTION('',(0.,-0.971659901407515,0.236383239669692));
#38536=DIRECTION('center_axis',(1.,0.,0.));
#38537=DIRECTION('ref_axis',(0.,-0.766044443118978,-0.642787609686539));
#38538=DIRECTION('center_axis',(-1.,0.,0.));
#38539=DIRECTION('ref_axis',(0.,1.,0.));
#38540=DIRECTION('',(0.,0.0640650759174113,-0.997945722996845));
#38541=DIRECTION('center_axis',(0.,-0.997945722996845,-0.0640650759174113));
#38542=DIRECTION('ref_axis',(0.,0.0640650759174113,-0.997945722996845));
#38543=DIRECTION('',(1.,0.,0.));
#38544=DIRECTION('',(0.,0.0640650759174113,-0.997945722996845));
#38545=DIRECTION('center_axis',(1.,0.,0.));
#38546=DIRECTION('ref_axis',(0.,-0.766044443118978,-0.642787609686539));
#38547=DIRECTION('center_axis',(1.,0.,0.));
#38548=DIRECTION('ref_axis',(0.,1.,0.));
#38549=DIRECTION('center_axis',(0.,0.4015190183003,0.915850685397551));
#38550=DIRECTION('ref_axis',(0.,-0.915850685397551,0.401519018300299));
#38551=DIRECTION('',(-1.,0.,0.));
#38552=DIRECTION('',(0.,-0.915850685397551,0.401519018300299));
#38553=DIRECTION('',(1.,0.,0.));
#38554=DIRECTION('',(0.,-0.915850685397551,0.401519018300299));
#38555=DIRECTION('center_axis',(1.,0.,0.));
#38556=DIRECTION('ref_axis',(0.,-0.866025403784439,-0.5));
#38557=DIRECTION('center_axis',(-1.,0.,0.));
#38558=DIRECTION('ref_axis',(0.,1.,0.));
#38559=DIRECTION('',(0.,-0.110199672748127,-0.993909468777819));
#38560=DIRECTION('center_axis',(0.,-0.993909468777819,0.110199672748127));
#38561=DIRECTION('ref_axis',(0.,-0.110199672748127,-0.993909468777819));
#38562=DIRECTION('',(1.,0.,0.));
#38563=DIRECTION('',(0.,-0.110199672748127,-0.993909468777819));
#38564=DIRECTION('center_axis',(1.,0.,0.));
#38565=DIRECTION('ref_axis',(0.,-0.866025403784439,-0.5));
#38566=DIRECTION('center_axis',(1.,0.,0.));
#38567=DIRECTION('ref_axis',(0.,1.,0.));
#38568=DIRECTION('center_axis',(0.,0.55445484473828,0.832213809754591));
#38569=DIRECTION('ref_axis',(0.,-0.83221380975459,0.55445484473828));
#38570=DIRECTION('',(-1.,0.,0.));
#38571=DIRECTION('',(0.,-0.83221380975459,0.55445484473828));
#38572=DIRECTION('',(1.,0.,0.));
#38573=DIRECTION('',(0.,-0.83221380975459,0.55445484473828));
#38574=DIRECTION('center_axis',(1.,0.,0.));
#38575=DIRECTION('ref_axis',(0.,-0.939692620785909,-0.342020143325668));
#38576=DIRECTION('center_axis',(-1.,0.,0.));
#38577=DIRECTION('ref_axis',(0.,1.,0.));
#38578=DIRECTION('',(0.,-0.281116060120939,-0.959673778292436));
#38579=DIRECTION('center_axis',(0.,-0.959673778292436,0.281116060120939));
#38580=DIRECTION('ref_axis',(0.,-0.281116060120939,-0.959673778292436));
#38581=DIRECTION('',(1.,0.,0.));
#38582=DIRECTION('',(0.,-0.281116060120939,-0.959673778292436));
#38583=DIRECTION('center_axis',(1.,0.,0.));
#38584=DIRECTION('ref_axis',(0.,-0.939692620785909,-0.342020143325668));
#38585=DIRECTION('center_axis',(1.,0.,0.));
#38586=DIRECTION('ref_axis',(0.,1.,0.));
#38587=DIRECTION('center_axis',(0.,0.690543841286576,0.723290538622745));
#38588=DIRECTION('ref_axis',(0.,-0.723290538622744,0.690543841286576));
#38589=DIRECTION('',(-1.,0.,0.));
#38590=DIRECTION('',(0.,-0.723290538622744,0.690543841286576));
#38591=DIRECTION('',(1.,0.,0.));
#38592=DIRECTION('',(0.,-0.723290538622744,0.690543841286576));
#38593=DIRECTION('center_axis',(1.,0.,0.));
#38594=DIRECTION('ref_axis',(0.,-0.984807753012208,-0.17364817766693));
#38595=DIRECTION('center_axis',(-1.,0.,0.));
#38596=DIRECTION('ref_axis',(0.,1.,0.));
#38597=DIRECTION('',(0.,-0.443490878258566,-0.896278885672002));
#38598=DIRECTION('center_axis',(0.,-0.896278885672002,0.443490878258566));
#38599=DIRECTION('ref_axis',(0.,-0.443490878258566,-0.896278885672002));
#38600=DIRECTION('',(1.,0.,0.));
#38601=DIRECTION('',(0.,-0.443490878258566,-0.896278885672002));
#38602=DIRECTION('center_axis',(1.,0.,0.));
#38603=DIRECTION('ref_axis',(0.,-0.984807753012208,-0.17364817766693));
#38604=DIRECTION('center_axis',(1.,0.,0.));
#38605=DIRECTION('ref_axis',(0.,1.,0.));
#38606=DIRECTION('center_axis',(0.,0.805651012649424,0.592390450477519));
#38607=DIRECTION('ref_axis',(0.,-0.592390450477519,0.805651012649424));
#38608=DIRECTION('',(-1.,0.,0.));
#38609=DIRECTION('',(0.,-0.592390450477519,0.805651012649424));
#38610=DIRECTION('',(1.,0.,0.));
#38611=DIRECTION('',(0.,-0.592390450477519,0.805651012649424));
#38612=DIRECTION('center_axis',(1.,0.,0.));
#38613=DIRECTION('ref_axis',(0.,-1.,1.83697019872103E-16));
#38614=DIRECTION('center_axis',(-1.,0.,0.));
#38615=DIRECTION('ref_axis',(0.,1.,0.));
#38616=DIRECTION('',(0.,-0.592390450477519,-0.805651012649424));
#38617=DIRECTION('center_axis',(0.,-0.805651012649424,0.592390450477519));
#38618=DIRECTION('ref_axis',(0.,-0.592390450477519,-0.805651012649424));
#38619=DIRECTION('',(1.,0.,0.));
#38620=DIRECTION('',(0.,-0.592390450477519,-0.805651012649424));
#38621=DIRECTION('center_axis',(1.,0.,0.));
#38622=DIRECTION('ref_axis',(0.,-1.,1.83697019872103E-16));
#38623=DIRECTION('center_axis',(1.,0.,0.));
#38624=DIRECTION('ref_axis',(0.,1.,0.));
#38625=DIRECTION('center_axis',(0.,0.896278885672002,0.443490878258566));
#38626=DIRECTION('ref_axis',(0.,-0.443490878258566,0.896278885672002));
#38627=DIRECTION('',(-1.,0.,0.));
#38628=DIRECTION('',(0.,-0.443490878258566,0.896278885672002));
#38629=DIRECTION('',(1.,0.,0.));
#38630=DIRECTION('',(0.,-0.443490878258566,0.896278885672002));
#38631=DIRECTION('center_axis',(1.,0.,0.));
#38632=DIRECTION('ref_axis',(0.,-0.984807753012208,0.17364817766693));
#38633=DIRECTION('center_axis',(-1.,0.,0.));
#38634=DIRECTION('ref_axis',(0.,1.,0.));
#38635=DIRECTION('',(0.,-0.723290538622745,-0.690543841286576));
#38636=DIRECTION('center_axis',(0.,-0.690543841286576,0.723290538622745));
#38637=DIRECTION('ref_axis',(0.,-0.723290538622745,-0.690543841286576));
#38638=DIRECTION('',(1.,0.,0.));
#38639=DIRECTION('',(0.,-0.723290538622745,-0.690543841286576));
#38640=DIRECTION('center_axis',(1.,0.,0.));
#38641=DIRECTION('ref_axis',(0.,-0.984807753012208,0.17364817766693));
#38642=DIRECTION('center_axis',(1.,0.,0.));
#38643=DIRECTION('ref_axis',(0.,1.,0.));
#38644=DIRECTION('center_axis',(0.,0.959673778292437,0.281116060120938));
#38645=DIRECTION('ref_axis',(0.,-0.281116060120938,0.959673778292437));
#38646=DIRECTION('',(-1.,0.,0.));
#38647=DIRECTION('',(0.,-0.281116060120938,0.959673778292437));
#38648=DIRECTION('',(1.,0.,0.));
#38649=DIRECTION('',(0.,-0.281116060120938,0.959673778292437));
#38650=DIRECTION('center_axis',(1.,0.,0.));
#38651=DIRECTION('ref_axis',(0.,-0.939692620785908,0.342020143325669));
#38652=DIRECTION('center_axis',(-1.,0.,0.));
#38653=DIRECTION('ref_axis',(0.,1.,0.));
#38654=DIRECTION('',(0.,-0.832213809754591,-0.554454844738279));
#38655=DIRECTION('center_axis',(0.,-0.554454844738279,0.832213809754591));
#38656=DIRECTION('ref_axis',(0.,-0.832213809754591,-0.554454844738279));
#38657=DIRECTION('',(1.,0.,0.));
#38658=DIRECTION('',(0.,-0.832213809754591,-0.554454844738279));
#38659=DIRECTION('center_axis',(1.,0.,0.));
#38660=DIRECTION('ref_axis',(0.,-0.939692620785908,0.342020143325669));
#38661=DIRECTION('center_axis',(1.,0.,0.));
#38662=DIRECTION('ref_axis',(0.,1.,0.));
#38663=DIRECTION('center_axis',(0.,0.993909468777819,0.110199672748126));
#38664=DIRECTION('ref_axis',(0.,-0.110199672748126,0.993909468777819));
#38665=DIRECTION('',(-1.,0.,0.));
#38666=DIRECTION('',(0.,-0.110199672748126,0.993909468777819));
#38667=DIRECTION('',(1.,0.,0.));
#38668=DIRECTION('',(0.,-0.110199672748126,0.993909468777819));
#38669=DIRECTION('center_axis',(1.,0.,0.));
#38670=DIRECTION('ref_axis',(0.,-0.866025403784438,0.5));
#38671=DIRECTION('center_axis',(-1.,0.,0.));
#38672=DIRECTION('ref_axis',(0.,1.,0.));
#38673=DIRECTION('',(0.,-0.915850685397551,-0.401519018300299));
#38674=DIRECTION('center_axis',(0.,-0.401519018300299,0.915850685397551));
#38675=DIRECTION('ref_axis',(0.,-0.915850685397551,-0.401519018300299));
#38676=DIRECTION('',(1.,0.,0.));
#38677=DIRECTION('',(0.,-0.915850685397551,-0.401519018300299));
#38678=DIRECTION('center_axis',(1.,0.,0.));
#38679=DIRECTION('ref_axis',(0.,-0.866025403784438,0.5));
#38680=DIRECTION('center_axis',(1.,0.,0.));
#38681=DIRECTION('ref_axis',(0.,1.,0.));
#38682=DIRECTION('center_axis',(0.,0.997945722996845,-0.0640650759174116));
#38683=DIRECTION('ref_axis',(0.,0.0640650759174116,0.997945722996845));
#38684=DIRECTION('',(-1.,0.,0.));
#38685=DIRECTION('',(0.,0.0640650759174116,0.997945722996845));
#38686=DIRECTION('',(1.,0.,0.));
#38687=DIRECTION('',(0.,0.0640650759174116,0.997945722996845));
#38688=DIRECTION('center_axis',(1.,0.,0.));
#38689=DIRECTION('ref_axis',(0.,-0.766044443118978,0.642787609686539));
#38690=DIRECTION('center_axis',(-1.,0.,0.));
#38691=DIRECTION('ref_axis',(0.,1.,0.));
#38692=DIRECTION('',(0.,-0.971659901407515,-0.236383239669692));
#38693=DIRECTION('center_axis',(0.,-0.236383239669692,0.971659901407515));
#38694=DIRECTION('ref_axis',(0.,-0.971659901407515,-0.236383239669692));
#38695=DIRECTION('',(1.,0.,0.));
#38696=DIRECTION('',(0.,-0.971659901407515,-0.236383239669692));
#38697=DIRECTION('center_axis',(1.,0.,0.));
#38698=DIRECTION('ref_axis',(0.,-0.766044443118978,0.642787609686539));
#38699=DIRECTION('center_axis',(1.,0.,0.));
#38700=DIRECTION('ref_axis',(0.,1.,0.));
#38701=DIRECTION('center_axis',(0.,0.971659901407515,-0.236383239669692));
#38702=DIRECTION('ref_axis',(0.,0.236383239669692,0.971659901407515));
#38703=DIRECTION('',(-1.,0.,0.));
#38704=DIRECTION('',(0.,0.236383239669692,0.971659901407515));
#38705=DIRECTION('',(1.,0.,0.));
#38706=DIRECTION('',(0.,0.236383239669692,0.971659901407515));
#38707=DIRECTION('center_axis',(1.,0.,0.));
#38708=DIRECTION('ref_axis',(0.,-0.642787609686539,0.766044443118978));
#38709=DIRECTION('center_axis',(-1.,0.,0.));
#38710=DIRECTION('ref_axis',(0.,1.,0.));
#38711=DIRECTION('',(0.,-0.997945722996845,-0.0640650759174114));
#38712=DIRECTION('center_axis',(0.,-0.0640650759174115,0.997945722996845));
#38713=DIRECTION('ref_axis',(0.,-0.997945722996845,-0.0640650759174114));
#38714=DIRECTION('',(1.,0.,0.));
#38715=DIRECTION('',(0.,-0.997945722996845,-0.0640650759174114));
#38716=DIRECTION('center_axis',(1.,0.,0.));
#38717=DIRECTION('ref_axis',(0.,-0.642787609686539,0.766044443118978));
#38718=DIRECTION('center_axis',(1.,0.,0.));
#38719=DIRECTION('ref_axis',(0.,1.,0.));
#38720=DIRECTION('center_axis',(0.,0.915850685397551,-0.4015190183003));
#38721=DIRECTION('ref_axis',(0.,0.4015190183003,0.915850685397551));
#38722=DIRECTION('',(-1.,0.,0.));
#38723=DIRECTION('',(0.,0.4015190183003,0.915850685397551));
#38724=DIRECTION('',(1.,0.,0.));
#38725=DIRECTION('',(0.,0.4015190183003,0.915850685397551));
#38726=DIRECTION('center_axis',(1.,0.,0.));
#38727=DIRECTION('ref_axis',(0.,-0.5,0.866025403784439));
#38728=DIRECTION('center_axis',(-1.,0.,0.));
#38729=DIRECTION('ref_axis',(0.,1.,0.));
#38730=DIRECTION('',(0.,-0.993909468777818,0.110199672748127));
#38731=DIRECTION('center_axis',(0.,0.110199672748127,0.993909468777819));
#38732=DIRECTION('ref_axis',(0.,-0.993909468777818,0.110199672748127));
#38733=DIRECTION('',(1.,0.,0.));
#38734=DIRECTION('',(0.,-0.993909468777818,0.110199672748127));
#38735=DIRECTION('center_axis',(1.,0.,0.));
#38736=DIRECTION('ref_axis',(0.,-0.5,0.866025403784439));
#38737=DIRECTION('center_axis',(1.,0.,0.));
#38738=DIRECTION('ref_axis',(0.,1.,0.));
#38739=DIRECTION('center_axis',(0.,0.832213809754591,-0.55445484473828));
#38740=DIRECTION('ref_axis',(0.,0.55445484473828,0.832213809754591));
#38741=DIRECTION('',(-1.,0.,0.));
#38742=DIRECTION('',(0.,0.55445484473828,0.832213809754591));
#38743=DIRECTION('',(1.,0.,0.));
#38744=DIRECTION('',(0.,0.55445484473828,0.832213809754591));
#38745=DIRECTION('center_axis',(1.,0.,0.));
#38746=DIRECTION('ref_axis',(0.,-0.342020143325669,0.939692620785909));
#38747=DIRECTION('center_axis',(-1.,0.,0.));
#38748=DIRECTION('ref_axis',(0.,1.,0.));
#38749=DIRECTION('',(0.,-0.959673778292437,0.281116060120939));
#38750=DIRECTION('center_axis',(0.,0.281116060120939,0.959673778292437));
#38751=DIRECTION('ref_axis',(0.,-0.959673778292437,0.281116060120939));
#38752=DIRECTION('',(1.,0.,0.));
#38753=DIRECTION('',(0.,-0.959673778292437,0.281116060120939));
#38754=DIRECTION('center_axis',(1.,0.,0.));
#38755=DIRECTION('ref_axis',(0.,-0.342020143325669,0.939692620785909));
#38756=DIRECTION('center_axis',(1.,0.,0.));
#38757=DIRECTION('ref_axis',(0.,1.,0.));
#38758=DIRECTION('center_axis',(0.,0.723290538622745,-0.690543841286576));
#38759=DIRECTION('ref_axis',(0.,0.690543841286576,0.723290538622745));
#38760=DIRECTION('',(-1.,0.,0.));
#38761=DIRECTION('',(0.,0.690543841286576,0.723290538622745));
#38762=DIRECTION('',(1.,0.,0.));
#38763=DIRECTION('',(0.,0.690543841286576,0.723290538622745));
#38764=DIRECTION('center_axis',(1.,0.,0.));
#38765=DIRECTION('ref_axis',(0.,-0.17364817766693,0.984807753012208));
#38766=DIRECTION('center_axis',(-1.,0.,0.));
#38767=DIRECTION('ref_axis',(0.,1.,0.));
#38768=DIRECTION('',(0.,-0.896278885672002,0.443490878258566));
#38769=DIRECTION('center_axis',(0.,0.443490878258566,0.896278885672002));
#38770=DIRECTION('ref_axis',(0.,-0.896278885672002,0.443490878258566));
#38771=DIRECTION('',(1.,0.,0.));
#38772=DIRECTION('',(0.,-0.896278885672002,0.443490878258566));
#38773=DIRECTION('center_axis',(1.,0.,0.));
#38774=DIRECTION('ref_axis',(0.,-0.17364817766693,0.984807753012208));
#38775=DIRECTION('center_axis',(1.,0.,0.));
#38776=DIRECTION('ref_axis',(0.,1.,0.));
#38777=DIRECTION('center_axis',(0.,0.592390450477519,-0.805651012649424));
#38778=DIRECTION('ref_axis',(0.,0.805651012649424,0.592390450477519));
#38779=DIRECTION('',(-1.,0.,0.));
#38780=DIRECTION('',(0.,0.805651012649424,0.592390450477519));
#38781=DIRECTION('',(1.,0.,0.));
#38782=DIRECTION('',(0.,0.805651012649424,0.592390450477519));
#38783=DIRECTION('center_axis',(1.,0.,0.));
#38784=DIRECTION('ref_axis',(0.,1.22464679914735E-16,1.));
#38785=DIRECTION('center_axis',(-1.,0.,0.));
#38786=DIRECTION('ref_axis',(0.,1.,0.));
#38787=DIRECTION('',(0.,-0.805651012649424,0.592390450477519));
#38788=DIRECTION('center_axis',(-1.,0.,0.));
#38789=DIRECTION('ref_axis',(0.,1.,0.));
#38790=DIRECTION('center_axis',(0.,0.592390450477519,0.805651012649424));
#38791=DIRECTION('ref_axis',(0.,-0.805651012649424,0.592390450477519));
#38792=DIRECTION('',(1.,0.,0.));
#38793=DIRECTION('',(0.,-0.805651012649424,0.592390450477519));
#38794=DIRECTION('center_axis',(1.,0.,0.));
#38795=DIRECTION('ref_axis',(0.,1.22464679914735E-16,1.));
#38796=DIRECTION('center_axis',(1.,0.,0.));
#38797=DIRECTION('ref_axis',(0.,1.,0.));
#38798=DIRECTION('center_axis',(1.,0.,0.));
#38799=DIRECTION('ref_axis',(0.,1.,0.));
#38800=DIRECTION('center_axis',(0.,0.443490878258565,-0.896278885672002));
#38801=DIRECTION('ref_axis',(0.,0.896278885672002,0.443490878258565));
#38802=DIRECTION('',(-1.,0.,0.));
#38803=DIRECTION('',(0.,0.896278885672002,0.443490878258565));
#38804=DIRECTION('',(1.,0.,0.));
#38805=DIRECTION('',(0.,0.896278885672002,0.443490878258565));
#38806=DIRECTION('center_axis',(1.,0.,0.));
#38807=DIRECTION('ref_axis',(0.,0.173648177666931,0.984807753012208));
#38808=DIRECTION('center_axis',(-1.,0.,0.));
#38809=DIRECTION('ref_axis',(0.,1.,0.));
#38810=DIRECTION('',(0.,-0.690543841286576,0.723290538622745));
#38811=DIRECTION('center_axis',(0.,0.723290538622745,0.690543841286576));
#38812=DIRECTION('ref_axis',(0.,-0.690543841286576,0.723290538622745));
#38813=DIRECTION('',(1.,0.,0.));
#38814=DIRECTION('',(0.,-0.690543841286576,0.723290538622745));
#38815=DIRECTION('center_axis',(1.,0.,0.));
#38816=DIRECTION('ref_axis',(0.,0.173648177666931,0.984807753012208));
#38817=DIRECTION('center_axis',(1.,0.,0.));
#38818=DIRECTION('ref_axis',(0.,1.,0.));
#38819=DIRECTION('center_axis',(0.,0.281116060120939,-0.959673778292437));
#38820=DIRECTION('ref_axis',(0.,0.959673778292437,0.281116060120938));
#38821=DIRECTION('',(-1.,0.,0.));
#38822=DIRECTION('',(0.,0.959673778292437,0.281116060120938));
#38823=DIRECTION('',(1.,0.,0.));
#38824=DIRECTION('',(0.,0.959673778292437,0.281116060120938));
#38825=DIRECTION('center_axis',(1.,0.,0.));
#38826=DIRECTION('ref_axis',(0.,0.342020143325669,0.939692620785908));
#38827=DIRECTION('center_axis',(-1.,0.,0.));
#38828=DIRECTION('ref_axis',(0.,1.,0.));
#38829=DIRECTION('',(0.,-0.554454844738279,0.832213809754591));
#38830=DIRECTION('center_axis',(0.,0.832213809754591,0.55445484473828));
#38831=DIRECTION('ref_axis',(0.,-0.554454844738279,0.832213809754591));
#38832=DIRECTION('',(1.,0.,0.));
#38833=DIRECTION('',(0.,-0.554454844738279,0.832213809754591));
#38834=DIRECTION('center_axis',(1.,0.,0.));
#38835=DIRECTION('ref_axis',(0.,0.342020143325669,0.939692620785908));
#38836=DIRECTION('center_axis',(1.,0.,0.));
#38837=DIRECTION('ref_axis',(0.,1.,0.));
#38838=DIRECTION('center_axis',(0.,0.110199672748127,-0.993909468777819));
#38839=DIRECTION('ref_axis',(0.,0.993909468777819,0.110199672748127));
#38840=DIRECTION('',(-1.,0.,0.));
#38841=DIRECTION('',(0.,0.993909468777819,0.110199672748127));
#38842=DIRECTION('',(1.,0.,0.));
#38843=DIRECTION('',(0.,0.993909468777819,0.110199672748127));
#38844=DIRECTION('center_axis',(1.,0.,0.));
#38845=DIRECTION('ref_axis',(0.,0.5,0.866025403784439));
#38846=DIRECTION('center_axis',(-1.,0.,0.));
#38847=DIRECTION('ref_axis',(0.,1.,0.));
#38848=DIRECTION('',(0.,-0.4015190183003,0.915850685397551));
#38849=DIRECTION('center_axis',(0.,0.915850685397551,0.4015190183003));
#38850=DIRECTION('ref_axis',(0.,-0.4015190183003,0.915850685397551));
#38851=DIRECTION('',(1.,0.,0.));
#38852=DIRECTION('',(0.,-0.4015190183003,0.915850685397551));
#38853=DIRECTION('center_axis',(1.,0.,0.));
#38854=DIRECTION('ref_axis',(0.,0.5,0.866025403784439));
#38855=DIRECTION('center_axis',(1.,0.,0.));
#38856=DIRECTION('ref_axis',(0.,1.,0.));
#38857=DIRECTION('center_axis',(0.,-0.0640650759174116,-0.997945722996845));
#38858=DIRECTION('ref_axis',(0.,0.997945722996845,-0.0640650759174116));
#38859=DIRECTION('',(-1.,0.,0.));
#38860=DIRECTION('',(0.,0.997945722996845,-0.0640650759174116));
#38861=DIRECTION('',(1.,0.,0.));
#38862=DIRECTION('',(0.,0.997945722996845,-0.0640650759174116));
#38863=DIRECTION('center_axis',(1.,0.,0.));
#38864=DIRECTION('ref_axis',(0.,0.642787609686539,0.766044443118978));
#38865=DIRECTION('center_axis',(-1.,0.,0.));
#38866=DIRECTION('ref_axis',(0.,1.,0.));
#38867=DIRECTION('',(0.,-0.236383239669692,0.971659901407515));
#38868=DIRECTION('center_axis',(0.,0.971659901407515,0.236383239669692));
#38869=DIRECTION('ref_axis',(0.,-0.236383239669692,0.971659901407515));
#38870=DIRECTION('',(1.,0.,0.));
#38871=DIRECTION('',(0.,-0.236383239669692,0.971659901407515));
#38872=DIRECTION('center_axis',(1.,0.,0.));
#38873=DIRECTION('ref_axis',(0.,0.642787609686539,0.766044443118978));
#38874=DIRECTION('center_axis',(1.,0.,0.));
#38875=DIRECTION('ref_axis',(0.,1.,0.));
#38876=DIRECTION('center_axis',(0.,-0.236383239669692,-0.971659901407515));
#38877=DIRECTION('ref_axis',(0.,0.971659901407515,-0.236383239669692));
#38878=DIRECTION('',(-1.,0.,0.));
#38879=DIRECTION('',(0.,0.971659901407515,-0.236383239669692));
#38880=DIRECTION('',(1.,0.,0.));
#38881=DIRECTION('',(0.,0.971659901407515,-0.236383239669692));
#38882=DIRECTION('center_axis',(1.,0.,0.));
#38883=DIRECTION('ref_axis',(0.,0.766044443118978,0.642787609686539));
#38884=DIRECTION('center_axis',(-1.,0.,0.));
#38885=DIRECTION('ref_axis',(0.,1.,0.));
#38886=DIRECTION('',(0.,-0.0640650759174115,0.997945722996845));
#38887=DIRECTION('center_axis',(0.,0.997945722996845,0.0640650759174115));
#38888=DIRECTION('ref_axis',(0.,-0.0640650759174115,0.997945722996845));
#38889=DIRECTION('',(1.,0.,0.));
#38890=DIRECTION('',(0.,-0.0640650759174115,0.997945722996845));
#38891=DIRECTION('center_axis',(1.,0.,0.));
#38892=DIRECTION('ref_axis',(0.,0.766044443118978,0.642787609686539));
#38893=DIRECTION('center_axis',(1.,0.,0.));
#38894=DIRECTION('ref_axis',(0.,1.,0.));
#38895=DIRECTION('center_axis',(0.,-0.4015190183003,-0.915850685397551));
#38896=DIRECTION('ref_axis',(0.,0.915850685397551,-0.4015190183003));
#38897=DIRECTION('',(-1.,0.,0.));
#38898=DIRECTION('',(0.,0.915850685397551,-0.4015190183003));
#38899=DIRECTION('',(1.,0.,0.));
#38900=DIRECTION('',(0.,0.915850685397551,-0.4015190183003));
#38901=DIRECTION('center_axis',(1.,0.,0.));
#38902=DIRECTION('ref_axis',(0.,0.866025403784439,0.5));
#38903=DIRECTION('center_axis',(-1.,0.,0.));
#38904=DIRECTION('ref_axis',(0.,1.,0.));
#38905=DIRECTION('',(0.,0.110199672748127,0.993909468777819));
#38906=DIRECTION('center_axis',(0.,0.993909468777819,-0.110199672748127));
#38907=DIRECTION('ref_axis',(0.,0.110199672748127,0.993909468777819));
#38908=DIRECTION('',(1.,0.,0.));
#38909=DIRECTION('',(0.,0.110199672748127,0.993909468777819));
#38910=DIRECTION('center_axis',(1.,0.,0.));
#38911=DIRECTION('ref_axis',(0.,0.866025403784439,0.5));
#38912=DIRECTION('center_axis',(1.,0.,0.));
#38913=DIRECTION('ref_axis',(0.,1.,0.));
#38914=DIRECTION('center_axis',(0.,-0.55445484473828,-0.832213809754591));
#38915=DIRECTION('ref_axis',(0.,0.832213809754591,-0.554454844738279));
#38916=DIRECTION('',(-1.,0.,0.));
#38917=DIRECTION('',(0.,0.832213809754591,-0.554454844738279));
#38918=DIRECTION('',(1.,0.,0.));
#38919=DIRECTION('',(0.,0.832213809754591,-0.554454844738279));
#38920=DIRECTION('center_axis',(1.,0.,0.));
#38921=DIRECTION('ref_axis',(0.,0.939692620785908,0.342020143325669));
#38922=DIRECTION('center_axis',(-1.,0.,0.));
#38923=DIRECTION('ref_axis',(0.,1.,0.));
#38924=DIRECTION('',(0.,0.281116060120939,0.959673778292437));
#38925=DIRECTION('center_axis',(0.,0.959673778292437,-0.281116060120939));
#38926=DIRECTION('ref_axis',(0.,0.281116060120939,0.959673778292437));
#38927=DIRECTION('',(1.,0.,0.));
#38928=DIRECTION('',(0.,0.281116060120939,0.959673778292437));
#38929=DIRECTION('center_axis',(1.,0.,0.));
#38930=DIRECTION('ref_axis',(0.,0.939692620785908,0.342020143325669));
#38931=DIRECTION('center_axis',(1.,0.,0.));
#38932=DIRECTION('ref_axis',(0.,1.,0.));
#38933=DIRECTION('center_axis',(0.,-0.690543841286576,-0.723290538622745));
#38934=DIRECTION('ref_axis',(0.,0.723290538622745,-0.690543841286576));
#38935=DIRECTION('',(-1.,0.,0.));
#38936=DIRECTION('',(0.,0.723290538622745,-0.690543841286576));
#38937=DIRECTION('',(1.,0.,0.));
#38938=DIRECTION('',(0.,0.723290538622745,-0.690543841286576));
#38939=DIRECTION('center_axis',(1.,0.,0.));
#38940=DIRECTION('ref_axis',(0.,0.984807753012208,0.17364817766693));
#38941=DIRECTION('center_axis',(-1.,0.,0.));
#38942=DIRECTION('ref_axis',(0.,1.,0.));
#38943=DIRECTION('',(0.,0.443490878258566,0.896278885672002));
#38944=DIRECTION('center_axis',(0.,0.896278885672002,-0.443490878258566));
#38945=DIRECTION('ref_axis',(0.,0.443490878258566,0.896278885672002));
#38946=DIRECTION('',(1.,0.,0.));
#38947=DIRECTION('',(0.,0.443490878258566,0.896278885672002));
#38948=DIRECTION('center_axis',(1.,0.,0.));
#38949=DIRECTION('ref_axis',(0.,0.984807753012208,0.17364817766693));
#38950=DIRECTION('center_axis',(1.,0.,0.));
#38951=DIRECTION('ref_axis',(0.,1.,0.));
#38952=DIRECTION('center_axis',(0.,-0.805651012649424,-0.592390450477519));
#38953=DIRECTION('ref_axis',(0.,0.592390450477519,-0.805651012649424));
#38954=DIRECTION('',(-1.,0.,0.));
#38955=DIRECTION('',(0.,0.592390450477519,-0.805651012649424));
#38956=DIRECTION('',(1.,0.,0.));
#38957=DIRECTION('',(0.,0.592390450477519,-0.805651012649424));
#38958=DIRECTION('center_axis',(1.,0.,0.));
#38959=DIRECTION('ref_axis',(0.,1.,-6.12323399573677E-17));
#38960=DIRECTION('center_axis',(-1.,0.,0.));
#38961=DIRECTION('ref_axis',(0.,1.,0.));
#38962=DIRECTION('',(0.,0.592390450477519,0.805651012649424));
#38963=DIRECTION('center_axis',(0.,0.805651012649424,-0.592390450477519));
#38964=DIRECTION('ref_axis',(0.,0.592390450477519,0.805651012649424));
#38965=DIRECTION('',(1.,0.,0.));
#38966=DIRECTION('',(0.,0.592390450477519,0.805651012649424));
#38967=DIRECTION('center_axis',(1.,0.,0.));
#38968=DIRECTION('ref_axis',(0.,1.,-6.12323399573677E-17));
#38969=DIRECTION('center_axis',(1.,0.,0.));
#38970=DIRECTION('ref_axis',(0.,1.,0.));
#38971=DIRECTION('center_axis',(0.,-0.896278885672002,-0.443490878258566));
#38972=DIRECTION('ref_axis',(0.,0.443490878258566,-0.896278885672002));
#38973=DIRECTION('',(-1.,0.,0.));
#38974=DIRECTION('',(0.,0.443490878258566,-0.896278885672002));
#38975=DIRECTION('',(1.,0.,0.));
#38976=DIRECTION('',(0.,0.443490878258566,-0.896278885672002));
#38977=DIRECTION('center_axis',(1.,0.,0.));
#38978=DIRECTION('ref_axis',(0.,0.984807753012208,-0.17364817766693));
#38979=DIRECTION('center_axis',(-1.,0.,0.));
#38980=DIRECTION('ref_axis',(0.,1.,0.));
#38981=DIRECTION('',(0.,0.723290538622745,0.690543841286576));
#38982=DIRECTION('center_axis',(0.,0.690543841286576,-0.723290538622745));
#38983=DIRECTION('ref_axis',(0.,0.723290538622745,0.690543841286576));
#38984=DIRECTION('',(1.,0.,0.));
#38985=DIRECTION('',(0.,0.723290538622745,0.690543841286576));
#38986=DIRECTION('center_axis',(1.,0.,0.));
#38987=DIRECTION('ref_axis',(0.,0.984807753012208,-0.17364817766693));
#38988=DIRECTION('center_axis',(1.,0.,0.));
#38989=DIRECTION('ref_axis',(0.,1.,0.));
#38990=DIRECTION('center_axis',(0.,-0.959673778292437,-0.281116060120939));
#38991=DIRECTION('ref_axis',(0.,0.281116060120939,-0.959673778292437));
#38992=DIRECTION('',(-1.,0.,0.));
#38993=DIRECTION('',(0.,0.281116060120939,-0.959673778292437));
#38994=DIRECTION('',(1.,0.,0.));
#38995=DIRECTION('',(0.,0.281116060120939,-0.959673778292437));
#38996=DIRECTION('center_axis',(1.,0.,0.));
#38997=DIRECTION('ref_axis',(0.,0.939692620785908,-0.342020143325669));
#38998=DIRECTION('center_axis',(-1.,0.,0.));
#38999=DIRECTION('ref_axis',(0.,1.,0.));
#39000=DIRECTION('',(0.,0.832213809754591,0.554454844738279));
#39001=DIRECTION('center_axis',(0.,0.55445484473828,-0.832213809754591));
#39002=DIRECTION('ref_axis',(0.,0.832213809754591,0.554454844738279));
#39003=DIRECTION('',(1.,0.,0.));
#39004=DIRECTION('',(0.,0.832213809754591,0.554454844738279));
#39005=DIRECTION('center_axis',(1.,0.,0.));
#39006=DIRECTION('ref_axis',(0.,0.939692620785908,-0.342020143325669));
#39007=DIRECTION('center_axis',(1.,0.,0.));
#39008=DIRECTION('ref_axis',(0.,1.,0.));
#39009=DIRECTION('center_axis',(0.,-0.993909468777819,-0.110199672748127));
#39010=DIRECTION('ref_axis',(0.,0.110199672748127,-0.993909468777819));
#39011=DIRECTION('',(-1.,0.,0.));
#39012=DIRECTION('',(0.,0.110199672748127,-0.993909468777819));
#39013=DIRECTION('',(1.,0.,0.));
#39014=DIRECTION('',(0.,0.110199672748127,-0.993909468777819));
#39015=DIRECTION('center_axis',(1.,0.,0.));
#39016=DIRECTION('ref_axis',(0.,0.866025403784439,-0.5));
#39017=DIRECTION('center_axis',(-1.,0.,0.));
#39018=DIRECTION('ref_axis',(0.,1.,0.));
#39019=DIRECTION('',(0.,0.915850685397551,0.401519018300299));
#39020=DIRECTION('center_axis',(0.,0.4015190183003,-0.915850685397551));
#39021=DIRECTION('ref_axis',(0.,0.915850685397551,0.401519018300299));
#39022=DIRECTION('',(1.,0.,0.));
#39023=DIRECTION('',(0.,0.915850685397551,0.401519018300299));
#39024=DIRECTION('center_axis',(1.,0.,0.));
#39025=DIRECTION('ref_axis',(0.,0.866025403784439,-0.5));
#39026=DIRECTION('center_axis',(1.,0.,0.));
#39027=DIRECTION('ref_axis',(0.,1.,0.));
#39028=DIRECTION('center_axis',(0.,-0.997945722996845,0.0640650759174115));
#39029=DIRECTION('ref_axis',(0.,-0.0640650759174115,-0.997945722996845));
#39030=DIRECTION('',(-1.,0.,0.));
#39031=DIRECTION('',(0.,-0.0640650759174115,-0.997945722996845));
#39032=DIRECTION('',(1.,0.,0.));
#39033=DIRECTION('',(0.,-0.0640650759174115,-0.997945722996845));
#39034=DIRECTION('center_axis',(1.,0.,0.));
#39035=DIRECTION('ref_axis',(0.,0.766044443118978,-0.642787609686539));
#39036=DIRECTION('center_axis',(-1.,0.,0.));
#39037=DIRECTION('ref_axis',(0.,1.,0.));
#39038=DIRECTION('',(0.,0.971659901407514,0.236383239669692));
#39039=DIRECTION('center_axis',(0.,0.236383239669692,-0.971659901407515));
#39040=DIRECTION('ref_axis',(0.,0.971659901407515,0.236383239669692));
#39041=DIRECTION('',(1.,0.,0.));
#39042=DIRECTION('',(0.,0.971659901407514,0.236383239669692));
#39043=DIRECTION('center_axis',(1.,0.,0.));
#39044=DIRECTION('ref_axis',(0.,0.766044443118978,-0.642787609686539));
#39045=DIRECTION('center_axis',(1.,0.,0.));
#39046=DIRECTION('ref_axis',(0.,1.,0.));
#39047=DIRECTION('center_axis',(0.,-0.971659901407515,0.236383239669692));
#39048=DIRECTION('ref_axis',(0.,-0.236383239669692,-0.971659901407515));
#39049=DIRECTION('',(-1.,0.,0.));
#39050=DIRECTION('',(0.,-0.236383239669692,-0.971659901407515));
#39051=DIRECTION('',(1.,0.,0.));
#39052=DIRECTION('',(0.,-0.236383239669692,-0.971659901407515));
#39053=DIRECTION('center_axis',(1.,0.,0.));
#39054=DIRECTION('ref_axis',(0.,0.642787609686539,-0.766044443118978));
#39055=DIRECTION('center_axis',(-1.,0.,0.));
#39056=DIRECTION('ref_axis',(0.,1.,0.));
#39057=DIRECTION('',(0.,0.997945722996845,0.0640650759174114));
#39058=DIRECTION('center_axis',(0.,0.0640650759174115,-0.997945722996845));
#39059=DIRECTION('ref_axis',(0.,0.997945722996845,0.0640650759174114));
#39060=DIRECTION('',(1.,0.,0.));
#39061=DIRECTION('',(0.,0.997945722996845,0.0640650759174114));
#39062=DIRECTION('center_axis',(1.,0.,0.));
#39063=DIRECTION('ref_axis',(0.,0.642787609686539,-0.766044443118978));
#39064=DIRECTION('center_axis',(1.,0.,0.));
#39065=DIRECTION('ref_axis',(0.,1.,0.));
#39066=DIRECTION('center_axis',(0.,-0.915850685397551,0.4015190183003));
#39067=DIRECTION('ref_axis',(0.,-0.4015190183003,-0.915850685397551));
#39068=DIRECTION('',(-1.,0.,0.));
#39069=DIRECTION('',(0.,-0.4015190183003,-0.915850685397551));
#39070=DIRECTION('',(1.,0.,0.));
#39071=DIRECTION('',(0.,-0.4015190183003,-0.915850685397551));
#39072=DIRECTION('center_axis',(1.,0.,0.));
#39073=DIRECTION('ref_axis',(0.,0.5,-0.866025403784439));
#39074=DIRECTION('center_axis',(-1.,0.,0.));
#39075=DIRECTION('ref_axis',(0.,1.,0.));
#39076=DIRECTION('',(0.,0.993909468777819,-0.110199672748127));
#39077=DIRECTION('center_axis',(0.,-0.110199672748127,-0.993909468777819));
#39078=DIRECTION('ref_axis',(0.,0.993909468777819,-0.110199672748127));
#39079=DIRECTION('',(1.,0.,0.));
#39080=DIRECTION('',(0.,0.993909468777819,-0.110199672748127));
#39081=DIRECTION('center_axis',(1.,0.,0.));
#39082=DIRECTION('ref_axis',(0.,0.5,-0.866025403784439));
#39083=DIRECTION('center_axis',(1.,0.,0.));
#39084=DIRECTION('ref_axis',(0.,1.,0.));
#39085=DIRECTION('center_axis',(0.,-0.832213809754591,0.55445484473828));
#39086=DIRECTION('ref_axis',(0.,-0.554454844738279,-0.832213809754591));
#39087=DIRECTION('',(-1.,0.,0.));
#39088=DIRECTION('',(0.,-0.554454844738279,-0.832213809754591));
#39089=DIRECTION('',(1.,0.,0.));
#39090=DIRECTION('',(0.,-0.554454844738279,-0.832213809754591));
#39091=DIRECTION('center_axis',(1.,0.,0.));
#39092=DIRECTION('ref_axis',(0.,0.342020143325669,-0.939692620785908));
#39093=DIRECTION('center_axis',(-1.,0.,0.));
#39094=DIRECTION('ref_axis',(0.,1.,0.));
#39095=DIRECTION('',(0.,0.959673778292437,-0.281116060120939));
#39096=DIRECTION('center_axis',(0.,-0.281116060120939,-0.959673778292437));
#39097=DIRECTION('ref_axis',(0.,0.959673778292437,-0.281116060120939));
#39098=DIRECTION('',(1.,0.,0.));
#39099=DIRECTION('',(0.,0.959673778292437,-0.281116060120939));
#39100=DIRECTION('center_axis',(1.,0.,0.));
#39101=DIRECTION('ref_axis',(0.,0.342020143325669,-0.939692620785908));
#39102=DIRECTION('center_axis',(1.,0.,0.));
#39103=DIRECTION('ref_axis',(0.,1.,0.));
#39104=DIRECTION('center_axis',(0.,-0.723290538622745,0.690543841286576));
#39105=DIRECTION('ref_axis',(0.,-0.690543841286576,-0.723290538622745));
#39106=DIRECTION('',(-1.,0.,0.));
#39107=DIRECTION('',(0.,-0.690543841286576,-0.723290538622745));
#39108=DIRECTION('',(1.,0.,0.));
#39109=DIRECTION('',(0.,-0.690543841286576,-0.723290538622745));
#39110=DIRECTION('center_axis',(1.,0.,0.));
#39111=DIRECTION('ref_axis',(0.,0.17364817766693,-0.984807753012208));
#39112=DIRECTION('center_axis',(-1.,0.,0.));
#39113=DIRECTION('ref_axis',(0.,1.,0.));
#39114=DIRECTION('',(0.,0.896278885672002,-0.443490878258566));
#39115=DIRECTION('center_axis',(0.,-0.443490878258566,-0.896278885672002));
#39116=DIRECTION('ref_axis',(0.,0.896278885672002,-0.443490878258566));
#39117=DIRECTION('',(1.,0.,0.));
#39118=DIRECTION('',(0.,0.896278885672002,-0.443490878258566));
#39119=DIRECTION('center_axis',(1.,0.,0.));
#39120=DIRECTION('ref_axis',(0.,0.17364817766693,-0.984807753012208));
#39121=DIRECTION('center_axis',(1.,0.,0.));
#39122=DIRECTION('ref_axis',(0.,1.,0.));
#39123=DIRECTION('center_axis',(0.,-0.592390450477519,0.805651012649424));
#39124=DIRECTION('ref_axis',(0.,-0.805651012649424,-0.592390450477519));
#39125=DIRECTION('',(-1.,0.,0.));
#39126=DIRECTION('',(0.,-0.805651012649424,-0.592390450477519));
#39127=DIRECTION('',(1.,0.,0.));
#39128=DIRECTION('',(0.,-0.805651012649424,-0.592390450477519));
#39129=DIRECTION('center_axis',(1.,0.,0.));
#39130=DIRECTION('ref_axis',(0.,0.,-1.));
#39131=DIRECTION('center_axis',(-1.,0.,0.));
#39132=DIRECTION('ref_axis',(0.,1.,0.));
#39133=DIRECTION('',(0.,0.805651012649424,-0.592390450477519));
#39134=DIRECTION('center_axis',(0.,-0.592390450477519,-0.805651012649424));
#39135=DIRECTION('ref_axis',(0.,0.805651012649424,-0.592390450477519));
#39136=DIRECTION('',(1.,0.,0.));
#39137=DIRECTION('',(0.,0.805651012649424,-0.592390450477519));
#39138=DIRECTION('center_axis',(1.,0.,0.));
#39139=DIRECTION('ref_axis',(0.,0.,-1.));
#39140=DIRECTION('center_axis',(1.,0.,0.));
#39141=DIRECTION('ref_axis',(0.,1.,0.));
#39142=DIRECTION('center_axis',(1.,0.,0.));
#39143=DIRECTION('ref_axis',(0.,1.,0.));
#39144=DIRECTION('',(0.520049754552021,-0.854135968561436,-1.04601487993539E-16));
#39145=DIRECTION('center_axis',(-1.,0.,0.));
#39146=DIRECTION('ref_axis',(0.,1.,0.));
#39147=DIRECTION('center_axis',(0.,0.5,0.866025403784439));
#39148=DIRECTION('ref_axis',(0.,0.866025403784439,-0.5));
#39149=DIRECTION('',(0.,0.866025403784439,-0.5));
#39150=DIRECTION('',(-1.,0.,0.));
#39151=DIRECTION('',(0.,0.866025403784439,-0.5));
#39152=DIRECTION('',(-1.,0.,0.));
#39153=DIRECTION('center_axis',(0.,-0.5,0.866025403784439));
#39154=DIRECTION('ref_axis',(0.,0.866025403784439,0.5));
#39155=DIRECTION('',(0.,0.866025403784439,0.5));
#39156=DIRECTION('',(-1.,0.,0.));
#39157=DIRECTION('',(0.,0.866025403784439,0.5));
#39158=DIRECTION('center_axis',(0.,-1.,-1.92296268638356E-16));
#39159=DIRECTION('ref_axis',(0.,-1.92296268638356E-16,1.));
#39160=DIRECTION('',(0.,-1.92296268638356E-16,1.));
#39161=DIRECTION('',(-1.,0.,0.));
#39162=DIRECTION('',(0.,-1.92296268638356E-16,1.));
#39163=DIRECTION('center_axis',(0.,-0.5,-0.866025403784439));
#39164=DIRECTION('ref_axis',(0.,-0.866025403784439,0.5));
#39165=DIRECTION('',(0.,-0.866025403784439,0.5));
#39166=DIRECTION('',(-1.,0.,0.));
#39167=DIRECTION('',(0.,-0.866025403784439,0.5));
#39168=DIRECTION('center_axis',(0.,0.5,-0.866025403784439));
#39169=DIRECTION('ref_axis',(0.,-0.866025403784439,-0.5));
#39170=DIRECTION('',(0.,-0.866025403784439,-0.5));
#39171=DIRECTION('',(-1.,0.,0.));
#39172=DIRECTION('',(0.,-0.866025403784439,-0.5));
#39173=DIRECTION('center_axis',(0.,1.,-3.84592537276713E-16));
#39174=DIRECTION('ref_axis',(0.,-3.84592537276713E-16,-1.));
#39175=DIRECTION('',(0.,-3.84592537276713E-16,-1.));
#39176=DIRECTION('',(0.,-3.84592537276713E-16,-1.));
#39177=DIRECTION('center_axis',(-1.,0.,0.));
#39178=DIRECTION('ref_axis',(0.,0.,1.));
#39179=DIRECTION('center_axis',(-1.,0.,0.));
#39180=DIRECTION('ref_axis',(0.,0.,1.));
#39181=DIRECTION('center_axis',(1.,0.,0.));
#39182=DIRECTION('ref_axis',(0.,0.,-1.));
#39183=DIRECTION('center_axis',(1.,0.,0.));
#39184=DIRECTION('ref_axis',(0.,1.,0.));
#39185=DIRECTION('',(-0.707106781186548,0.707106781186547,8.65956056235493E-17));
#39186=DIRECTION('center_axis',(1.,0.,0.));
#39187=DIRECTION('ref_axis',(0.,1.,0.));
#39188=DIRECTION('center_axis',(1.,0.,0.));
#39189=DIRECTION('ref_axis',(0.,0.,-1.));
#39190=DIRECTION('',(-1.,0.,0.));
#39191=DIRECTION('',(-1.,0.,0.));
#39192=DIRECTION('center_axis',(-1.,0.,0.));
#39193=DIRECTION('ref_axis',(0.,1.,0.));
#39194=DIRECTION('center_axis',(1.,0.,0.));
#39195=DIRECTION('ref_axis',(0.,0.,-1.));
#39196=DIRECTION('',(-0.707106781186547,-0.707106781186548,-8.65956056235494E-17));
#39197=DIRECTION('center_axis',(1.,0.,0.));
#39198=DIRECTION('ref_axis',(0.,0.,-1.));
#55997=CARTESIAN_POINT('',(0.,0.,0.));
#55998=CARTESIAN_POINT('Origin',(-17.3,0.,0.));
#55999=CARTESIAN_POINT('',(-34.4758449541571,-1.46537014458274,0.000897397219902993));
#56000=CARTESIAN_POINT('',(-34.5471550458428,-1.46483013109474,0.00162234200369738));
#56001=CARTESIAN_POINT('',(-17.3,-1.4635,-1.79227059055215E-16));
#56002=CARTESIAN_POINT('',(-34.6365,0.634777570163803,1.32001124579653));
#56003=CARTESIAN_POINT('Ctrl Pts',(-34.4758449541571,-1.46537014458274,
0.000897397219902993));
#56004=CARTESIAN_POINT('Ctrl Pts',(-34.4783310796223,-1.46566838207244,
0.0464499273981202));
#56005=CARTESIAN_POINT('Ctrl Pts',(-34.4808172050875,-1.46372976632423,
0.0919749017138783));
#56006=CARTESIAN_POINT('Ctrl Pts',(-34.4833033305527,-1.4594716333831,0.137279627198249));
#56007=CARTESIAN_POINT('Ctrl Pts',(-34.5098178729584,-1.41405862104037,
0.620454785430562));
#56008=CARTESIAN_POINT('Ctrl Pts',(-34.5363324153641,-1.10481827728657,
1.07857832446841));
#56009=CARTESIAN_POINT('Ctrl Pts',(-34.5628469577697,-0.673702411121009,
1.30178944989929));
#56010=CARTESIAN_POINT('Ctrl Pts',(-34.5873979718465,-0.274512731095817,
1.50847072686393));
#56011=CARTESIAN_POINT('Ctrl Pts',(-34.6119489859233,0.22916992251388,1.51374407429557));
#56012=CARTESIAN_POINT('Ctrl Pts',(-34.6365,0.635548045752396,1.32098221395621));
#56013=CARTESIAN_POINT('',(-34.6365,-0.63400709457496,1.31904027763697));
#56014=CARTESIAN_POINT('Origin',(-34.6365,0.,0.));
#56015=CARTESIAN_POINT('Ctrl Pts',(-34.6365,-0.63400709457496,1.31904027763697));
#56016=CARTESIAN_POINT('Ctrl Pts',(-34.6099854575943,-1.07350019101018,
1.10779446059807));
#56017=CARTESIAN_POINT('Ctrl Pts',(-34.5834709151886,-1.39526457424107,
0.66143532399529));
#56018=CARTESIAN_POINT('Ctrl Pts',(-34.5569563727829,-1.45465419899784,
0.18052244014254));
#56019=CARTESIAN_POINT('Ctrl Pts',(-34.5536892638029,-1.46197215958701,
0.121264589208655));
#56020=CARTESIAN_POINT('Ctrl Pts',(-34.5504221548229,-1.46530647157864,
0.0614821070656839));
#56021=CARTESIAN_POINT('Ctrl Pts',(-34.5471550458428,-1.46483013109474,
0.00162234200369738));
#56022=CARTESIAN_POINT('Origin',(-17.3,0.,0.));
#56023=CARTESIAN_POINT('',(-33.9758449541571,-1.4616392812288,0.000897080157781296));
#56024=CARTESIAN_POINT('',(-34.0471550458428,-1.461397981138,0.000713649214188957));
#56025=CARTESIAN_POINT('',(-17.3,-1.4635,-1.79227059055215E-16));
#56026=CARTESIAN_POINT('Ctrl Pts',(-33.9758449541571,-1.4616392812288,0.000897080157781296));
#56027=CARTESIAN_POINT('Ctrl Pts',(-33.9859104918548,-1.46267180320561,
0.186551578039893));
#56028=CARTESIAN_POINT('Ctrl Pts',(-33.9959760295526,-1.42989485312375,
0.371854708030454));
#56029=CARTESIAN_POINT('Ctrl Pts',(-34.0060415672503,-1.36164030601831,
0.543008955714544));
#56030=CARTESIAN_POINT('Ctrl Pts',(-34.032556109656,-1.18184483577603,0.993861825616221));
#56031=CARTESIAN_POINT('Ctrl Pts',(-34.0590706520617,-0.755871778961322,
1.3465361831291));
#56032=CARTESIAN_POINT('Ctrl Pts',(-34.0855851944674,-0.279385519054958,
1.43904678126577));
#56033=CARTESIAN_POINT('Ctrl Pts',(-34.1120997368731,0.197100740851406,
1.53155737940244));
#56034=CARTESIAN_POINT('Ctrl Pts',(-34.1386142792788,0.724100203849429,
1.3639042181629));
#56035=CARTESIAN_POINT('Ctrl Pts',(-34.1651288216845,1.05953716804195,1.01307402656519));
#56036=CARTESIAN_POINT('Ctrl Pts',(-34.1916433640901,1.39497413223448,0.662243834967482));
#56037=CARTESIAN_POINT('Ctrl Pts',(-34.2181579064958,1.53884859762151,0.128236613011602));
#56038=CARTESIAN_POINT('Ctrl Pts',(-34.2446724489015,1.42508057453266,-0.34361308056253));
#56039=CARTESIAN_POINT('Ctrl Pts',(-34.2711869913072,1.31131255144381,-0.815462774136661));
#56040=CARTESIAN_POINT('Ctrl Pts',(-34.2977015337129,0.939902039879098,
-1.22515493932904));
#56041=CARTESIAN_POINT('Ctrl Pts',(-34.3242160761186,0.481438861446158,
-1.38458468548627));
#56042=CARTESIAN_POINT('Ctrl Pts',(-34.3507306185242,0.0229756830132183,
-1.54401443164349));
#56043=CARTESIAN_POINT('Ctrl Pts',(-34.3772451609299,-0.522540162287944,
-1.45318175876555));
#56044=CARTESIAN_POINT('Ctrl Pts',(-34.4037597033356,-0.904505244472703,
-1.1536520336132));
#56045=CARTESIAN_POINT('Ctrl Pts',(-34.4277881202761,-1.25065552347862,
-0.88220759335438));
#56046=CARTESIAN_POINT('Ctrl Pts',(-34.4518165372166,-1.46248767752697,
-0.439368069321345));
#56047=CARTESIAN_POINT('Ctrl Pts',(-34.4758449541571,-1.46537014458274,
0.000897397219902993));
#56048=CARTESIAN_POINT('Ctrl Pts',(-34.5471550458428,-1.46483013109474,
0.00162234200369738));
#56049=CARTESIAN_POINT('Ctrl Pts',(-34.5239076124172,-1.46144068380198,
-0.424315669752557));
#56050=CARTESIAN_POINT('Ctrl Pts',(-34.5006601789915,-1.26511130217635,
-0.854166649541362));
#56051=CARTESIAN_POINT('Ctrl Pts',(-34.4774127455659,-0.938168170832327,
-1.12676217466842));
#56052=CARTESIAN_POINT('Ctrl Pts',(-34.4508982031602,-0.565277651627364,
-1.4376672745239));
#56053=CARTESIAN_POINT('Ctrl Pts',(-34.4243836607545,-0.0224817469347706,
-1.54401084313214));
#56054=CARTESIAN_POINT('Ctrl Pts',(-34.3978691183488,0.440521457961799,
-1.39802412172701));
#56055=CARTESIAN_POINT('Ctrl Pts',(-34.3713545759431,0.903524662858368,
-1.25203740032188));
#56056=CARTESIAN_POINT('Ctrl Pts',(-34.3448400335375,1.28673516795891,-0.853720388903368));
#56057=CARTESIAN_POINT('Ctrl Pts',(-34.3183254911318,1.41432065046245,-0.385486997806588));
#56058=CARTESIAN_POINT('Ctrl Pts',(-34.2918109487261,1.54190613296599,0.0827463932901925));
#56059=CARTESIAN_POINT('Ctrl Pts',(-34.2652964063204,1.41386659287251,0.620896164065243));
#56060=CARTESIAN_POINT('Ctrl Pts',(-34.2387818639147,1.08891519320202,0.981481756368469));
#56061=CARTESIAN_POINT('Ctrl Pts',(-34.212267321509,0.763963793531522,1.34206734867169));
#56062=CARTESIAN_POINT('Ctrl Pts',(-34.1857527791033,0.242100534284002,
1.5250887625031));
#56063=CARTESIAN_POINT('Ctrl Pts',(-34.1592382366976,-0.236909082514337,
1.44662785965613));
#56064=CARTESIAN_POINT('Ctrl Pts',(-34.132723694292,-0.715918699312675,
1.36816695680916));
#56065=CARTESIAN_POINT('Ctrl Pts',(-34.1062091518863,-1.15207467366184,
1.02822373728382));
#56066=CARTESIAN_POINT('Ctrl Pts',(-34.0796946094806,-1.34506104653608,
0.582868204388268));
#56067=CARTESIAN_POINT('Ctrl Pts',(-34.068848088268,-1.42400756407709,0.400682965782681));
#56068=CARTESIAN_POINT('Ctrl Pts',(-34.0580015670554,-1.46226087156527,
0.200857506589857));
#56069=CARTESIAN_POINT('Ctrl Pts',(-34.0471550458428,-1.461397981138,0.000713649214188957));
#56070=CARTESIAN_POINT('Origin',(-17.3,0.,0.));
#56071=CARTESIAN_POINT('',(-33.4758449541571,-1.46210997131077,-0.00113575995333209));
#56072=CARTESIAN_POINT('',(-33.5471550458428,-1.46247549057344,-0.00124878738715978));
#56073=CARTESIAN_POINT('',(-17.3,-1.4635,-1.79227059055215E-16));
#56074=CARTESIAN_POINT('Ctrl Pts',(-33.4758449541571,-1.46210997131077,
-0.00113575995333209));
#56075=CARTESIAN_POINT('Ctrl Pts',(-33.4934899040874,-1.45976617832587,
0.324054087244827));
#56076=CARTESIAN_POINT('Ctrl Pts',(-33.5111348540177,-1.35274610243324,
0.650643945905838));
#56077=CARTESIAN_POINT('Ctrl Pts',(-33.528779803948,-1.15337718085729,0.904788922614451));
#56078=CARTESIAN_POINT('Ctrl Pts',(-33.5552943463537,-0.853791421397257,
1.28668503389574));
#56079=CARTESIAN_POINT('Ctrl Pts',(-33.5818088887594,-0.345680300135375,
1.50499929303762));
#56080=CARTESIAN_POINT('Ctrl Pts',(-33.608323431165,0.137560532310046,1.45945151745205));
#56081=CARTESIAN_POINT('Ctrl Pts',(-33.6348379735707,0.620801364755467,
1.41390374186649));
#56082=CARTESIAN_POINT('Ctrl Pts',(-33.6613525159764,1.07917190838443,1.10449393155347));
#56083=CARTESIAN_POINT('Ctrl Pts',(-33.6878670583821,1.30212421740846,0.673345854018389));
#56084=CARTESIAN_POINT('Ctrl Pts',(-33.7143816007878,1.5250765264325,0.242197776483304));
#56085=CARTESIAN_POINT('Ctrl Pts',(-33.7408961431935,1.51261060085162,-0.310688568273853));
#56086=CARTESIAN_POINT('Ctrl Pts',(-33.7674106855992,1.27045269311141,-0.731349505481218));
#56087=CARTESIAN_POINT('Ctrl Pts',(-33.7939252280048,1.0282947853712,-1.15201044268858));
#56088=CARTESIAN_POINT('Ctrl Pts',(-33.8204397704105,0.556444895471674,
-1.44044597234615));
#56089=CARTESIAN_POINT('Ctrl Pts',(-33.8469543128162,0.071642192326496,
-1.46416793330233));
#56090=CARTESIAN_POINT('Ctrl Pts',(-33.8734688552219,-0.413160510818682,
-1.48788989425851));
#56091=CARTESIAN_POINT('Ctrl Pts',(-33.8999833976276,-0.91091602720951,
-1.24689828651329));
#56092=CARTESIAN_POINT('Ctrl Pts',(-33.9264979400333,-1.19298484356999,
-0.851886791495445));
#56093=CARTESIAN_POINT('Ctrl Pts',(-33.9429469447412,-1.36797376916733,
-0.606830857969515));
#56094=CARTESIAN_POINT('Ctrl Pts',(-33.9593959494492,-1.45995194376432,
-0.302497711200068));
#56095=CARTESIAN_POINT('Ctrl Pts',(-33.9758449541571,-1.4616392812288,0.000897080157781296));
#56096=CARTESIAN_POINT('Ctrl Pts',(-34.0471550458428,-1.461397981138,0.000713649214188957));
#56097=CARTESIAN_POINT('Ctrl Pts',(-34.0314870246497,-1.46015151831025,
-0.288398236298732));
#56098=CARTESIAN_POINT('Ctrl Pts',(-34.0158190034566,-1.37728366376588,
-0.578174503939485));
#56099=CARTESIAN_POINT('Ctrl Pts',(-34.0001509822635,-1.21754783627738,
-0.81640383976837));
#56100=CARTESIAN_POINT('Ctrl Pts',(-33.9736364398579,-0.947231481745092,
-1.2195525047637));
#56101=CARTESIAN_POINT('Ctrl Pts',(-33.9471218974522,-0.456782001281173,
-1.47508198848859));
#56102=CARTESIAN_POINT('Ctrl Pts',(-33.9206073550465,0.0285098714968319,
-1.46563947024646));
#56103=CARTESIAN_POINT('Ctrl Pts',(-33.8940928126408,0.513801744274836,
-1.45619695200433));
#56104=CARTESIAN_POINT('Ctrl Pts',(-33.8675782702351,0.993936009366925,
-1.18178243179517));
#56105=CARTESIAN_POINT('Ctrl Pts',(-33.8410637278294,1.24837193381408,-0.76843381664129));
#56106=CARTESIAN_POINT('Ctrl Pts',(-33.8145491854237,1.50280785826124,-0.355085201487411));
#56107=CARTESIAN_POINT('Ctrl Pts',(-33.7880346430181,1.53154544206345,0.197197508611189));
#56108=CARTESIAN_POINT('Ctrl Pts',(-33.7615201006124,1.32138222003508,0.634722724967845));
#56109=CARTESIAN_POINT('Ctrl Pts',(-33.7350055582067,1.1112189980067,1.0722479413245));
#56110=CARTESIAN_POINT('Ctrl Pts',(-33.708491015801,0.662154970147739,1.39501566393922));
#56111=CARTESIAN_POINT('Ctrl Pts',(-33.6819764733953,0.180464277792477,
1.4547690367785));
#56112=CARTESIAN_POINT('Ctrl Pts',(-33.6554619309896,-0.301226414562783,
1.51452240961778));
#56113=CARTESIAN_POINT('Ctrl Pts',(-33.6289473885839,-0.815543771414339,
1.31126143268162));
#56114=CARTESIAN_POINT('Ctrl Pts',(-33.6024328461783,-1.12624192354582,
0.938350275931457));
#56115=CARTESIAN_POINT('Ctrl Pts',(-33.5840069127331,-1.34215752884309,
0.679200559142212));
#56116=CARTESIAN_POINT('Ctrl Pts',(-33.565580979288,-1.45973783110767,0.33812044750393));
#56117=CARTESIAN_POINT('Ctrl Pts',(-33.5471550458428,-1.46247549057344,
-0.00124878738715978));
#56118=CARTESIAN_POINT('Origin',(-17.3,0.,0.));
#56119=CARTESIAN_POINT('',(-32.9758449541571,-1.46576386267191,-0.000435669595795773));
#56120=CARTESIAN_POINT('',(-33.0471550458428,-1.46589447233764,-0.0001750908953165));
#56121=CARTESIAN_POINT('',(-17.3,-1.4635,-1.79227059055215E-16));
#56122=CARTESIAN_POINT('Ctrl Pts',(-32.9758449541571,-1.46576386267191,
-0.000435669595795773));
#56123=CARTESIAN_POINT('Ctrl Pts',(-33.0010693163199,-1.46395560202229,
0.461460515586922));
#56124=CARTESIAN_POINT('Ctrl Pts',(-33.0262936784828,-1.22744187685039,
0.924951081530073));
#56125=CARTESIAN_POINT('Ctrl Pts',(-33.0515180406456,-0.851584434241105,
1.19319982047713));
#56126=CARTESIAN_POINT('Ctrl Pts',(-33.0780325830513,-0.456502567107242,
1.47516899449099));
#56127=CARTESIAN_POINT('Ctrl Pts',(-33.104547125457,0.0925419150148735,
1.54141303362098));
#56128=CARTESIAN_POINT('Ctrl Pts',(-33.1310616678627,0.543350994710775,
1.36150341542638));
#56129=CARTESIAN_POINT('Ctrl Pts',(-33.1575762102684,0.994160074406676,
1.18159379723179));
#56130=CARTESIAN_POINT('Ctrl Pts',(-33.1840907526741,1.34673375167636,0.755530521712624));
#56131=CARTESIAN_POINT('Ctrl Pts',(-33.2106052950797,1.43912087941628,0.279021425816014));
#56132=CARTESIAN_POINT('Ctrl Pts',(-33.2371198374854,1.53150800715619,-0.197487670080597));
#56133=CARTESIAN_POINT('Ctrl Pts',(-33.2636343798911,1.36370858536632,-0.724442586354652));
#56134=CARTESIAN_POINT('Ctrl Pts',(-33.2901489222968,1.01279958114557,-1.05979190284854));
#56135=CARTESIAN_POINT('Ctrl Pts',(-33.3166634647025,0.661890576924812,
-1.39514121934244));
#56136=CARTESIAN_POINT('Ctrl Pts',(-33.3431780071082,0.127871990273167,
-1.53888493605617));
#56137=CARTESIAN_POINT('Ctrl Pts',(-33.3696925495139,-0.34396015959519,
-1.42499587153609));
#56138=CARTESIAN_POINT('Ctrl Pts',(-33.3962070919196,-0.815792309463548,
-1.31110680701601));
#56139=CARTESIAN_POINT('Ctrl Pts',(-33.4227216343252,-1.22543802254862,
-0.939584961262129));
#56140=CARTESIAN_POINT('Ctrl Pts',(-33.4492361767309,-1.38473068026206,
-0.481085056674836));
#56141=CARTESIAN_POINT('Ctrl Pts',(-33.4581057692063,-1.43801694621464,
-0.327708572122606));
#56142=CARTESIAN_POINT('Ctrl Pts',(-33.4669753616817,-1.46328812646025,
-0.164599041695517));
#56143=CARTESIAN_POINT('Ctrl Pts',(-33.4758449541571,-1.46210997131077,
-0.00113575995333209));
#56144=CARTESIAN_POINT('Ctrl Pts',(-33.5471550458428,-1.46247549057344,
-0.00124878738715978));
#56145=CARTESIAN_POINT('Ctrl Pts',(-33.5390664368823,-1.46367726724064,
-0.150224959609039));
#56146=CARTESIAN_POINT('Ctrl Pts',(-33.5309778279217,-1.44274851149922,
-0.298871440590991));
#56147=CARTESIAN_POINT('Ctrl Pts',(-33.5228892189612,-1.39829282246071,
-0.44011278706805));
#56148=CARTESIAN_POINT('Ctrl Pts',(-33.4963746765555,-1.25256662183269,
-0.903103356753219));
#56149=CARTESIAN_POINT('Ctrl Pts',(-33.4698601341498,-0.854035273165233,
-1.28652315955938));
#56150=CARTESIAN_POINT('Ctrl Pts',(-33.4433455917441,-0.385760277856051,
-1.41425266684387));
#56151=CARTESIAN_POINT('Ctrl Pts',(-33.4168310493384,0.0825147174531302,
-1.54198217412836));
#56152=CARTESIAN_POINT('Ctrl Pts',(-33.3903165069327,0.620533359404036,
-1.41402138589117));
#56153=CARTESIAN_POINT('Ctrl Pts',(-33.3638019645271,0.981162324775984,
-1.08914754473287));
#56154=CARTESIAN_POINT('Ctrl Pts',(-33.3372874221214,1.34179129014793,-0.764273703574562));
#56155=CARTESIAN_POINT('Ctrl Pts',(-33.3107728797157,1.52503057894092,-0.242486809495135));
#56156=CARTESIAN_POINT('Ctrl Pts',(-33.28425833731,1.44671103502957,0.236535484996721));
#56157=CARTESIAN_POINT('Ctrl Pts',(-33.2577437949043,1.36839149111822,0.715557779488577));
#56158=CARTESIAN_POINT('Ctrl Pts',(-33.2312292524986,1.02851311450254,1.15181547439287));
#56159=CARTESIAN_POINT('Ctrl Pts',(-33.2047147100929,0.583195617041653,
1.34491808800433));
#56160=CARTESIAN_POINT('Ctrl Pts',(-33.1782001676873,0.137878119580767,
1.5380207016158));
#56161=CARTESIAN_POINT('Ctrl Pts',(-33.1516856252816,-0.412878498725314,
1.48796823393444));
#56162=CARTESIAN_POINT('Ctrl Pts',(-33.1251710828759,-0.816089779884158,
1.21775174235156));
#56163=CARTESIAN_POINT('Ctrl Pts',(-33.0991657371982,-1.21155761739175,
0.95272460502037));
#56164=CARTESIAN_POINT('Ctrl Pts',(-33.0731603915205,-1.46509275032866,
0.475908495121908));
#56165=CARTESIAN_POINT('Ctrl Pts',(-33.0471550458428,-1.46589447233764,
-0.0001750908953165));
#56166=CARTESIAN_POINT('Origin',(-17.3,0.,0.));
#56167=CARTESIAN_POINT('',(-32.4758449541571,-1.46343401324079,0.00135214320468362));
#56168=CARTESIAN_POINT('',(-32.5471550458428,-1.46300356173616,0.00133575934057721));
#56169=CARTESIAN_POINT('',(-17.3,-1.4635,-1.79227059055215E-16));
#56170=CARTESIAN_POINT('Ctrl Pts',(-32.4758449541571,-1.46343401324079,
0.00135214320468362));
#56171=CARTESIAN_POINT('Ctrl Pts',(-32.4821341861468,-1.46449987346685,
0.116994707761757));
#56172=CARTESIAN_POINT('Ctrl Pts',(-32.4884234181365,-1.45195163790634,
0.232408645151303));
#56173=CARTESIAN_POINT('Ctrl Pts',(-32.4947126501262,-1.42490895575888,
0.344320092666205));
#56174=CARTESIAN_POINT('Ctrl Pts',(-32.5212271925319,-1.31090070423688,
0.816123458430666));
#56175=CARTESIAN_POINT('Ctrl Pts',(-32.5477417349376,-0.939275356078788,
1.22567530827207));
#56176=CARTESIAN_POINT('Ctrl Pts',(-32.5742562773433,-0.480735248577563,
1.38485215067918));
#56177=CARTESIAN_POINT('Ctrl Pts',(-32.6007708197489,-0.0221951410763392,
1.54402899308628));
#56178=CARTESIAN_POINT('Ctrl Pts',(-32.6272853621546,0.523259725768014,
1.45283082805909));
#56179=CARTESIAN_POINT('Ctrl Pts',(-32.6537999045603,0.905080187032809,
1.15314860853539));
#56180=CARTESIAN_POINT('Ctrl Pts',(-32.680314446966,1.2869006482976,0.853466389011679));
#56181=CARTESIAN_POINT('Ctrl Pts',(-32.7068289893717,1.50508670398284,0.345300114991455));
#56182=CARTESIAN_POINT('Ctrl Pts',(-32.7333435317774,1.45941680067057,-0.13792918600512));
#56183=CARTESIAN_POINT('Ctrl Pts',(-32.7598580741831,1.41374689735831,-0.621158487001693));
#56184=CARTESIAN_POINT('Ctrl Pts',(-32.7863726165887,1.10422103504854,-1.07945081497461));
#56185=CARTESIAN_POINT('Ctrl Pts',(-32.8128871589944,0.673016781644122,
-1.30229423339842));
#56186=CARTESIAN_POINT('Ctrl Pts',(-32.8394017014001,0.2418125282397,-1.52513765182224));
#56187=CARTESIAN_POINT('Ctrl Pts',(-32.8659162438058,-0.311070116259374,
-1.51253216069693));
#56188=CARTESIAN_POINT('Ctrl Pts',(-32.8924307862115,-0.731670112660202,
-1.27026796542771));
#56189=CARTESIAN_POINT('Ctrl Pts',(-32.9189453286172,-1.15227010906103,
-1.02800377015849));
#56190=CARTESIAN_POINT('Ctrl Pts',(-32.9454598710229,-1.44058745736361,
-0.55608087074537));
#56191=CARTESIAN_POINT('Ctrl Pts',(-32.9719744134285,-1.46418650544209,
-0.071272266589932));
#56192=CARTESIAN_POINT('Ctrl Pts',(-32.9732645936714,-1.46533481964322,
-0.0476817978927391));
#56193=CARTESIAN_POINT('Ctrl Pts',(-32.9745547739142,-1.465856351915,-0.0240608193030587));
#56194=CARTESIAN_POINT('Ctrl Pts',(-32.9758449541571,-1.46576386267191,
-0.000435669595795773));
#56195=CARTESIAN_POINT('Ctrl Pts',(-33.0471550458428,-1.46589447233764,
-0.0001750908953165));
#56196=CARTESIAN_POINT('Ctrl Pts',(-33.0466458491148,-1.46591017042636,
-0.00949702828685));
#56197=CARTESIAN_POINT('Ctrl Pts',(-33.0461366523868,-1.46582897190017,
-0.0188186848327125));
#56198=CARTESIAN_POINT('Ctrl Pts',(-33.0456274556588,-1.46565004497337,
-0.0281384651248314));
#56199=CARTESIAN_POINT('Ctrl Pts',(-33.0191129132531,-1.45633308489213,
-0.513431665533941));
#56200=CARTESIAN_POINT('Ctrl Pts',(-32.9925983708474,-1.18203322071805,
-0.993637550867758));
#56201=CARTESIAN_POINT('Ctrl Pts',(-32.9660838284418,-0.768747318591459,
-1.24817842464081));
#56202=CARTESIAN_POINT('Ctrl Pts',(-32.9395692860361,-0.35546141646487,
-1.50271929841385));
#56203=CARTESIAN_POINT('Ctrl Pts',(-32.9130547436304,0.196810523614232,
-1.53159516062613));
#56204=CARTESIAN_POINT('Ctrl Pts',(-32.8865402012247,0.634387985068444,
-1.32154217130706));
#56205=CARTESIAN_POINT('Ctrl Pts',(-32.860025658819,1.07196544652266,-1.11148918198798));
#56206=CARTESIAN_POINT('Ctrl Pts',(-32.8335111164133,1.39484842935199,-0.662507341137544));
#56207=CARTESIAN_POINT('Ctrl Pts',(-32.8069965740076,1.45472390680499,-0.180831909756413));
#56208=CARTESIAN_POINT('Ctrl Pts',(-32.780482031602,1.51459938425799,0.300843521624713));
#56209=CARTESIAN_POINT('Ctrl Pts',(-32.7539674891963,1.31146735633467,0.815212543536533));
#56210=CARTESIAN_POINT('Ctrl Pts',(-32.7274529467906,0.938634461852072,
1.12600496032996));
#56211=CARTESIAN_POINT('Ctrl Pts',(-32.7009384043849,0.565801567369472,
1.4367973771234));
#56212=CARTESIAN_POINT('Ctrl Pts',(-32.6744238619792,0.0232678063275967,
1.54401318879844));
#56213=CARTESIAN_POINT('Ctrl Pts',(-32.6479093195735,-0.439759436949033,
1.39840389810825));
#56214=CARTESIAN_POINT('Ctrl Pts',(-32.6213947771678,-0.902786680225661,
1.25279460741805));
#56215=CARTESIAN_POINT('Ctrl Pts',(-32.5948802347622,-1.28630740573704,
0.854360214362621));
#56216=CARTESIAN_POINT('Ctrl Pts',(-32.5683656923565,-1.41415525502841,
0.38611751970031));
#56217=CARTESIAN_POINT('Ctrl Pts',(-32.5612954768519,-1.44824642780646,
0.261258613631341));
#56218=CARTESIAN_POINT('Ctrl Pts',(-32.5542252613474,-1.46415811092022,
0.131436023825928));
#56219=CARTESIAN_POINT('Ctrl Pts',(-32.5471550458428,-1.46300356173616,
0.00133575934057721));
#56220=CARTESIAN_POINT('Origin',(-17.3,0.,0.));
#56221=CARTESIAN_POINT('',(-31.9758449541571,-1.4610973901521,-0.000186288173925353));
#56222=CARTESIAN_POINT('',(-32.0471550458428,-1.46118615381657,-0.000418794261562428));
#56223=CARTESIAN_POINT('',(-17.3,-1.4635,-1.79227059055215E-16));
#56224=CARTESIAN_POINT('Ctrl Pts',(-31.9758449541571,-1.4610973901521,-0.000186288173925353));
#56225=CARTESIAN_POINT('Ctrl Pts',(-31.9897135983793,-1.46080759427907,
0.25585153086225));
#56226=CARTESIAN_POINT('Ctrl Pts',(-32.0035822426016,-1.39685690896212,
0.512024759540195));
#56227=CARTESIAN_POINT('Ctrl Pts',(-32.0174508868239,-1.27008311131556,
0.731990948556328));
#56228=CARTESIAN_POINT('Ctrl Pts',(-32.0439654292295,-1.02771268348116,
1.15252973756993));
#56229=CARTESIAN_POINT('Ctrl Pts',(-32.0704799716352,-0.555716971662109,
1.44072787270177));
#56230=CARTESIAN_POINT('Ctrl Pts',(-32.0969945140409,-0.0709024224430543,
1.4642044614433));
#56231=CARTESIAN_POINT('Ctrl Pts',(-32.1235090564466,0.413912126776,1.48768105018482));
#56232=CARTESIAN_POINT('Ctrl Pts',(-32.1500235988523,0.91154551339507,1.24643609253604));
#56233=CARTESIAN_POINT('Ctrl Pts',(-32.176538141258,1.19341488474662,0.851283014796641));
#56234=CARTESIAN_POINT('Ctrl Pts',(-32.2030526836637,1.47528425609817,0.45612993705724));
#56235=CARTESIAN_POINT('Ctrl Pts',(-32.2295672260693,1.54138961218219,-0.0929312607727704));
#56236=CARTESIAN_POINT('Ctrl Pts',(-32.256081768475,1.3613661276533,-0.543694882167351));
#56237=CARTESIAN_POINT('Ctrl Pts',(-32.2825963108807,1.18134264312441,-0.994458503561922));
#56238=CARTESIAN_POINT('Ctrl Pts',(-32.3091108532864,0.755190317982634,
-1.34692454852107));
#56239=CARTESIAN_POINT('Ctrl Pts',(-32.3356253956921,0.278657903762824,
-1.43919131149949));
#56240=CARTESIAN_POINT('Ctrl Pts',(-32.3621399380978,-0.19787451045699,
-1.53145807447791));
#56241=CARTESIAN_POINT('Ctrl Pts',(-32.3886544805034,-0.724787013754835,
-1.3635255554756));
#56242=CARTESIAN_POINT('Ctrl Pts',(-32.4151690229091,-1.06004768796081,
-1.01253185513069));
#56243=CARTESIAN_POINT('Ctrl Pts',(-32.4353943333251,-1.31578475112933,
-0.744793629257785));
#56244=CARTESIAN_POINT('Ctrl Pts',(-32.4556196437411,-1.46000635244413,
-0.37053853745336));
#56245=CARTESIAN_POINT('Ctrl Pts',(-32.4758449541571,-1.46343401324079,
0.00135214320468362));
#56246=CARTESIAN_POINT('Ctrl Pts',(-32.5471550458428,-1.46300356173616,
0.00133575934057721));
#56247=CARTESIAN_POINT('Ctrl Pts',(-32.5277107189417,-1.45982834992771,
-0.356462679893697));
#56248=CARTESIAN_POINT('Ctrl Pts',(-32.5082663920405,-1.32757336974612,
-0.716361300512106));
#56249=CARTESIAN_POINT('Ctrl Pts',(-32.4888220651394,-1.0893953049412,-0.980887197291753));
#56250=CARTESIAN_POINT('Ctrl Pts',(-32.4623075227337,-0.764612532491269,
-1.34159822335231));
#56251=CARTESIAN_POINT('Ctrl Pts',(-32.4357929803281,-0.24287201452005,
-1.52496927920423));
#56252=CARTESIAN_POINT('Ctrl Pts',(-32.4092784379224,0.236170029881672,
-1.44677072867951));
#56253=CARTESIAN_POINT('Ctrl Pts',(-32.3827638955167,0.715212074283389,
-1.36857217815479));
#56254=CARTESIAN_POINT('Ctrl Pts',(-32.356249353111,1.15155564511561,-1.02880402125342));
#56255=CARTESIAN_POINT('Ctrl Pts',(-32.3297348107053,1.34477074540355,-0.583535317384259));
#56256=CARTESIAN_POINT('Ctrl Pts',(-32.3032202682996,1.53798584569149,-0.138266613515089));
#56257=CARTESIAN_POINT('Ctrl Pts',(-32.2767057258939,1.48807247543514,0.412502637321881));
#56258=CARTESIAN_POINT('Ctrl Pts',(-32.2501911834882,1.21795783540472,0.81578216178961));
#56259=CARTESIAN_POINT('Ctrl Pts',(-32.2236766410825,0.947843195374297,
1.21906168625734));
#56260=CARTESIAN_POINT('Ctrl Pts',(-32.1971620986768,0.457527285569812,
1.47485148435582));
#56261=CARTESIAN_POINT('Ctrl Pts',(-32.1706475562712,-0.0277682501593372,
1.46565710472151));
#56262=CARTESIAN_POINT('Ctrl Pts',(-32.1441330138655,-0.513063785888485,
1.4564627250872));
#56263=CARTESIAN_POINT('Ctrl Pts',(-32.1176184714598,-0.993338947542297,
1.1822841677201));
#56264=CARTESIAN_POINT('Ctrl Pts',(-32.0911039290541,-1.24798420716327,
0.76906257417729));
#56265=CARTESIAN_POINT('Ctrl Pts',(-32.076454301317,-1.38867900782723,0.54075229728431));
#56266=CARTESIAN_POINT('Ctrl Pts',(-32.0618046735799,-1.46049564483494,
0.269996276654853));
#56267=CARTESIAN_POINT('Ctrl Pts',(-32.0471550458428,-1.46118615381657,
-0.000418794261562428));
#56268=CARTESIAN_POINT('Origin',(-17.3,0.,0.));
#56269=CARTESIAN_POINT('',(-31.4758449541571,-1.46411995320351,-0.00128603361858132));
#56270=CARTESIAN_POINT('',(-31.5471550458428,-1.46454451199446,-0.00118531342847866));
#56271=CARTESIAN_POINT('',(-17.3,-1.4635,-1.79227059055215E-16));
#56272=CARTESIAN_POINT('Ctrl Pts',(-31.4758449541571,-1.46411995320351,
-0.00128603361858132));
#56273=CARTESIAN_POINT('Ctrl Pts',(-31.4972930106119,-1.4604966735953,0.392614030616494));
#56274=CARTESIAN_POINT('Ctrl Pts',(-31.5187410670667,-1.2962572267619,0.789177174870507));
#56275=CARTESIAN_POINT('Ctrl Pts',(-31.5401891235215,-1.01226406354304,
1.06030341132948));
#56276=CARTESIAN_POINT('Ctrl Pts',(-31.5667036659272,-0.661185690313245,
1.3954754167294));
#56277=CARTESIAN_POINT('Ctrl Pts',(-31.5932182083329,-0.127094551235654,
1.53894935940639));
#56278=CARTESIAN_POINT('Ctrl Pts',(-31.6197327507385,0.344680001926412,
1.42482193788896));
#56279=CARTESIAN_POINT('Ctrl Pts',(-31.6462472931442,0.816454555088478,
1.31069451637152));
#56280=CARTESIAN_POINT('Ctrl Pts',(-31.6727618355499,1.22591252233502,0.938965730659652));
#56281=CARTESIAN_POINT('Ctrl Pts',(-31.6992763779556,1.38497353623587,0.480385431027943));
#56282=CARTESIAN_POINT('Ctrl Pts',(-31.7257909203613,1.54403455013671,0.0218051313962338));
#56283=CARTESIAN_POINT('Ctrl Pts',(-31.752305462767,1.45269861069187,-0.523626682155316));
#56284=CARTESIAN_POINT('Ctrl Pts',(-31.7788200051727,1.15291995600268,-0.905371433980737));
#56285=CARTESIAN_POINT('Ctrl Pts',(-31.8053345475784,0.853141301313501,
-1.28711618580616));
#56286=CARTESIAN_POINT('Ctrl Pts',(-31.831849089984,0.344919931379984,-1.50517387590545));
#56287=CARTESIAN_POINT('Ctrl Pts',(-31.8583636323897,-0.138297818302765,
-1.45938191432897));
#56288=CARTESIAN_POINT('Ctrl Pts',(-31.8848781747954,-0.621515567985517,
-1.41358995275248));
#56289=CARTESIAN_POINT('Ctrl Pts',(-31.9113927172011,-1.0797296974175,-1.10394833950022));
#56290=CARTESIAN_POINT('Ctrl Pts',(-31.9379072596068,-1.30246419020861,
-0.672687811426406));
#56291=CARTESIAN_POINT('Ctrl Pts',(-31.9505531577902,-1.40869561878388,
-0.4670015640414));
#56292=CARTESIAN_POINT('Ctrl Pts',(-31.9631990559737,-1.46136163581632,
-0.233650218660073));
#56293=CARTESIAN_POINT('Ctrl Pts',(-31.9758449541571,-1.4610973901521,-0.000186288173925353));
#56294=CARTESIAN_POINT('Ctrl Pts',(-32.0471550458428,-1.46118615381657,
-0.000418794261562428));
#56295=CARTESIAN_POINT('Ctrl Pts',(-32.0352901311742,-1.46174540557996,
-0.219431304279028));
#56296=CARTESIAN_POINT('Ctrl Pts',(-32.0234252165056,-1.41564890171275,
-0.438220165590512));
#56297=CARTESIAN_POINT('Ctrl Pts',(-32.011560301837,-1.32170236948958,-0.634054154480603));
#56298=CARTESIAN_POINT('Ctrl Pts',(-31.9850457594313,-1.11175991460677,
-1.07168465987714));
#56299=CARTESIAN_POINT('Ctrl Pts',(-31.9585312170257,-0.662859647253007,
-1.3946810409517));
#56300=CARTESIAN_POINT('Ctrl Pts',(-31.93201667462,-0.181199355667255,-1.45467818359834));
#56301=CARTESIAN_POINT('Ctrl Pts',(-31.9055021322143,0.3004609359185,-1.51467532624497));
#56302=CARTESIAN_POINT('Ctrl Pts',(-31.8789875898086,0.814881251736254,
-1.31167323046369));
#56303=CARTESIAN_POINT('Ctrl Pts',(-31.8524730474029,1.1257678333244,-0.938918851542513));
#56304=CARTESIAN_POINT('Ctrl Pts',(-31.8259585049972,1.43665441491254,-0.566164472621339));
#56305=CARTESIAN_POINT('Ctrl Pts',(-31.7994439625915,1.54400726227108,-0.0236578105602783));
#56306=CARTESIAN_POINT('Ctrl Pts',(-31.7729294201859,1.39851493297882,0.439406197686252));
#56307=CARTESIAN_POINT('Ctrl Pts',(-31.7464148777802,1.25302260368656,0.902470205932789));
#56308=CARTESIAN_POINT('Ctrl Pts',(-31.7199003353745,0.854685097743509,
1.28609156036479));
#56309=CARTESIAN_POINT('Ctrl Pts',(-31.6933857929688,0.386474711384964,
1.41405767979603));
#56310=CARTESIAN_POINT('Ctrl Pts',(-31.6668712505631,-0.0817356749735745,
1.54202379922726));
#56311=CARTESIAN_POINT('Ctrl Pts',(-31.6403567081574,-0.619818941747609,
1.41433468365773));
#56312=CARTESIAN_POINT('Ctrl Pts',(-31.6138421657518,-0.980611993776293,
1.08964303420528));
#56313=CARTESIAN_POINT('Ctrl Pts',(-31.5916131257821,-1.28309065064331,
0.817430768835746));
#56314=CARTESIAN_POINT('Ctrl Pts',(-31.5693840858125,-1.46095786977572,
0.406751927520254));
#56315=CARTESIAN_POINT('Ctrl Pts',(-31.5471550458428,-1.46454451199446,
-0.00118531342847866));
#56316=CARTESIAN_POINT('Origin',(-17.3,0.,0.));
#56317=CARTESIAN_POINT('',(-30.9758449541571,-1.46537689164811,0.00080145734256621));
#56318=CARTESIAN_POINT('',(-31.0471550458428,-1.46504041338933,0.000995257504430862));
#56319=CARTESIAN_POINT('',(-17.3,-1.4635,-1.79227059055215E-16));
#56320=CARTESIAN_POINT('Ctrl Pts',(-30.9758449541571,-1.46537689164811,
0.00080145734256621));
#56321=CARTESIAN_POINT('Ctrl Pts',(-30.9783578804388,-1.46568003330817,
0.0468491384676566));
#56322=CARTESIAN_POINT('Ctrl Pts',(-30.9808708067204,-1.4636984540663,0.092870385363776));
#56323=CARTESIAN_POINT('Ctrl Pts',(-30.9833837330021,-1.45934693488595,
0.138666441710288));
#56324=CARTESIAN_POINT('Ctrl Pts',(-31.0098982754078,-1.41343291795737,
0.621872609306444));
#56325=CARTESIAN_POINT('Ctrl Pts',(-31.0364128178134,-1.10367557347831,
1.08000851120647));
#56326=CARTESIAN_POINT('Ctrl Pts',(-31.0629273602191,-0.672358798268734,
1.30263406404417));
#56327=CARTESIAN_POINT('Ctrl Pts',(-31.0894419026248,-0.241042023059151,
1.52525961688188));
#56328=CARTESIAN_POINT('Ctrl Pts',(-31.1159564450305,0.311834182880956,
1.51237482065725));
#56329=CARTESIAN_POINT('Ctrl Pts',(-31.1424709874362,0.732311737710161,
1.26989817592968));
#56330=CARTESIAN_POINT('Ctrl Pts',(-31.1689855298419,1.15278929253936,1.02742153120211));
#56331=CARTESIAN_POINT('Ctrl Pts',(-31.1955000722476,1.44086819625767,0.555353037971591));
#56332=CARTESIAN_POINT('Ctrl Pts',(-31.2220146146532,1.46422232409926,0.070532574226254));
#56333=CARTESIAN_POINT('Ctrl Pts',(-31.2485291570589,1.48757645194085,-0.414287889519083));
#56334=CARTESIAN_POINT('Ctrl Pts',(-31.2750436994646,1.24620580390573,-0.911860323779238));
#56335=CARTESIAN_POINT('Ctrl Pts',(-31.3015582418703,0.850981540896159,
-1.19362987373457));
#56336=CARTESIAN_POINT('Ctrl Pts',(-31.328072784276,0.455757277886592,-1.4753994236899));
#56337=CARTESIAN_POINT('Ctrl Pts',(-31.3545873266817,-0.0933206000974209,
-1.54136608934041));
#56338=CARTESIAN_POINT('Ctrl Pts',(-31.3811018690874,-0.544038734665332,
-1.36122875138654));
#56339=CARTESIAN_POINT('Ctrl Pts',(-31.407616411493,-0.994756869233242,
-1.18109141343267));
#56340=CARTESIAN_POINT('Ctrl Pts',(-31.4341309538987,-1.34711526038505,
-0.754850071874408));
#56341=CARTESIAN_POINT('Ctrl Pts',(-31.4606454963044,-1.43926165226995,
-0.278294367033853));
#56342=CARTESIAN_POINT('Ctrl Pts',(-31.4657119822553,-1.45686928783713,
-0.187232535890486));
#56343=CARTESIAN_POINT('Ctrl Pts',(-31.4707784682062,-1.46497584871413,
-0.0943335853026628));
#56344=CARTESIAN_POINT('Ctrl Pts',(-31.4758449541571,-1.46411995320351,
-0.00128603361858132));
#56345=CARTESIAN_POINT('Ctrl Pts',(-31.5471550458428,-1.46454451199446,
-0.00118531342847866));
#56346=CARTESIAN_POINT('Ctrl Pts',(-31.5428695434068,-1.46523597523294,
-0.0798309068605571));
#56347=CARTESIAN_POINT('Ctrl Pts',(-31.5385840409707,-1.45944988408569,
-0.15837460215921));
#56348=CARTESIAN_POINT('Ctrl Pts',(-31.5342985385347,-1.44683033710717,
-0.23580458001566));
#56349=CARTESIAN_POINT('Ctrl Pts',(-31.507783996129,-1.36875279112603,-0.714866361448761));
#56350=CARTESIAN_POINT('Ctrl Pts',(-31.4812694537233,-1.02909486188039,
-1.15129574097958));
#56351=CARTESIAN_POINT('Ctrl Pts',(-31.4547549113176,-0.583874976762647,
-1.34462330629827));
#56352=CARTESIAN_POINT('Ctrl Pts',(-31.4282403689119,-0.1386550916449,-1.53795087161695));
#56353=CARTESIAN_POINT('Ctrl Pts',(-31.4017258265063,0.41212674934496,-1.48817662272349));
#56354=CARTESIAN_POINT('Ctrl Pts',(-31.3752112841006,0.815474489679166,
-1.21816385638901));
#56355=CARTESIAN_POINT('Ctrl Pts',(-31.3486967416949,1.21882223001337,-0.948151090054522));
#56356=CARTESIAN_POINT('Ctrl Pts',(-31.3221821992892,1.47473586969192,-0.457899806279018));
#56357=CARTESIAN_POINT('Ctrl Pts',(-31.2956676568835,1.46566407199324,0.0273980363937246));
#56358=CARTESIAN_POINT('Ctrl Pts',(-31.2691531144778,1.45659227429456,0.512695879066464));
#56359=CARTESIAN_POINT('Ctrl Pts',(-31.2426385720721,1.18253503921864,0.993040280636447));
#56360=CARTESIAN_POINT('Ctrl Pts',(-31.2161240296665,0.769377780148935,
1.24778990849547));
#56361=CARTESIAN_POINT('Ctrl Pts',(-31.1896094872608,0.356220521079224,
1.5025395363545));
#56362=CARTESIAN_POINT('Ctrl Pts',(-31.1630949448551,-0.19603676198427,
1.53169439050258));
#56363=CARTESIAN_POINT('Ctrl Pts',(-31.1365804024494,-0.633720283150774,
1.32186248416896));
#56364=CARTESIAN_POINT('Ctrl Pts',(-31.1100658600437,-1.07140380431728,
1.11203057783535));
#56365=CARTESIAN_POINT('Ctrl Pts',(-31.083551317638,-1.39451356358678,0.663211911020028));
#56366=CARTESIAN_POINT('Ctrl Pts',(-31.0570367752323,-1.45463236773102,
0.181566789582494));
#56367=CARTESIAN_POINT('Ctrl Pts',(-31.0537428654358,-1.4621009453476,0.121731867309701));
#56368=CARTESIAN_POINT('Ctrl Pts',(-31.0504489556393,-1.46551073892982,
0.0613903287927805));
#56369=CARTESIAN_POINT('Ctrl Pts',(-31.0471550458428,-1.46504041338933,
0.000995257504430862));
#56370=CARTESIAN_POINT('Origin',(-17.3,0.,0.));
#56371=CARTESIAN_POINT('',(-30.4758449541571,-1.46163047894353,0.000888967245564962));
#56372=CARTESIAN_POINT('',(-30.5471550458428,-1.46139501350857,0.000694879315414263));
#56373=CARTESIAN_POINT('',(-17.3,-1.4635,-1.79227059055215E-16));
#56374=CARTESIAN_POINT('Ctrl Pts',(-30.4758449541571,-1.46163047894353,
0.000888967245564962));
#56375=CARTESIAN_POINT('Ctrl Pts',(-30.4859372926713,-1.46265825863814,
0.187040242740951));
#56376=CARTESIAN_POINT('Ctrl Pts',(-30.4960296311855,-1.42970103069593,
0.372841193739307));
#56377=CARTESIAN_POINT('Ctrl Pts',(-30.5061219696997,-1.36109128827009,
0.544382552450832));
#56378=CARTESIAN_POINT('Ctrl Pts',(-30.5326365121054,-1.18084010838424,
0.995055171436328));
#56379=CARTESIAN_POINT('Ctrl Pts',(-30.5591510545111,-0.754509777603949,
1.34730588630464));
#56380=CARTESIAN_POINT('Ctrl Pts',(-30.5856655969168,-0.277930812548528,
1.43933190121449));
#56381=CARTESIAN_POINT('Ctrl Pts',(-30.6121801393225,0.198648152506894,
1.53135791612434));
#56382=CARTESIAN_POINT('Ctrl Pts',(-30.6386946817282,0.725475751837446,
1.36315923107573));
#56383=CARTESIAN_POINT('Ctrl Pts',(-30.6652092241338,1.06055906704721,1.01199620736521));
#56384=CARTESIAN_POINT('Ctrl Pts',(-30.6917237665395,1.39564238225697,0.66083318365468));
#56385=CARTESIAN_POINT('Ctrl Pts',(-30.7182383089452,1.53898141334595,0.126705821282239));
#56386=CARTESIAN_POINT('Ctrl Pts',(-30.7447528513509,1.4247348291133,-0.345039889185446));
#56387=CARTESIAN_POINT('Ctrl Pts',(-30.7712673937566,1.31048824488065,-0.816785599653127));
#56388=CARTESIAN_POINT('Ctrl Pts',(-30.7977819361623,0.938656045326382,
-1.22614965821605));
#56389=CARTESIAN_POINT('Ctrl Pts',(-30.824296478568,0.480035582825442,-1.38509483344609));
#56390=CARTESIAN_POINT('Ctrl Pts',(-30.8508110209736,0.0214151203245024,
-1.54404000867613));
#56391=CARTESIAN_POINT('Ctrl Pts',(-30.8773255633793,-0.523993605123111,
-1.45256630057329));
#56392=CARTESIAN_POINT('Ctrl Pts',(-30.903840105785,-0.905662623157868,
-1.15269122987573));
#56393=CARTESIAN_POINT('Ctrl Pts',(-30.927841721909,-1.25115880850179,-0.881236938041353));
#56394=CARTESIAN_POINT('Ctrl Pts',(-30.9518433380331,-1.46248150637196,
-0.439011987974939));
#56395=CARTESIAN_POINT('Ctrl Pts',(-30.9758449541571,-1.46537689164811,
0.00080145734256621));
#56396=CARTESIAN_POINT('Ctrl Pts',(-31.0471550458428,-1.46504041338933,
0.000995257504430862));
#56397=CARTESIAN_POINT('Ctrl Pts',(-31.0239344132336,-1.46172482272134,
-0.424763748792314));
#56398=CARTESIAN_POINT('Ctrl Pts',(-31.0007137806245,-1.26558138617169,
-0.853183139647398));
#56399=CARTESIAN_POINT('Ctrl Pts',(-30.9774931480153,-0.939203181247643,
-1.12553063426295));
#56400=CARTESIAN_POINT('Ctrl Pts',(-30.9509786056096,-0.566527341601074,
-1.4365113606111));
#56401=CARTESIAN_POINT('Ctrl Pts',(-30.9244640632039,-0.024047813288972,
-1.54400123724768));
#56402=CARTESIAN_POINT('Ctrl Pts',(-30.8979495207982,0.439052930346154,
-1.39862587874117));
#56403=CARTESIAN_POINT('Ctrl Pts',(-30.8714349783925,0.902153673981284,
-1.25325052023465));
#56404=CARTESIAN_POINT('Ctrl Pts',(-30.8449204359868,1.28587563293943,-0.855009926585044));
#56405=CARTESIAN_POINT('Ctrl Pts',(-30.8184058935812,1.41396001436526,-0.386831878347976));
#56406=CARTESIAN_POINT('Ctrl Pts',(-30.7918913511755,1.5420443957911,0.0813461698890949));
#56407=CARTESIAN_POINT('Ctrl Pts',(-30.7653768087698,1.4144911996846,0.619461672713624));
#56408=CARTESIAN_POINT('Ctrl Pts',(-30.7388622663641,1.08989069393563,0.980336727661757));
#56409=CARTESIAN_POINT('Ctrl Pts',(-30.7123477239584,0.765290188186653,
1.34121178260988));
#56410=CARTESIAN_POINT('Ctrl Pts',(-30.6858331815527,0.243642372795188,
1.52484638968162));
#56411=CARTESIAN_POINT('Ctrl Pts',(-30.659318639147,-0.235439115098553,
1.44688985324096));
#56412=CARTESIAN_POINT('Ctrl Pts',(-30.6328040967413,-0.714520602992297,
1.3689333168003));
#56413=CARTESIAN_POINT('Ctrl Pts',(-30.6062895543357,-1.15103576338832,
1.02938563684725));
#56414=CARTESIAN_POINT('Ctrl Pts',(-30.57977501193,-1.34447578140578,0.584214598879012));
#56415=CARTESIAN_POINT('Ctrl Pts',(-30.5689016899009,-1.42380340384888,
0.40165485563416));
#56416=CARTESIAN_POINT('Ctrl Pts',(-30.5580283678719,-1.46225235444837,
0.201332117172804));
#56417=CARTESIAN_POINT('Ctrl Pts',(-30.5471550458428,-1.46139501350857,
0.000694879315414263));
#56418=CARTESIAN_POINT('Origin',(-17.3,0.,0.));
#56419=CARTESIAN_POINT('',(-29.9758449541571,-1.46212182688944,-0.00114026912922158));
#56420=CARTESIAN_POINT('',(-30.0471550458428,-1.46248873579703,-0.0012520286611161));
#56421=CARTESIAN_POINT('',(-17.3,-1.4635,-1.79227059055215E-16));
#56422=CARTESIAN_POINT('Ctrl Pts',(-29.9758449541571,-1.46212182688944,
-0.00114026912922158));
#56423=CARTESIAN_POINT('Ctrl Pts',(-29.9935167049038,-1.45976391963976,
0.324536834983454));
#56424=CARTESIAN_POINT('Ctrl Pts',(-30.0111884556506,-1.35239124379562,
0.651624606709122));
#56425=CARTESIAN_POINT('Ctrl Pts',(-30.0288602063974,-1.15246243020409,
0.90595375455135));
#56426=CARTESIAN_POINT('Ctrl Pts',(-30.055374748803,-0.852490962630948,
1.287547014444));
#56427=CARTESIAN_POINT('Ctrl Pts',(-30.0818892912087,-0.344159498409212,
1.50534793168417));
#56428=CARTESIAN_POINT('Ctrl Pts',(-30.1084038336144,0.139035056270542,
1.45931186233288));
#56429=CARTESIAN_POINT('Ctrl Pts',(-30.1349183760201,0.6222296109503,1.41327579298159));
#56430=CARTESIAN_POINT('Ctrl Pts',(-30.1614329184258,1.08028725608808,1.10340273703883));
#56431=CARTESIAN_POINT('Ctrl Pts',(-30.1879474608315,1.3028038547683,0.672029742212693));
#56432=CARTESIAN_POINT('Ctrl Pts',(-30.2144620032372,1.52532045344853,0.240656747386556));
#56433=CARTESIAN_POINT('Ctrl Pts',(-30.2409765456428,1.51229600567119,-0.312216186322958));
#56434=CARTESIAN_POINT('Ctrl Pts',(-30.2674910880485,1.26971315952106,-0.732632480140392));
#56435=CARTESIAN_POINT('Ctrl Pts',(-30.2940056304542,1.02713031337092,-1.15304877395783));
#56436=CARTESIAN_POINT('Ctrl Pts',(-30.3205201728599,0.55498906884799,-1.44100842788317));
#56437=CARTESIAN_POINT('Ctrl Pts',(-30.3470347152656,0.0701627215092274,
-1.46424009333443));
#56438=CARTESIAN_POINT('Ctrl Pts',(-30.3735492576713,-0.414663625829532,
-1.48747175878569));
#56439=CARTESIAN_POINT('Ctrl Pts',(-30.400063800077,-0.912175075984127,
-1.24597543576286));
#56440=CARTESIAN_POINT('Ctrl Pts',(-30.4265783424827,-1.19384478656572,
-0.850680012700103));
#56441=CARTESIAN_POINT('Ctrl Pts',(-30.4430005463741,-1.36830140536949,
-0.60584750020262));
#56442=CARTESIAN_POINT('Ctrl Pts',(-30.4594227502656,-1.45995808084902,
-0.302015478194993));
#56443=CARTESIAN_POINT('Ctrl Pts',(-30.4758449541571,-1.46163047894353,
0.000888967245564962));
#56444=CARTESIAN_POINT('Ctrl Pts',(-30.5471550458428,-1.46139501350857,
0.000694879315414263));
#56445=CARTESIAN_POINT('Ctrl Pts',(-30.5315138254662,-1.46016173277417,
-0.28792080269058));
#56446=CARTESIAN_POINT('Ctrl Pts',(-30.5158726050895,-1.37759319561782,
-0.577187268273936));
#56447=CARTESIAN_POINT('Ctrl Pts',(-30.5002313847129,-1.21836979964959,
-0.815166765534423));
#56448=CARTESIAN_POINT('Ctrl Pts',(-30.4737168423072,-0.948458924237074,
-1.21858269599621));
#56449=CARTESIAN_POINT('Ctrl Pts',(-30.4472022999015,-0.458272297773157,
-1.47462016093639));
#56450=CARTESIAN_POINT('Ctrl Pts',(-30.4206877574959,0.0270278208791361,
-1.46567094575439));
#56451=CARTESIAN_POINT('Ctrl Pts',(-30.3941732150902,0.512327939531434,
-1.45672173057239));
#56452=CARTESIAN_POINT('Ctrl Pts',(-30.3676586726845,0.992741550372114,
-1.18278583526821));
#56453=CARTESIAN_POINT('Ctrl Pts',(-30.3411441302788,1.24759553021592,-0.769692937030927));
#56454=CARTESIAN_POINT('Ctrl Pts',(-30.3146295878731,1.50244951005973,-0.356600038793641));
#56455=CARTESIAN_POINT('Ctrl Pts',(-30.2881150454674,1.53174385890668,0.195649862376755));
#56456=CARTESIAN_POINT('Ctrl Pts',(-30.2616005030617,1.32202251450984,0.633386371387252));
#56457=CARTESIAN_POINT('Ctrl Pts',(-30.2350859606561,1.11230117011302,1.07112288039774));
#56458=CARTESIAN_POINT('Ctrl Pts',(-30.2085714182504,0.663564132472433,
1.39434599724833));
#56459=CARTESIAN_POINT('Ctrl Pts',(-30.1820568758447,0.181934211913454,
1.45458645905476));
#56460=CARTESIAN_POINT('Ctrl Pts',(-30.155542333439,-0.29969570864554,1.51482692086119));
#56461=CARTESIAN_POINT('Ctrl Pts',(-30.1290277910333,-0.814218512122926,
1.31208472762344));
#56462=CARTESIAN_POINT('Ctrl Pts',(-30.1025132486276,-1.12529336338979,
0.93948745102898));
#56463=CARTESIAN_POINT('Ctrl Pts',(-30.084060514366,-1.34178518429572,0.680179240975944));
#56464=CARTESIAN_POINT('Ctrl Pts',(-30.0656077801044,-1.45973837855422,
0.338602880955323));
#56465=CARTESIAN_POINT('Ctrl Pts',(-30.0471550458428,-1.46248873579703,
-0.0012520286611161));
#56466=CARTESIAN_POINT('Origin',(-17.3,0.,0.));
#56467=CARTESIAN_POINT('',(-29.4758449541571,-1.4657700110061,-0.000426988761815655));
#56468=CARTESIAN_POINT('',(-29.5471550458428,-1.46589706054516,-0.000165931013407645));
#56469=CARTESIAN_POINT('',(-17.3,-1.4635,-1.79227059055215E-16));
#56470=CARTESIAN_POINT('Ctrl Pts',(-29.4758449541571,-1.4657700110061,-0.000426988761815655));
#56471=CARTESIAN_POINT('Ctrl Pts',(-29.5010961171364,-1.46399203858896,
0.461954784892472));
#56472=CARTESIAN_POINT('Ctrl Pts',(-29.5263472801157,-1.22690634601226,
0.925906164443394));
#56473=CARTESIAN_POINT('Ctrl Pts',(-29.551598443095,-0.850378430228461,
1.19405962322649));
#56474=CARTESIAN_POINT('Ctrl Pts',(-29.5781129855007,-0.455011872333391,
1.4756294764631));
#56475=CARTESIAN_POINT('Ctrl Pts',(-29.6046275279064,0.0940992608542971,
1.54131874862981));
#56476=CARTESIAN_POINT('Ctrl Pts',(-29.631142070312,0.544726335503297,1.3609537383125));
#56477=CARTESIAN_POINT('Ctrl Pts',(-29.6576566127177,0.99535341015231,1.18058872799518));
#56478=CARTESIAN_POINT('Ctrl Pts',(-29.6841711551234,1.34749642626262,0.754169435193818));
#56479=CARTESIAN_POINT('Ctrl Pts',(-29.7106856975291,1.43940205832593,0.277567240330494));
#56480=CARTESIAN_POINT('Ctrl Pts',(-29.7372002399348,1.53130769038923,-0.199034954532819));
#56481=CARTESIAN_POINT('Ctrl Pts',(-29.7637147823405,1.36297593840554,-0.725820051458098));
#56482=CARTESIAN_POINT('Ctrl Pts',(-29.7902293247462,1.0117282866194,-1.06081465509852));
#56483=CARTESIAN_POINT('Ctrl Pts',(-29.8167438671519,0.66048063483325,-1.39580925873894));
#56484=CARTESIAN_POINT('Ctrl Pts',(-29.8432584095575,0.126317083244657,
-1.53901336909452));
#56485=CARTESIAN_POINT('Ctrl Pts',(-29.8697729519632,-0.345399754430043,
-1.42464762943588));
#56486=CARTESIAN_POINT('Ctrl Pts',(-29.8962874943689,-0.817116592104736,
-1.31028188977725));
#56487=CARTESIAN_POINT('Ctrl Pts',(-29.9228020367746,-1.22638671586554,
-0.938346300104411));
#56488=CARTESIAN_POINT('Ctrl Pts',(-29.9493165791803,-1.38521604228366,
-0.479685703995432));
#56489=CARTESIAN_POINT('Ctrl Pts',(-29.9581593708392,-1.43818677137845,
-0.326719077926747));
#56490=CARTESIAN_POINT('Ctrl Pts',(-29.9670021624982,-1.46330170334077,
-0.16410628313783));
#56491=CARTESIAN_POINT('Ctrl Pts',(-29.9758449541571,-1.46212182688944,
-0.00114026912922158));
#56492=CARTESIAN_POINT('Ctrl Pts',(-30.0471550458428,-1.46248873579703,
-0.0012520286611161));
#56493=CARTESIAN_POINT('Ctrl Pts',(-30.0390932376987,-1.4636903383403,-0.149731112536215));
#56494=CARTESIAN_POINT('Ctrl Pts',(-30.0310314295547,-1.44290288229849,
-0.297881618793177));
#56495=CARTESIAN_POINT('Ctrl Pts',(-30.0229696214106,-1.39873673526752,
-0.438699634993247));
#56496=CARTESIAN_POINT('Ctrl Pts',(-29.9964550790049,-1.25347835682203,
-0.901837084469851));
#56497=CARTESIAN_POINT('Ctrl Pts',(-29.9699405365992,-0.855334700874716,
-1.2856596234719));
#56498=CARTESIAN_POINT('Ctrl Pts',(-29.9434259941935,-0.387189020630112,
-1.41386225872025));
#56499=CARTESIAN_POINT('Ctrl Pts',(-29.9169114517878,0.0809566596144957,
-1.54206489396861));
#56500=CARTESIAN_POINT('Ctrl Pts',(-29.8903969093821,0.619104364156387,
-1.41464762546327));
#56501=CARTESIAN_POINT('Ctrl Pts',(-29.8638823669764,0.980061398999209,
-1.0901382841281));
#56502=CARTESIAN_POINT('Ctrl Pts',(-29.8373678245708,1.34101843384203,-0.765628942792929));
#56503=CARTESIAN_POINT('Ctrl Pts',(-29.8108532821651,1.52478479898578,-0.244027528627926));
#56504=CARTESIAN_POINT('Ctrl Pts',(-29.7843387397594,1.44694927705943,0.235073635159805));
#56505=CARTESIAN_POINT('Ctrl Pts',(-29.7578241973537,1.36911375513308,0.714174798947536));
#56506=CARTESIAN_POINT('Ctrl Pts',(-29.731309654948,1.02967634613663,1.150775712358));
#56507=CARTESIAN_POINT('Ctrl Pts',(-29.7047951125423,0.584554183720977,
1.34432817073226));
#56508=CARTESIAN_POINT('Ctrl Pts',(-29.6782805701366,0.139432021305321,
1.53788062910652));
#56509=CARTESIAN_POINT('Ctrl Pts',(-29.6517660277309,-0.411374894529538,
1.48838463244457));
#56510=CARTESIAN_POINT('Ctrl Pts',(-29.6252514853253,-0.814858989379939,
1.21857566517502));
#56511=CARTESIAN_POINT('Ctrl Pts',(-29.5992193388311,-1.21100224180705,
0.9536755038247));
#56512=CARTESIAN_POINT('Ctrl Pts',(-29.5731871923369,-1.465134583482,0.476406034057459));
#56513=CARTESIAN_POINT('Ctrl Pts',(-29.5471550458428,-1.46589706054516,
-0.000165931013407645));
#56514=CARTESIAN_POINT('Origin',(-17.3,0.,0.));
#56515=CARTESIAN_POINT('',(-28.9758449541571,-1.46341902613524,0.00135233047681406));
#56516=CARTESIAN_POINT('',(-29.0471550458428,-1.46298909506461,0.00133440455282766));
#56517=CARTESIAN_POINT('',(-17.3,-1.4635,-1.79227059055215E-16));
#56518=CARTESIAN_POINT('Ctrl Pts',(-28.9758449541571,-1.46341902613524,
0.00135233047681406));
#56519=CARTESIAN_POINT('Ctrl Pts',(-28.9821609869633,-1.46448859466354,
0.117490729182389));
#56520=CARTESIAN_POINT('Ctrl Pts',(-28.9884770197694,-1.45183179978412,
0.233398749586752));
#56521=CARTESIAN_POINT('Ctrl Pts',(-28.9947930525756,-1.42456033886225,
0.345759597637241));
#56522=CARTESIAN_POINT('Ctrl Pts',(-29.0213075949813,-1.31007545107446,
0.8174475324222));
#56523=CARTESIAN_POINT('Ctrl Pts',(-29.047822137387,-0.938036495013489,
1.2266236952684));
#56524=CARTESIAN_POINT('Ctrl Pts',(-29.0743366797926,-0.479335794560193,
1.38533716274088));
#56525=CARTESIAN_POINT('Ctrl Pts',(-29.1008512221983,-0.0206350941068899,
1.54405063021337));
#56526=CARTESIAN_POINT('Ctrl Pts',(-29.127365764604,0.524727350738727,1.45230140231214));
#56527=CARTESIAN_POINT('Ctrl Pts',(-29.1538803070097,0.906244828142636,
1.15223355700237));
#56528=CARTESIAN_POINT('Ctrl Pts',(-29.1803948494154,1.28776230554654,0.852165711692601));
#56529=CARTESIAN_POINT('Ctrl Pts',(-29.2069093918211,1.50543481550872,0.343779248974287));
#56530=CARTESIAN_POINT('Ctrl Pts',(-29.2334239342268,1.45927669667193,-0.139403661960002));
#56531=CARTESIAN_POINT('Ctrl Pts',(-29.2599384766324,1.41311857783515,-0.622586572894284));
#56532=CARTESIAN_POINT('Ctrl Pts',(-29.2864530190381,1.10312983019941,-1.08056593204455));
#56533=CARTESIAN_POINT('Ctrl Pts',(-29.3129675614438,0.671700643279443,
-1.30297356237016));
#56534=CARTESIAN_POINT('Ctrl Pts',(-29.3394821038495,0.240271456359465,
-1.52538119269578));
#56535=CARTESIAN_POINT('Ctrl Pts',(-29.3659966462552,-0.312598169844754,
-1.51221709419673));
#56536=CARTESIAN_POINT('Ctrl Pts',(-29.3925111886609,-0.732953175826774,
-1.26952806210145));
#56537=CARTESIAN_POINT('Ctrl Pts',(-29.4190257310666,-1.15330818180879,
-1.02683903000616));
#56538=CARTESIAN_POINT('Ctrl Pts',(-29.4455402734722,-1.44114856756861,
-0.554625064314648));
#56539=CARTESIAN_POINT('Ctrl Pts',(-29.4720548158779,-1.4642577691473,-0.0697928643156378));
#56540=CARTESIAN_POINT('Ctrl Pts',(-29.4733181953043,-1.46535888903042,
-0.0466913143301533));
#56541=CARTESIAN_POINT('Ctrl Pts',(-29.4745815747307,-1.46585896745433,
-0.023561116106705));
#56542=CARTESIAN_POINT('Ctrl Pts',(-29.4758449541571,-1.4657700110061,-0.000426988761815655));
#56543=CARTESIAN_POINT('Ctrl Pts',(-29.5471550458428,-1.46589706054516,
-0.000165931013407645));
#56544=CARTESIAN_POINT('Ctrl Pts',(-29.5466726499313,-1.46591118983788,
-0.00899718000605618));
#56545=CARTESIAN_POINT('Ctrl Pts',(-29.5461902540197,-1.46583831452614,
-0.017828189482769));
#56546=CARTESIAN_POINT('Ctrl Pts',(-29.5457078581082,-1.46567772600194,
-0.0266576036401217));
#56547=CARTESIAN_POINT('Ctrl Pts',(-29.5191933157025,-1.4568510939076,-0.511959967308562));
#56548=CARTESIAN_POINT('Ctrl Pts',(-29.4926787732968,-1.18303655585298,
-0.992442756768303));
#56549=CARTESIAN_POINT('Ctrl Pts',(-29.4661642308911,-0.770008044804517,
-1.24740107233655));
#56550=CARTESIAN_POINT('Ctrl Pts',(-29.4396496884855,-0.356979533756049,
-1.50235938790479));
#56551=CARTESIAN_POINT('Ctrl Pts',(-29.4131351460798,0.195262950286247,
-1.53179322958155));
#56552=CARTESIAN_POINT('Ctrl Pts',(-29.3866206036741,0.63305241921202,-1.32218246050227));
#56553=CARTESIAN_POINT('Ctrl Pts',(-29.3601060612684,1.07084188813778,-1.11257169142301));
#56554=CARTESIAN_POINT('Ctrl Pts',(-29.3335915188627,1.39417834194701,-0.663916311587708));
#56555=CARTESIAN_POINT('Ctrl Pts',(-29.307076976457,1.45454045757213,-0.182301622636509));
#56556=CARTESIAN_POINT('Ctrl Pts',(-29.2805624340513,1.51490257319725,0.299313066314696));
#56557=CARTESIAN_POINT('Ctrl Pts',(-29.2540478916456,1.31229035063826,0.813887064381816));
#56558=CARTESIAN_POINT('Ctrl Pts',(-29.22753334924,0.939771660868593,1.12505602072));
#56559=CARTESIAN_POINT('Ctrl Pts',(-29.2010188068343,0.567252971098922,
1.43622497705819));
#56560=CARTESIAN_POINT('Ctrl Pts',(-29.1745042644286,0.0248278141185692,
1.54398889166744));
#56561=CARTESIAN_POINT('Ctrl Pts',(-29.1479897220229,-0.438346311650147,
1.39884750255085));
#56562=CARTESIAN_POINT('Ctrl Pts',(-29.1214751796172,-0.901520437418864,
1.25370611343427));
#56563=CARTESIAN_POINT('Ctrl Pts',(-29.0949606372115,-1.28544353197594,
0.855659420591842));
#56564=CARTESIAN_POINT('Ctrl Pts',(-29.0684460948058,-1.41376441286716,
0.387546138208605));
#56565=CARTESIAN_POINT('Ctrl Pts',(-29.0613490784848,-1.44811142787792,
0.262248573033834));
#56566=CARTESIAN_POINT('Ctrl Pts',(-29.0542520621638,-1.4641459298896,0.131931116546837));
#56567=CARTESIAN_POINT('Ctrl Pts',(-29.0471550458428,-1.46298909506461,
0.00133440455282766));
#56568=CARTESIAN_POINT('Origin',(-17.3,0.,0.));
#56569=CARTESIAN_POINT('',(-28.4758449541571,-1.46109929919025,-0.000194400770703457));
#56570=CARTESIAN_POINT('',(-28.5471550458428,-1.46119040624119,-0.000426588110409748));
#56571=CARTESIAN_POINT('',(-17.3,-1.4635,-1.79227059055215E-16));
#56572=CARTESIAN_POINT('Ctrl Pts',(-28.4758449541571,-1.46109929919025,
-0.000194400770703457));
#56573=CARTESIAN_POINT('Ctrl Pts',(-28.4897403991958,-1.46079627679699,
0.256337369532174));
#56574=CARTESIAN_POINT('Ctrl Pts',(-28.5036358442345,-1.39658427978759,
0.513011004497548));
#56575=CARTESIAN_POINT('Ctrl Pts',(-28.5175312892732,-1.26934288368266,
0.733273824748846));
#56576=CARTESIAN_POINT('Ctrl Pts',(-28.5440458316789,-1.02654768112642,
1.15356751607571));
#56577=CARTESIAN_POINT('Ctrl Pts',(-28.5705603740846,-0.55426102439479,
1.44128861530504));
#56578=CARTESIAN_POINT('Ctrl Pts',(-28.5970749164903,-0.0694230026690815,
1.46427535153673));
#56579=CARTESIAN_POINT('Ctrl Pts',(-28.623589458896,0.415415019056634,1.48726208776842));
#56580=CARTESIAN_POINT('Ctrl Pts',(-28.6501040013017,0.912804405776441,
1.24551446100245));
#56581=CARTESIAN_POINT('Ctrl Pts',(-28.6766185437074,1.19427438370317,0.850076793500457));
#56582=CARTESIAN_POINT('Ctrl Pts',(-28.703133086113,1.4757443616299,0.45463912599847));
#56583=CARTESIAN_POINT('Ctrl Pts',(-28.7296476285187,1.54129493076356,-0.0944885822395179));
#56584=CARTESIAN_POINT('Ctrl Pts',(-28.7561621709244,1.36081610152252,-0.54507008380085));
#56585=CARTESIAN_POINT('Ctrl Pts',(-28.7826767133301,1.18033727228147,-0.995651585362183));
#56586=CARTESIAN_POINT('Ctrl Pts',(-28.8091912557358,0.753829044665707,
-1.34768688024685));
#56587=CARTESIAN_POINT('Ctrl Pts',(-28.8357057981415,0.277203650402953,
-1.43947212359979));
#56588=CARTESIAN_POINT('Ctrl Pts',(-28.8622203405472,-0.199421743859794,
-1.53125736695273));
#56589=CARTESIAN_POINT('Ctrl Pts',(-28.8887348829528,-0.726164304769535,
-1.36279255877395));
#56590=CARTESIAN_POINT('Ctrl Pts',(-28.9152494253585,-1.0610701754671,-1.01146030132271));
#56591=CARTESIAN_POINT('Ctrl Pts',(-28.935447934958,-1.31619807247997,-0.743818949412031));
#56592=CARTESIAN_POINT('Ctrl Pts',(-28.9556464445576,-1.45999857363774,
-0.370055265575945));
#56593=CARTESIAN_POINT('Ctrl Pts',(-28.9758449541571,-1.46341902613524,
0.00135233047681406));
#56594=CARTESIAN_POINT('Ctrl Pts',(-29.0471550458428,-1.46298909506461,
0.00133440455282766));
#56595=CARTESIAN_POINT('Ctrl Pts',(-29.0277375197581,-1.459823980406,-0.355979845128287));
#56596=CARTESIAN_POINT('Ctrl Pts',(-29.0083199936734,-1.32796855895135,
-0.715384535896872));
#56597=CARTESIAN_POINT('Ctrl Pts',(-28.9889024675888,-1.09038580476693,
-0.979786007806199));
#56598=CARTESIAN_POINT('Ctrl Pts',(-28.9623879251831,-0.765967648550108,
-1.34082499951372));
#56599=CARTESIAN_POINT('Ctrl Pts',(-28.9358733827774,-0.244412668891087,
-1.52472311100471));
#56600=CARTESIAN_POINT('Ctrl Pts',(-28.9093588403717,0.234708140222739,
-1.44700860855878));
#56601=CARTESIAN_POINT('Ctrl Pts',(-28.882844297966,0.713828949336565,-1.36929410611286));
#56602=CARTESIAN_POINT('Ctrl Pts',(-28.8563297555604,1.1505155879052,-1.02996698973001));
#56603=CARTESIAN_POINT('Ctrl Pts',(-28.8298152131547,1.34418047428712,-0.58489373126688));
#56604=CARTESIAN_POINT('Ctrl Pts',(-28.803300670749,1.53784536066904,-0.139820472803748));
#56605=CARTESIAN_POINT('Ctrl Pts',(-28.7767861283433,1.48848849486424,0.410998927739651));
#56606=CARTESIAN_POINT('Ctrl Pts',(-28.7502715859376,1.21878145295217,0.814551161235334));
#56607=CARTESIAN_POINT('Ctrl Pts',(-28.7237570435319,0.94907441104011,1.21810339473101));
#56608=CARTESIAN_POINT('Ctrl Pts',(-28.6972425011262,0.45901719302078,1.47438846117896));
#56609=CARTESIAN_POINT('Ctrl Pts',(-28.6707279587205,-0.0262873847002612,
1.46568441273545));
#56610=CARTESIAN_POINT('Ctrl Pts',(-28.6442134163149,-0.511591962421303,
1.45698036429194));
#56611=CARTESIAN_POINT('Ctrl Pts',(-28.6176988739092,-0.992143899844064,
1.18328720095696));
#56612=CARTESIAN_POINT('Ctrl Pts',(-28.5911843315035,-1.24720653486975,
0.77032310344961));
#56613=CARTESIAN_POINT('Ctrl Pts',(-28.5765079029499,-1.38838975735801,
0.541737673630878));
#56614=CARTESIAN_POINT('Ctrl Pts',(-28.5618314743964,-1.46048564494658,
0.270481227632335));
#56615=CARTESIAN_POINT('Ctrl Pts',(-28.5471550458428,-1.46119040624119,
-0.000426588110409748));
#56616=CARTESIAN_POINT('Origin',(-17.3,0.,0.));
#56617=CARTESIAN_POINT('',(-27.9758449541571,-1.46413482731608,-0.00128332369852588));
#56618=CARTESIAN_POINT('',(-28.0471550458428,-1.46455866562899,-0.00118106958518242));
#56619=CARTESIAN_POINT('',(-17.3,-1.4635,-1.79227059055215E-16));
#56620=CARTESIAN_POINT('Ctrl Pts',(-27.9758449541571,-1.46413482731608,
-0.00128332369852588));
#56621=CARTESIAN_POINT('Ctrl Pts',(-27.9973198114283,-1.46051051517567,
0.393098621091974));
#56622=CARTESIAN_POINT('Ctrl Pts',(-28.0187946686996,-1.29581441774694,
0.790148035238067));
#56623=CARTESIAN_POINT('Ctrl Pts',(-28.0402695259709,-1.01119225149223,
1.06132562813666));
#56624=CARTESIAN_POINT('Ctrl Pts',(-28.0667840683766,-0.659775410791775,
1.39614274452351));
#56625=CARTESIAN_POINT('Ctrl Pts',(-28.0932986107822,-0.125539583016236,
1.53907698601051));
#56626=CARTESIAN_POINT('Ctrl Pts',(-28.1198131531879,0.346119418784083,
1.42447295739799));
#56627=CARTESIAN_POINT('Ctrl Pts',(-28.1463276955936,0.817778420584388,
1.30986892878547));
#56628=CARTESIAN_POINT('Ctrl Pts',(-28.1728422379993,1.22686059640947,0.93772663007344));
#56629=CARTESIAN_POINT('Ctrl Pts',(-28.199356780405,1.38545819480999,0.478985854542129));
#56630=CARTESIAN_POINT('Ctrl Pts',(-28.2258713228107,1.54405579321051,0.0202450790108123));
#56631=CARTESIAN_POINT('Ctrl Pts',(-28.2523858652164,1.45216881418645,-0.5250941733398));
#56632=CARTESIAN_POINT('Ctrl Pts',(-28.2789004076221,1.15200461028516,-0.906535843913156));
#56633=CARTESIAN_POINT('Ctrl Pts',(-28.3054149500277,0.85184040638387,-1.28797751448652));
#56634=CARTESIAN_POINT('Ctrl Pts',(-28.3319294924334,0.343398977605346,
-1.50552160328263));
#56635=CARTESIAN_POINT('Ctrl Pts',(-28.3584440348391,-0.139772258755166,
-1.45924143790536));
#56636=CARTESIAN_POINT('Ctrl Pts',(-28.3849585772448,-0.622943495115664,
-1.41296127252808));
#56637=CARTESIAN_POINT('Ctrl Pts',(-28.4114731196505,-1.08084453905814,
-1.10285685297743));
#56638=CARTESIAN_POINT('Ctrl Pts',(-28.4379876620562,-1.30314318683895,
-0.671371501489916));
#56639=CARTESIAN_POINT('Ctrl Pts',(-28.4506067594232,-1.40894204385757,
-0.466014170424791));
#56640=CARTESIAN_POINT('Ctrl Pts',(-28.4632258567901,-1.46137448786354,
-0.233162785601588));
#56641=CARTESIAN_POINT('Ctrl Pts',(-28.4758449541571,-1.46109929919025,
-0.000194400770703457));
#56642=CARTESIAN_POINT('Ctrl Pts',(-28.5471550458428,-1.46119040624119,
-0.000426588110409748));
#56643=CARTESIAN_POINT('Ctrl Pts',(-28.5353169319907,-1.46175887181942,
-0.21894279963225));
#56644=CARTESIAN_POINT('Ctrl Pts',(-28.5234788181386,-1.41587918011866,
-0.437232186984281));
#56645=CARTESIAN_POINT('Ctrl Pts',(-28.5116407042864,-1.32234232213604,
-0.632718426646407));
#56646=CARTESIAN_POINT('Ctrl Pts',(-28.4851261618807,-1.11284214174804,
-1.07056082755534));
#56647=CARTESIAN_POINT('Ctrl Pts',(-28.458611619475,-0.664268448343429,
-1.39401059769349));
#56648=CARTESIAN_POINT('Ctrl Pts',(-28.4320970770694,-0.18266902172827,
-1.45449436328604));
#56649=CARTESIAN_POINT('Ctrl Pts',(-28.4055825346637,0.298930404886896,
-1.5149781288786));
#56650=CARTESIAN_POINT('Ctrl Pts',(-28.379067992258,0.813555564712618,-1.31249588992556));
#56651=CARTESIAN_POINT('Ctrl Pts',(-28.3525534498523,1.12481860626874,-0.940055810748326));
#56652=CARTESIAN_POINT('Ctrl Pts',(-28.3260389074466,1.43608164782485,-0.567615731571103));
#56653=CARTESIAN_POINT('Ctrl Pts',(-28.2995243650409,1.54398257111138,-0.0252178121697132));
#56654=CARTESIAN_POINT('Ctrl Pts',(-28.2730098226352,1.3989581805841,0.437992960339399));
#56655=CARTESIAN_POINT('Ctrl Pts',(-28.2464952802295,1.25393379005681,0.901203732848524));
#56656=CARTESIAN_POINT('Ctrl Pts',(-28.2199807378239,0.855984085715685,
1.28522735846536));
#56657=CARTESIAN_POINT('Ctrl Pts',(-28.1934661954182,0.387903231060652,
1.41366647681225));
#56658=CARTESIAN_POINT('Ctrl Pts',(-28.1669516530125,-0.0801776235943734,
1.54210559515913));
#56659=CARTESIAN_POINT('Ctrl Pts',(-28.1404371106068,-0.61838962856331,
1.41496020623609));
#56660=CARTESIAN_POINT('Ctrl Pts',(-28.1139225682011,-0.979510554100306,
1.09063325583633));
#56661=CARTESIAN_POINT('Ctrl Pts',(-28.091666727415,-1.28262911071393,0.818398915137616));
#56662=CARTESIAN_POINT('Ctrl Pts',(-28.0694108866289,-1.46097587203959,
0.407237771902873));
#56663=CARTESIAN_POINT('Ctrl Pts',(-28.0471550458428,-1.46455866562899,
-0.00118106958518242));
#56664=CARTESIAN_POINT('Origin',(-17.3,0.,0.));
#56665=CARTESIAN_POINT('',(-27.4758449541571,-1.46536634381812,0.000808685770614676));
#56666=CARTESIAN_POINT('',(-27.5471550458428,-1.46502789863774,0.00100125412595091));
#56667=CARTESIAN_POINT('',(-17.3,-1.4635,-1.79227059055215E-16));
#56668=CARTESIAN_POINT('Ctrl Pts',(-27.4758449541571,-1.46536634381812,
0.000808685770614676));
#56669=CARTESIAN_POINT('Ctrl Pts',(-27.4783846812552,-1.46567494044697,
0.0473483563683534));
#56670=CARTESIAN_POINT('Ctrl Pts',(-27.4809244083533,-1.46365077701734,
0.0938608341503805));
#56671=CARTESIAN_POINT('Ctrl Pts',(-27.4834641354515,-1.4592060860354,0.140140846632458));
#56672=CARTESIAN_POINT('Ctrl Pts',(-27.5099786778571,-1.41280387707044,
0.623300377591606));
#56673=CARTESIAN_POINT('Ctrl Pts',(-27.5364932202628,-1.10258380539034,
1.08112307711105));
#56674=CARTESIAN_POINT('Ctrl Pts',(-27.5630077626685,-0.671042316865148,
1.30331272816384));
#56675=CARTESIAN_POINT('Ctrl Pts',(-27.5895223050742,-0.239500828339974,
1.52550237921661));
#56676=CARTESIAN_POINT('Ctrl Pts',(-27.6160368474799,0.313362077030277,
1.51205898180275));
#56677=CARTESIAN_POINT('Ctrl Pts',(-27.6425513898856,0.733594426886151,
1.26915762427651));
#56678=CARTESIAN_POINT('Ctrl Pts',(-27.6690659322913,1.15382677674203,1.02625626675027));
#56679=CARTESIAN_POINT('Ctrl Pts',(-27.6955804746969,1.44142857108353,0.553896949111648));
#56680=CARTESIAN_POINT('Ctrl Pts',(-27.7220950171026,1.4642928405016,0.0690531365931595));
#56681=CARTESIAN_POINT('Ctrl Pts',(-27.7486095595083,1.48715710991968,-0.415790675925329));
#56682=CARTESIAN_POINT('Ctrl Pts',(-27.775124101914,1.24528385441433,-0.913118983323688));
#56683=CARTESIAN_POINT('Ctrl Pts',(-27.8016386443197,0.849775102535385,
-1.19448906798203));
#56684=CARTESIAN_POINT('Ctrl Pts',(-27.8281531867254,0.454266350656434,
-1.47585915264038));
#56685=CARTESIAN_POINT('Ctrl Pts',(-27.8546677291311,-0.0948778975961176,
-1.54127101455871));
#56686=CARTESIAN_POINT('Ctrl Pts',(-27.8811822715368,-0.545413797321521,
-1.36067837790895));
#56687=CARTESIAN_POINT('Ctrl Pts',(-27.9076968139424,-0.995949697046905,
-1.18008574125919));
#56688=CARTESIAN_POINT('Ctrl Pts',(-27.9342113563481,-1.34787724824515,
-0.753488606041366));
#56689=CARTESIAN_POINT('Ctrl Pts',(-27.9607258987538,-1.4395420970316,-0.27684004278912));
#56690=CARTESIAN_POINT('Ctrl Pts',(-27.9657655838882,-1.45696506321787,
-0.186242262830691));
#56691=CARTESIAN_POINT('Ctrl Pts',(-27.9708052690226,-1.46498537508856,
-0.0938362473031713));
#56692=CARTESIAN_POINT('Ctrl Pts',(-27.9758449541571,-1.46413482731608,
-0.00128332369852588));
#56693=CARTESIAN_POINT('Ctrl Pts',(-28.0471550458428,-1.46455866562899,
-0.00118106958518242));
#56694=CARTESIAN_POINT('Ctrl Pts',(-28.0428963442232,-1.46524424066561,
-0.0793328679570782));
#56695=CARTESIAN_POINT('Ctrl Pts',(-28.0386376426036,-1.45953072434846,
-0.157384255245247));
#56696=CARTESIAN_POINT('Ctrl Pts',(-28.0343789409841,-1.44706784773524,
-0.234342630310688));
#56697=CARTESIAN_POINT('Ctrl Pts',(-28.0078643985784,-1.36947436972812,
-0.713483054181464));
#56698=CARTESIAN_POINT('Ctrl Pts',(-27.9813498561727,-1.03025756760883,
-1.15025539004653));
#56699=CARTESIAN_POINT('Ctrl Pts',(-27.954835313767,-0.585233241495049,
-1.34403269207979));
#56700=CARTESIAN_POINT('Ctrl Pts',(-27.9283207713613,-0.140208915381278,
-1.53780999411304));
#56701=CARTESIAN_POINT('Ctrl Pts',(-27.9018062289556,0.41062293472698,-1.48859226231448));
#56702=CARTESIAN_POINT('Ctrl Pts',(-27.87529168655,0.814243281120257,-1.21898716296791));
#56703=CARTESIAN_POINT('Ctrl Pts',(-27.8487771441443,1.21786362751354,-0.94938206362134));
#56704=CARTESIAN_POINT('Ctrl Pts',(-27.8222626017386,1.47427247019185,-0.459389596726757));
#56705=CARTESIAN_POINT('Ctrl Pts',(-27.7957480593329,1.4656910059545,0.0259171640831991));
#56706=CARTESIAN_POINT('Ctrl Pts',(-27.7692335169272,1.45710954171716,0.511223924893148));
#56707=CARTESIAN_POINT('Ctrl Pts',(-27.7427189745215,1.18353777056415,0.991844979618477));
#56708=CARTESIAN_POINT('Ctrl Pts',(-27.7162044321158,0.770638112946094,
1.24701191782794));
#56709=CARTESIAN_POINT('Ctrl Pts',(-27.6896898897102,0.357738455328029,
1.50217885603741));
#56710=CARTESIAN_POINT('Ctrl Pts',(-27.6631753473044,-0.194489088755087,
1.53189167773102));
#56711=CARTESIAN_POINT('Ctrl Pts',(-27.6366608048988,-0.632384393711719,
1.32250209940094));
#56712=CARTESIAN_POINT('Ctrl Pts',(-27.6101462624931,-1.07027969866835,
1.11311252107087));
#56713=CARTESIAN_POINT('Ctrl Pts',(-27.5836317200874,-1.39384276449848,
0.664620542717102));
#56714=CARTESIAN_POINT('Ctrl Pts',(-27.5571171776817,-1.45444817619946,
0.183036409165274));
#56715=CARTESIAN_POINT('Ctrl Pts',(-27.5537964670688,-1.4620384649836,0.122722279701757));
#56716=CARTESIAN_POINT('Ctrl Pts',(-27.5504757564558,-1.46550417497613,
0.0618890887112012));
#56717=CARTESIAN_POINT('Ctrl Pts',(-27.5471550458428,-1.46502789863774,
0.00100125412595091));
#56718=CARTESIAN_POINT('Origin',(-17.3,0.,0.));
#56719=CARTESIAN_POINT('',(-26.9758449541571,-1.46162142615836,0.000882726340737661));
#56720=CARTESIAN_POINT('',(-27.0471550458428,-1.46138800853787,0.00068780616967229));
#56721=CARTESIAN_POINT('',(-17.3,-1.4635,-1.79227059055215E-16));
#56722=CARTESIAN_POINT('Ctrl Pts',(-26.9758449541571,-1.46162142615836,
0.000882726340737661));
#56723=CARTESIAN_POINT('Ctrl Pts',(-26.9859640934878,-1.46264431827847,
0.187531233801553));
#56724=CARTESIAN_POINT('Ctrl Pts',(-26.9960832328184,-1.42950625207749,
0.373830171742523));
#56725=CARTESIAN_POINT('Ctrl Pts',(-27.0062023721491,-1.36054056748059,
0.54575747604334));
#56726=CARTESIAN_POINT('Ctrl Pts',(-27.0327169145548,-1.17983413494441,
0.996247745187448));
#56727=CARTESIAN_POINT('Ctrl Pts',(-27.0592314569605,-0.753148119342491,
1.34806753024541));
#56728=CARTESIAN_POINT('Ctrl Pts',(-27.0857459993662,-0.276476417512137,
1.4396119786169));
#56729=CARTESIAN_POINT('Ctrl Pts',(-27.1122605417718,0.200195284318217,
1.53115642698839));
#56730=CARTESIAN_POINT('Ctrl Pts',(-27.1387750841775,0.726852672377007,
1.3624255386734));
#56731=CARTESIAN_POINT('Ctrl Pts',(-27.1652896265832,1.06158101309092,1.01092413714505));
#56732=CARTESIAN_POINT('Ctrl Pts',(-27.1918041689889,1.39630935380484,0.659422735616693));
#56733=CARTESIAN_POINT('Ctrl Pts',(-27.2183187113946,1.53910864717388,0.125150820874972));
#56734=CARTESIAN_POINT('Ctrl Pts',(-27.2448332538003,1.42438548504866,-0.346479217847628));
#56735=CARTESIAN_POINT('Ctrl Pts',(-27.271347796206,1.30966232292344,-0.818109256570215));
#56736=CARTESIAN_POINT('Ctrl Pts',(-27.2978623386116,0.937416705303969,
-1.22709741927369));
#56737=CARTESIAN_POINT('Ctrl Pts',(-27.3243768810173,0.478635883963488,
-1.38557913848329));
#56738=CARTESIAN_POINT('Ctrl Pts',(-27.350891423423,0.0198550626230001,
-1.5440608576929));
#56739=CARTESIAN_POINT('Ctrl Pts',(-27.3774059658287,-0.525460962438503,
-1.45203613340863));
#56740=CARTESIAN_POINT('Ctrl Pts',(-27.4039205082344,-0.906826801844342,
-1.15177559006708));
#56741=CARTESIAN_POINT('Ctrl Pts',(-27.427895323542,-1.25166305903765,-0.880275861328805));
#56742=CARTESIAN_POINT('Ctrl Pts',(-27.4518701388495,-1.46245321697601,
-0.438521984001684));
#56743=CARTESIAN_POINT('Ctrl Pts',(-27.4758449541571,-1.46536634381812,
0.000808685770614676));
#56744=CARTESIAN_POINT('Ctrl Pts',(-27.5471550458428,-1.46502789863774,
0.00100125412595091));
#56745=CARTESIAN_POINT('Ctrl Pts',(-27.5239612140501,-1.46170129943445,
-0.424275850141513));
#56746=CARTESIAN_POINT('Ctrl Pts',(-27.5007673822574,-1.26606638633314,
-0.852218721532124));
#56747=CARTESIAN_POINT('Ctrl Pts',(-27.4775735504647,-0.94033990065008,
-1.12458112005112));
#56748=CARTESIAN_POINT('Ctrl Pts',(-27.451059008059,-0.567978455827939,
-1.43593822696579));
#56749=CARTESIAN_POINT('Ctrl Pts',(-27.4245444656533,-0.0256078086118435,
-1.54397615204525));
#56750=CARTESIAN_POINT('Ctrl Pts',(-27.3980299232476,0.437639581083625,
-1.39906876936017));
#56751=CARTESIAN_POINT('Ctrl Pts',(-27.3715153808419,0.9008869707791,-1.2541613866751));
#56752=CARTESIAN_POINT('Ctrl Pts',(-27.3450008384362,1.28501110295395,-0.856308696225503));
#56753=CARTESIAN_POINT('Ctrl Pts',(-27.3184862960305,1.41356845056175,-0.388260299163449));
#56754=CARTESIAN_POINT('Ctrl Pts',(-27.2919717536248,1.54212579816955,0.0797880978986051));
#56755=CARTESIAN_POINT('Ctrl Pts',(-27.2654572112192,1.41511636121028,0.618032201573119));
#56756=CARTESIAN_POINT('Ctrl Pts',(-27.2389426688135,1.09088063732047,0.979235037899136));
#56757=CARTESIAN_POINT('Ctrl Pts',(-27.2124281264078,0.766644913430665,
1.34043787422515));
#56758=CARTESIAN_POINT('Ctrl Pts',(-27.1859135840021,0.245182902610327,
1.52459944320268));
#56759=CARTESIAN_POINT('Ctrl Pts',(-27.1593990415964,-0.23397710544699,
1.44712699458503));
#56760=CARTESIAN_POINT('Ctrl Pts',(-27.1328844991907,-0.713137113504306,
1.36965454596737));
#56761=CARTESIAN_POINT('Ctrl Pts',(-27.106369956785,-1.1499951187986,1.03054807975452));
#56762=CARTESIAN_POINT('Ctrl Pts',(-27.0798554143794,-1.3438848241197,0.585572714383804));
#56763=CARTESIAN_POINT('Ctrl Pts',(-27.0689552915338,-1.42359284148406,
0.402643434611333));
#56764=CARTESIAN_POINT('Ctrl Pts',(-27.0580551686883,-1.46223847794561,
0.201821989221122));
#56765=CARTESIAN_POINT('Ctrl Pts',(-27.0471550458428,-1.46138800853787,
0.00068780616967229));
#56766=CARTESIAN_POINT('Origin',(-17.3,0.,0.));
#56767=CARTESIAN_POINT('',(-26.4758449541571,-1.46213373306659,-0.00114472513446554));
#56768=CARTESIAN_POINT('',(-26.5471550458428,-1.46250200525633,-0.00125517408728269));
#56769=CARTESIAN_POINT('',(-17.3,-1.4635,-1.79227059055215E-16));
#56770=CARTESIAN_POINT('Ctrl Pts',(-26.4758449541571,-1.46213373306659,
-0.00114472513446554));
#56771=CARTESIAN_POINT('Ctrl Pts',(-26.4935435057203,-1.45976174366936,
0.325019611661761));
#56772=CARTESIAN_POINT('Ctrl Pts',(-26.5112420572835,-1.35203577341253,
0.652605278604839));
#56773=CARTESIAN_POINT('Ctrl Pts',(-26.5289406088467,-1.15154649636273,
0.90711770191763));
#56774=CARTESIAN_POINT('Ctrl Pts',(-26.5554551512524,-0.851189632738311,
1.28840768582383));
#56775=CARTESIAN_POINT('Ctrl Pts',(-26.5819696936581,-0.342638369162514,
1.50569489065639));
#56776=CARTESIAN_POINT('Ctrl Pts',(-26.6084842360638,0.140509425568441,
1.45917064106431));
#56777=CARTESIAN_POINT('Ctrl Pts',(-26.6349987784695,0.623657220299389,
1.41264639147224));
#56778=CARTESIAN_POINT('Ctrl Pts',(-26.6615133208752,1.08140154618549,1.10231068745555));
#56779=CARTESIAN_POINT('Ctrl Pts',(-26.6880278632808,1.30348218633397,0.67071308942618));
#56780=CARTESIAN_POINT('Ctrl Pts',(-26.7145424056865,1.52556282648246,0.239115491396808));
#56781=CARTESIAN_POINT('Ctrl Pts',(-26.7410569480922,1.51197978089332,-0.313744000645244));
#56782=CARTESIAN_POINT('Ctrl Pts',(-26.7675714904979,1.26897228389482,-0.733914982218229));
#56783=CARTESIAN_POINT('Ctrl Pts',(-26.7940860329036,1.02596478689631,-1.15408596379121));
#56784=CARTESIAN_POINT('Ctrl Pts',(-26.8206005753093,0.553532838488442,
-1.44156843489514));
#56785=CARTESIAN_POINT('Ctrl Pts',(-26.847115117715,0.0686832661114671,
-1.4643102360408));
#56786=CARTESIAN_POINT('Ctrl Pts',(-26.8736296601207,-0.416166306265507,
-1.48705203718647));
#56787=CARTESIAN_POINT('Ctrl Pts',(-26.9001442025263,-0.913433502611594,
-1.24505316837387));
#56788=CARTESIAN_POINT('Ctrl Pts',(-26.926658744932,-1.19470367604941,-0.849473357352444));
#56789=CARTESIAN_POINT('Ctrl Pts',(-26.943054148007,-1.36862852815262,-0.604864555480574));
#56790=CARTESIAN_POINT('Ctrl Pts',(-26.9594495510821,-1.45996409858695,
-0.301532075271507));
#56791=CARTESIAN_POINT('Ctrl Pts',(-26.9758449541571,-1.46162142615836,
0.000882726340737661));
#56792=CARTESIAN_POINT('Ctrl Pts',(-27.0471550458428,-1.46138800853787,
0.00068780616967229));
#56793=CARTESIAN_POINT('Ctrl Pts',(-27.0315406262826,-1.46016971161189,
-0.287436792659947));
#56794=CARTESIAN_POINT('Ctrl Pts',(-27.0159262067225,-1.37790325039224,
-0.576203146234523));
#56795=CARTESIAN_POINT('Ctrl Pts',(-27.0003117871623,-1.2191927952091,-0.813935349054367));
#56796=CARTESIAN_POINT('Ctrl Pts',(-26.9737972447566,-0.949689655629521,
-1.21762378259322));
#56797=CARTESIAN_POINT('Ctrl Pts',(-26.9472827023509,-0.459761971122466,
-1.47415638514234));
#56798=CARTESIAN_POINT('Ctrl Pts',(-26.9207681599452,0.0255469418125742,
-1.46569750565868));
#56799=CARTESIAN_POINT('Ctrl Pts',(-26.8942536175395,0.510855854747614,
-1.45723862617501));
#56800=CARTESIAN_POINT('Ctrl Pts',(-26.8677390751339,0.991545996110626,
-1.18378826465857));
#56801=CARTESIAN_POINT('Ctrl Pts',(-26.8412245327282,1.24681722122356,-0.770953073273854));
#56802=CARTESIAN_POINT('Ctrl Pts',(-26.8147099903225,1.5020884463365,-0.358117881889143));
#56803=CARTESIAN_POINT('Ctrl Pts',(-26.7881954479168,1.53194075519934,0.194102139363843));
#56804=CARTESIAN_POINT('Ctrl Pts',(-26.7616809055111,1.32266179228677,0.632050320429307));
#56805=CARTESIAN_POINT('Ctrl Pts',(-26.7351663631054,1.1133828293742,1.06999850149476));
#56806=CARTESIAN_POINT('Ctrl Pts',(-26.7086518206997,0.664972594686232,
1.39367484237271));
#56807=CARTESIAN_POINT('Ctrl Pts',(-26.6821372782941,0.18340378492406,1.45440189631531));
#56808=CARTESIAN_POINT('Ctrl Pts',(-26.6556227358884,-0.298165024838112,
1.51512895025791));
#56809=CARTESIAN_POINT('Ctrl Pts',(-26.6291081934827,-0.812892409674494,
1.31290671726514));
#56810=CARTESIAN_POINT('Ctrl Pts',(-26.602593651077,-1.12434356208232,0.940623930555713));
#56811=CARTESIAN_POINT('Ctrl Pts',(-26.5841141159989,-1.34141208274397,
0.681158286733034));
#56812=CARTESIAN_POINT('Ctrl Pts',(-26.5656345809209,-1.45973894627015,
0.339085538839498));
#56813=CARTESIAN_POINT('Ctrl Pts',(-26.5471550458428,-1.46250200525633,
-0.00125517408728269));
#56814=CARTESIAN_POINT('Origin',(-17.3,0.,0.));
#56815=CARTESIAN_POINT('',(-25.9758449541571,-1.46577604770729,-0.000418285830775106));
#56816=CARTESIAN_POINT('',(-26.0471550458428,-1.46589951635168,-0.000156764579445036));
#56817=CARTESIAN_POINT('',(-17.3,-1.4635,-1.79227059055215E-16));
#56818=CARTESIAN_POINT('Ctrl Pts',(-25.9758449541571,-1.46577604770729,
-0.000418285830775106));
#56819=CARTESIAN_POINT('Ctrl Pts',(-26.0011229179528,-1.46402865658604,
0.462449158555644));
#56820=CARTESIAN_POINT('Ctrl Pts',(-26.0264008817486,-1.22637013755602,
0.926861111284242));
#56821=CARTESIAN_POINT('Ctrl Pts',(-26.0516788455444,-0.849171557970889,
1.19491820789161));
#56822=CARTESIAN_POINT('Ctrl Pts',(-26.0781933879501,-0.453520713046003,
1.47608845216313));
#56823=CARTESIAN_POINT('Ctrl Pts',(-26.1047079303558,0.0956565101240506,
1.54122288713929));
#56824=CARTESIAN_POINT('Ctrl Pts',(-26.1312224727614,0.54610111994442,1.36040267024623));
#56825=CARTESIAN_POINT('Ctrl Pts',(-26.1577370151671,0.996545729764802,
1.17958245335315));
#56826=CARTESIAN_POINT('Ctrl Pts',(-26.1842515575728,1.34825772623547,0.752807584590828));
#56827=CARTESIAN_POINT('Ctrl Pts',(-26.2107660999785,1.43968176835123,0.276112774595261));
#56828=CARTESIAN_POINT('Ctrl Pts',(-26.2372806423842,1.53110581046699,-0.200582035400292));
#56829=CARTESIAN_POINT('Ctrl Pts',(-26.2637951847899,1.36224189822785,-0.727196786629095));
#56830=CARTESIAN_POINT('Ctrl Pts',(-26.2903097271955,1.0106559582983,-1.06183633031355));
#56831=CARTESIAN_POINT('Ctrl Pts',(-26.3168242696012,0.659070018368756,
-1.39647587399801));
#56832=CARTESIAN_POINT('Ctrl Pts',(-26.3433388120069,0.1247620507488,-1.53914021013813));
#56833=CARTESIAN_POINT('Ctrl Pts',(-26.3698533544126,-0.346838994804863,
-1.42429792181986));
#56834=CARTESIAN_POINT('Ctrl Pts',(-26.3963678968183,-0.818440040358527,
-1.30945563350158));
#56835=CARTESIAN_POINT('Ctrl Pts',(-26.422882439224,-1.22733416384589,-0.937106720724912));
#56836=CARTESIAN_POINT('Ctrl Pts',(-26.4493969816297,-1.38569999375305,
-0.478285882846657));
#56837=CARTESIAN_POINT('Ctrl Pts',(-26.4582129724721,-1.43835606772408,
-0.325729589655548));
#56838=CARTESIAN_POINT('Ctrl Pts',(-26.4670289633146,-1.46331526686215,
-0.163613489658279));
#56839=CARTESIAN_POINT('Ctrl Pts',(-26.4758449541571,-1.46213373306659,
-0.00114472513446554));
#56840=CARTESIAN_POINT('Ctrl Pts',(-26.5471550458428,-1.46250200525633,
-0.00125517408728269));
#56841=CARTESIAN_POINT('Ctrl Pts',(-26.5391200385152,-1.46370339907424,
-0.149237258631324));
#56842=CARTESIAN_POINT('Ctrl Pts',(-26.5310850311876,-1.44305676186228,
-0.296891891566712));
#56843=CARTESIAN_POINT('Ctrl Pts',(-26.5230500238599,-1.39917926887205,
-0.437286173905273));
#56844=CARTESIAN_POINT('Ctrl Pts',(-26.4965354814543,-1.25438890327467,
-0.900570151230718));
#56845=CARTESIAN_POINT('Ctrl Pts',(-26.4700209390486,-0.856633252100626,
-1.2847947654555));
#56846=CARTESIAN_POINT('Ctrl Pts',(-26.4435063966429,-0.388617342494253,
-1.41347033412192));
#56847=CARTESIAN_POINT('Ctrl Pts',(-26.4169918542372,0.0793985671121137,
-1.54214590278835));
#56848=CARTESIAN_POINT('Ctrl Pts',(-26.3904773118315,0.617674735150821,
-1.41527242589641));
#56849=CARTESIAN_POINT('Ctrl Pts',(-26.3639627694258,0.978959459220186,
-1.09112794920365));
#56850=CARTESIAN_POINT('Ctrl Pts',(-26.3374482270201,1.34024418328956,-0.766983472510881));
#56851=CARTESIAN_POINT('Ctrl Pts',(-26.3109336846144,1.52453746338961,-0.245567996017281));
#56852=CARTESIAN_POINT('Ctrl Pts',(-26.2844191422087,1.44718604910436,0.233611565654946));
#56853=CARTESIAN_POINT('Ctrl Pts',(-26.2579045998031,1.36983463481912,0.71279112732716));
#56854=CARTESIAN_POINT('Ctrl Pts',(-26.2313900573974,1.0308385261486,1.14973477417799));
#56855=CARTESIAN_POINT('Ctrl Pts',(-26.2048755149917,0.585912149911522,
1.34373687041627));
#56856=CARTESIAN_POINT('Ctrl Pts',(-26.178360972586,0.140985773674437,1.53773896665454));
#56857=CARTESIAN_POINT('Ctrl Pts',(-26.1518464301803,-0.409870870129208,
1.48879951228024));
#56858=CARTESIAN_POINT('Ctrl Pts',(-26.1253318877746,-0.813627365057277,
1.21939834966265));
#56859=CARTESIAN_POINT('Ctrl Pts',(-26.099272940464,-1.21044617741552,0.954626263663422));
#56860=CARTESIAN_POINT('Ctrl Pts',(-26.0732139931534,-1.4651766057368,0.476903693889965));
#56861=CARTESIAN_POINT('Ctrl Pts',(-26.0471550458428,-1.46589951635168,
-0.000156764579445036));
#56862=CARTESIAN_POINT('Origin',(-17.3,0.,0.));
#56863=CARTESIAN_POINT('',(-25.4758449541571,-1.4634040497188,0.00135246395512149));
#56864=CARTESIAN_POINT('',(-25.5471550458428,-1.462974653714,0.00133299795035805));
#56865=CARTESIAN_POINT('',(-17.3,-1.4635,-1.79227059055215E-16));
#56866=CARTESIAN_POINT('Ctrl Pts',(-25.4758449541571,-1.4634040497188,0.00135246395512149));
#56867=CARTESIAN_POINT('Ctrl Pts',(-25.4821877877797,-1.46447728228524,
0.117986719967053));
#56868=CARTESIAN_POINT('Ctrl Pts',(-25.4885306214023,-1.45171144302068,
0.234388849588667));
#56869=CARTESIAN_POINT('Ctrl Pts',(-25.494873455025,-1.42421026771716,0.347198749632873));
#56870=CARTESIAN_POINT('Ctrl Pts',(-25.5213879974306,-1.30924886053307,
0.818770771928236));
#56871=CARTESIAN_POINT('Ctrl Pts',(-25.5479025398363,-0.93679667635601,
1.22757083011101));
#56872=CARTESIAN_POINT('Ctrl Pts',(-25.574417082242,-0.477935851213949,
1.38582076061156));
#56873=CARTESIAN_POINT('Ctrl Pts',(-25.6009316246477,-0.0190750260718746,
1.54407069111212));
#56874=CARTESIAN_POINT('Ctrl Pts',(-25.6274461670534,0.526194440035206,
1.45177049393048));
#56875=CARTESIAN_POINT('Ctrl Pts',(-25.6539607094591,0.907408544114477,
1.15131732918673));
#56876=CARTESIAN_POINT('Ctrl Pts',(-25.6804752518648,1.28862264819373,0.850864164442985));
#56877=CARTESIAN_POINT('Ctrl Pts',(-25.7069897942705,1.50578139024517,0.342258032137153));
#56878=CARTESIAN_POINT('Ctrl Pts',(-25.7335043366762,1.45913510299437,-0.140877995539519));
#56879=CARTESIAN_POINT('Ctrl Pts',(-25.7600188790818,1.41248881574355,-0.624014023216204));
#56880=CARTESIAN_POINT('Ctrl Pts',(-25.7865334214875,1.10203749919048,-1.08167994626373));
#56881=CARTESIAN_POINT('Ctrl Pts',(-25.8130479638932,0.670383819193945,
-1.30365156133859));
#56882=CARTESIAN_POINT('Ctrl Pts',(-25.8395625062989,0.238730139197424,
-1.52562317641345));
#56883=CARTESIAN_POINT('Ctrl Pts',(-25.8660770487046,-0.314125904242543,
-1.51190048351566));
#56884=CARTESIAN_POINT('Ctrl Pts',(-25.8925915911103,-0.734235490724634,
-1.26878686254941));
#56885=CARTESIAN_POINT('Ctrl Pts',(-25.919106133516,-1.15434507720673,-1.02567324158315));
#56886=CARTESIAN_POINT('Ctrl Pts',(-25.9456206759216,-1.44170820673095,
-0.553168692548412));
#56887=CARTESIAN_POINT('Ctrl Pts',(-25.9721352183273,-1.46432753815322,
-0.0683133912476058));
#56888=CARTESIAN_POINT('Ctrl Pts',(-25.9733717969372,-1.46538245288565,
-0.0457008307393826));
#56889=CARTESIAN_POINT('Ctrl Pts',(-25.9746083755472,-1.46586152874133,
-0.023061406359889));
#56890=CARTESIAN_POINT('Ctrl Pts',(-25.9758449541571,-1.46577604770729,
-0.000418285830775106));
#56891=CARTESIAN_POINT('Ctrl Pts',(-26.0471550458428,-1.46589951635168,
-0.000156764579445036));
#56892=CARTESIAN_POINT('Ctrl Pts',(-26.0466994507477,-1.46591215517881,
-0.00849733192252772));
#56893=CARTESIAN_POINT('Ctrl Pts',(-26.0462438556526,-1.46584715304275,
-0.0168376968819965));
#56894=CARTESIAN_POINT('Ctrl Pts',(-26.0457882605576,-1.46570391184755,
-0.025176717911968));
#56895=CARTESIAN_POINT('Ctrl Pts',(-26.0192737181519,-1.45736761765727,
-0.510487752008116));
#56896=CARTESIAN_POINT('Ctrl Pts',(-25.9927591757462,-1.18403868322423,
-0.991246949339548));
#56897=CARTESIAN_POINT('Ctrl Pts',(-25.9662446333405,-0.771267984412847,
-1.24662244506899));
#56898=CARTESIAN_POINT('Ctrl Pts',(-25.9397300909348,-0.358497285601448,
-1.50199794079844));
#56899=CARTESIAN_POINT('Ctrl Pts',(-25.9132155485291,0.193715177588312,
-1.53198973492588));
#56900=CARTESIAN_POINT('Ctrl Pts',(-25.8867010061235,0.631716206820391,
-1.32282140078338));
#56901=CARTESIAN_POINT('Ctrl Pts',(-25.8601864637178,1.06971723605247,-1.11365306664087));
#56902=CARTESIAN_POINT('Ctrl Pts',(-25.8336719213121,1.39350683132687,-0.665324604228429));
#56903=CARTESIAN_POINT('Ctrl Pts',(-25.8071573789064,1.45435552363656,-0.183771148981231));
#56904=CARTESIAN_POINT('Ctrl Pts',(-25.7806428365007,1.51520421594625,0.297782306265959));
#56905=CARTESIAN_POINT('Ctrl Pts',(-25.754128294095,1.31311200529122,0.812560754347889));
#56906=CARTESIAN_POINT('Ctrl Pts',(-25.7276137516893,0.940907900447105,
1.12410593237749));
#56907=CARTESIAN_POINT('Ctrl Pts',(-25.7010992092837,0.568703795602993,
1.43565111040708));
#56908=CARTESIAN_POINT('Ctrl Pts',(-25.674584666878,0.0263877965697636,
1.54396301838436));
#56909=CARTESIAN_POINT('Ctrl Pts',(-25.6480701244723,-0.436932738826931,
1.39928967911267));
#56910=CARTESIAN_POINT('Ctrl Pts',(-25.6215555820666,-0.900253274223638,
1.25461633984098));
#56911=CARTESIAN_POINT('Ctrl Pts',(-25.5950410396609,-1.28457834598382,
0.856957753320337));
#56912=CARTESIAN_POINT('Ctrl Pts',(-25.5685264972552,-1.41337212749903,
0.388974361030265));
#56913=CARTESIAN_POINT('Ctrl Pts',(-25.5614026801177,-1.44797590583016,
0.263238526745882));
#56914=CARTESIAN_POINT('Ctrl Pts',(-25.5542788629803,-1.46413372082814,
0.132426176049788));
#56915=CARTESIAN_POINT('Ctrl Pts',(-25.5471550458428,-1.462974653714,0.00133299795035805));
#56916=CARTESIAN_POINT('Origin',(-17.3,0.,0.));
#56917=CARTESIAN_POINT('',(-24.9758449541571,-1.46110128969025,-0.00020250645966946));
#56918=CARTESIAN_POINT('',(-25.0471550458428,-1.4611947376406,-0.000434366747377157));
#56919=CARTESIAN_POINT('',(-17.3,-1.4635,-1.79227059055215E-16));
#56920=CARTESIAN_POINT('Ctrl Pts',(-24.9758449541571,-1.46110128969025,
-0.00020250645966946));
#56921=CARTESIAN_POINT('Ctrl Pts',(-24.9897672000123,-1.4607849998905,0.256823176151405));
#56922=CARTESIAN_POINT('Ctrl Pts',(-25.0036894458674,-1.39631108339353,
0.513997221673354));
#56923=CARTESIAN_POINT('Ctrl Pts',(-25.0176116917226,-1.26860136025212,
0.734555952384895));
#56924=CARTESIAN_POINT('Ctrl Pts',(-25.0441262341283,-1.02538163082939,
1.15460411697203));
#56925=CARTESIAN_POINT('Ctrl Pts',(-25.070640776534,-0.55280451131479,1.44184788658205));
#56926=CARTESIAN_POINT('Ctrl Pts',(-25.0971553189397,-0.0679435120251727,
1.46434474683774));
#56927=CARTESIAN_POINT('Ctrl Pts',(-25.1236698613453,0.416917487264431,
1.48684160709344));
#56928=CARTESIAN_POINT('Ctrl Pts',(-25.150184403751,0.914062366329063,1.24459155799483));
#56929=CARTESIAN_POINT('Ctrl Pts',(-25.1766989461567,1.1951326634949,0.848869704410039));
#56930=CARTESIAN_POINT('Ctrl Pts',(-25.2032134885624,1.47620296066076,0.45314785082523));
#56931=CARTESIAN_POINT('Ctrl Pts',(-25.2297280309681,1.5411986759278,-0.0960458072457594));
#56932=CARTESIAN_POINT('Ctrl Pts',(-25.2562425733738,1.36026468621463,-0.546444729002872));
#56933=CARTESIAN_POINT('Ctrl Pts',(-25.2827571157795,1.17933069650146,-0.996843650759966));
#56934=CARTESIAN_POINT('Ctrl Pts',(-25.3092716581851,0.752467001808086,
-1.34844783620318));
#56935=CARTESIAN_POINT('Ctrl Pts',(-25.3357862005908,0.275749114061697,
-1.43975146623013));
#56936=CARTESIAN_POINT('Ctrl Pts',(-25.3623007429965,-0.200968773684707,
-1.53105509625708));
#56937=CARTESIAN_POINT('Ctrl Pts',(-25.3888152854022,-0.727540854484134,
-1.36205817086775));
#56938=CARTESIAN_POINT('Ctrl Pts',(-25.4153298278079,-1.06209157978827,
-1.01038771496909));
#56939=CARTESIAN_POINT('Ctrl Pts',(-25.435501536591,-1.31661076781507,-0.74284419430576));
#56940=CARTESIAN_POINT('Ctrl Pts',(-25.455673245374,-1.45999091671316,-0.369572013396846));
#56941=CARTESIAN_POINT('Ctrl Pts',(-25.4758449541571,-1.4634040497188,0.00135246395512149));
#56942=CARTESIAN_POINT('Ctrl Pts',(-25.5471550458428,-1.462974653714,0.00133299795035805));
#56943=CARTESIAN_POINT('Ctrl Pts',(-25.5277643205746,-1.45981972265052,
-0.355497020564954));
#56944=CARTESIAN_POINT('Ctrl Pts',(-25.5083735953064,-1.32836312994779,
-0.714407703616101));
#56945=CARTESIAN_POINT('Ctrl Pts',(-25.4889828700381,-1.09137519147001,
-0.978683818081121));
#56946=CARTESIAN_POINT('Ctrl Pts',(-25.4624683276325,-0.767321982655538,
-1.34005040684294));
#56947=CARTESIAN_POINT('Ctrl Pts',(-25.4359537852268,-0.24595307375636,
-1.52447538630709));
#56948=CARTESIAN_POINT('Ctrl Pts',(-25.4094392428211,0.23324601095786,-1.44724501128948));
#56949=CARTESIAN_POINT('Ctrl Pts',(-25.3829247004154,0.71244509567208,-1.37001463627187));
#56950=CARTESIAN_POINT('Ctrl Pts',(-25.3564101580097,1.14947435620134,-1.0311289067725));
#56951=CARTESIAN_POINT('Ctrl Pts',(-25.329895615604,1.34358883097895,-0.586251548056509));
#56952=CARTESIAN_POINT('Ctrl Pts',(-25.3033810731983,1.53770330575656,-0.141374189340514));
#56953=CARTESIAN_POINT('Ctrl Pts',(-25.2768665307927,1.48890299478252,0.409494798592106));
#56954=CARTESIAN_POINT('Ctrl Pts',(-25.250351988387,1.21960382631541,0.813319329148672));
#56955=CARTESIAN_POINT('Ctrl Pts',(-25.2238374459813,0.950304657848305,
1.21714385970524));
#56956=CARTESIAN_POINT('Ctrl Pts',(-25.1973229035756,0.460506631888131,
1.47392393288575));
#56957=CARTESIAN_POINT('Ctrl Pts',(-25.1708083611699,-0.024806492405043,
1.46571022452073));
#56958=CARTESIAN_POINT('Ctrl Pts',(-25.1442938187642,-0.510119616698223,
1.4574965161557));
#56959=CARTESIAN_POINT('Ctrl Pts',(-25.1177792763586,-0.990947839324403,
1.18428902624514));
#56960=CARTESIAN_POINT('Ctrl Pts',(-25.0912647339529,-1.24642758937672,
0.771582846342876));
#56961=CARTESIAN_POINT('Ctrl Pts',(-25.0765615045829,-1.38809993306417,
0.542723017925664));
#56962=CARTESIAN_POINT('Ctrl Pts',(-25.0618582752128,-1.46047569528562,
0.270966149981189));
#56963=CARTESIAN_POINT('Ctrl Pts',(-25.0471550458428,-1.4611947376406,-0.000434366747377157));
#56964=CARTESIAN_POINT('Origin',(-17.3,0.,0.));
#56965=CARTESIAN_POINT('',(-24.4758449541571,-1.46414968530619,-0.00128056012016223));
#56966=CARTESIAN_POINT('',(-24.5471550458428,-1.46457278513142,-0.00117677452095056));
#56967=CARTESIAN_POINT('',(-17.3,-1.4635,-1.79227059055215E-16));
#56968=CARTESIAN_POINT('Ctrl Pts',(-24.4758449541571,-1.46414968530619,
-0.00128056012016223));
#56969=CARTESIAN_POINT('Ctrl Pts',(-24.4973466122448,-1.46052449486356,
0.393583248871125));
#56970=CARTESIAN_POINT('Ctrl Pts',(-24.5188482703325,-1.29537096979211,
0.791118806776767));
#56971=CARTESIAN_POINT('Ctrl Pts',(-24.5403499284202,-1.01011940717455,
1.06234676149878));
#56972=CARTESIAN_POINT('Ctrl Pts',(-24.5668644708259,-0.658364457744287,
1.39680864707739));
#56973=CARTESIAN_POINT('Ctrl Pts',(-24.5933790132316,-0.123984486640841,
1.53920304146123));
#56974=CARTESIAN_POINT('Ctrl Pts',(-24.6198935556373,0.347558482308701,
1.42412252274616));
#56975=CARTESIAN_POINT('Ctrl Pts',(-24.646408098043,0.819101451258258,1.30904200403109));
#56976=CARTESIAN_POINT('Ctrl Pts',(-24.6729226404487,1.22780741805391,0.936486572217083));
#56977=CARTESIAN_POINT('Ctrl Pts',(-24.6994371828544,1.38594143905111,0.477585789087716));
#56978=CARTESIAN_POINT('Ctrl Pts',(-24.72595172526,1.54407546004832,0.0186850059583487));
#56979=CARTESIAN_POINT('Ctrl Pts',(-24.7524662676657,1.45163753524709,-0.526561128486383));
#56980=CARTESIAN_POINT('Ctrl Pts',(-24.7789808100714,1.15108808855372,-0.907699328416276));
#56981=CARTESIAN_POINT('Ctrl Pts',(-24.8054953524771,0.850538641860351,
-1.28883752834616));
#56982=CARTESIAN_POINT('Ctrl Pts',(-24.8320098948828,0.341877673274856,
-1.50586779376121));
#56983=CARTESIAN_POINT('Ctrl Pts',(-24.8585244372885,-0.141246556522215,
-1.45909947182782));
#56984=CARTESIAN_POINT('Ctrl Pts',(-24.8850389796942,-0.6243707863193,-1.41233114989443));
#56985=CARTESIAN_POINT('Ctrl Pts',(-24.9115535220998,-1.08195827732796,
-1.10176424061258));
#56986=CARTESIAN_POINT('Ctrl Pts',(-24.9380680645055,-1.30382085316685,
-0.670054506189522));
#56987=CARTESIAN_POINT('Ctrl Pts',(-24.950660361056,-1.40918791195588,-0.465026755137965));
#56988=CARTESIAN_POINT('Ctrl Pts',(-24.9632526576066,-1.46138736529873,
-0.232675316536856));
#56989=CARTESIAN_POINT('Ctrl Pts',(-24.9758449541571,-1.46110128969025,
-0.00020250645966946));
#56990=CARTESIAN_POINT('Ctrl Pts',(-25.0471550458428,-1.4611947376406,-0.000434366747377157));
#56991=CARTESIAN_POINT('Ctrl Pts',(-25.0353437328071,-1.46177235457949,
-0.218454257510994));
#56992=CARTESIAN_POINT('Ctrl Pts',(-25.0235324197715,-1.41610890745192,
-0.436244189947807));
#56993=CARTESIAN_POINT('Ctrl Pts',(-25.0117211067358,-1.32298092488054,
-0.631382052906385));
#56994=CARTESIAN_POINT('Ctrl Pts',(-24.9852065643301,-1.11392323285356,
-1.06943590235947));
#56995=CARTESIAN_POINT('Ctrl Pts',(-24.9586920219244,-0.665676571321139,
-1.3933387313717));
#56996=CARTESIAN_POINT('Ctrl Pts',(-24.9321774795187,-0.184138501313287,
-1.45430905816616));
#56997=CARTESIAN_POINT('Ctrl Pts',(-24.9056629371131,0.297399568694545,
-1.51527938496062));
#56998=CARTESIAN_POINT('Ctrl Pts',(-24.8791483947074,0.812229047177795,
-1.31331720953735));
#56999=CARTESIAN_POINT('Ctrl Pts',(-24.8526338523017,1.12386823095177,-0.941191810306153));
#57000=CARTESIAN_POINT('Ctrl Pts',(-24.826119309896,1.43550741472577,-0.569066411074926));
#57001=CARTESIAN_POINT('Ctrl Pts',(-24.7996047674903,1.54395630379045,-0.0267777880357327));
#57002=CARTESIAN_POINT('Ctrl Pts',(-24.7730902250846,1.39940000007497,0.436579275871188));
#57003=CARTESIAN_POINT('Ctrl Pts',(-24.7465756826789,1.2548436963595,0.899936339778083));
#57004=CARTESIAN_POINT('Ctrl Pts',(-24.7200611402733,0.857282199863888,
1.28436184455272));
#57005=CARTESIAN_POINT('Ctrl Pts',(-24.6935465978676,0.389331354748685,
1.41327383069934));
#57006=CARTESIAN_POINT('Ctrl Pts',(-24.6670320554619,-0.0786194903665382,
1.54218581684597));
#57007=CARTESIAN_POINT('Ctrl Pts',(-24.6405175130562,-0.616959684101348,
1.41558428436456));
#57008=CARTESIAN_POINT('Ctrl Pts',(-24.6140029706505,-0.978408114499494,
1.09162236410381));
#57009=CARTESIAN_POINT('Ctrl Pts',(-24.5917203290479,-1.28216692387813,
0.819366963591972));
#57010=CARTESIAN_POINT('Ctrl Pts',(-24.5694376874454,-1.4609940220446,0.407723665612911));
#57011=CARTESIAN_POINT('Ctrl Pts',(-24.5471550458428,-1.46457278513142,
-0.00117677452095056));
#57012=CARTESIAN_POINT('Origin',(-17.3,0.,0.));
#57013=CARTESIAN_POINT('',(-23.9758449541571,-1.46535571869621,0.000815875462887895));
#57014=CARTESIAN_POINT('',(-24.0471550458428,-1.46501532673864,0.00100720506673913));
#57015=CARTESIAN_POINT('',(-17.3,-1.4635,-1.79227059055215E-16));
#57016=CARTESIAN_POINT('Ctrl Pts',(-23.9758449541571,-1.46535571869621,
0.000815875462887895));
#57017=CARTESIAN_POINT('Ctrl Pts',(-23.9784114820717,-1.46566979594398,
0.0478475604868917));
#57018=CARTESIAN_POINT('Ctrl Pts',(-23.9809780099863,-1.46360259269125,
0.0948512818988251));
#57019=CARTESIAN_POINT('Ctrl Pts',(-23.9835445379008,-1.45906374756695,
0.141615108493016));
#57020=CARTESIAN_POINT('Ctrl Pts',(-24.0100590803065,-1.41217339393492,
0.624727509585923));
#57021=CARTESIAN_POINT('Ctrl Pts',(-24.0365736227122,-1.10149091173927,
1.08223653936045));
#57022=CARTESIAN_POINT('Ctrl Pts',(-24.0630881651179,-0.669725150433888,
1.30399006180796));
#57023=CARTESIAN_POINT('Ctrl Pts',(-24.0896027075236,-0.237959389128517,
1.52574358425545));
#57024=CARTESIAN_POINT('Ctrl Pts',(-24.1161172499293,0.314889651286583,
1.51174159937593));
#57025=CARTESIAN_POINT('Ctrl Pts',(-24.142631792335,0.734876367178585,1.26841577701478));
#57026=CARTESIAN_POINT('Ctrl Pts',(-24.1691463347406,1.1548630830706,1.02508995465363));
#57027=CARTESIAN_POINT('Ctrl Pts',(-24.1956608771463,1.44198747443951,0.552440294810826));
#57028=CARTESIAN_POINT('Ctrl Pts',(-24.222175419552,1.46436186209328,0.0675736284677887));
#57029=CARTESIAN_POINT('Ctrl Pts',(-24.2486899619577,1.48673624974706,-0.417293037875236));
#57030=CARTESIAN_POINT('Ctrl Pts',(-24.2752045043634,1.24436063368571,-0.914376710718497));
#57031=CARTESIAN_POINT('Ctrl Pts',(-24.3017190467691,0.848567796689088,
-1.19534704284565));
#57032=CARTESIAN_POINT('Ctrl Pts',(-24.3282335891748,0.452774959692452,
-1.47631737497281));
#57033=CARTESIAN_POINT('Ctrl Pts',(-24.3547481315804,-0.0964350982394741,
-1.54117436638384));
#57034=CARTESIAN_POINT('Ctrl Pts',(-24.3812626739861,-0.546788303196699,
-1.36012661539464));
#57035=CARTESIAN_POINT('Ctrl Pts',(-24.4077772163918,-0.997141508153911,
-1.17907886440544));
#57036=CARTESIAN_POINT('Ctrl Pts',(-24.4342917587975,-1.34863786013643,
-0.752126371016021));
#57037=CARTESIAN_POINT('Ctrl Pts',(-24.4608063012032,-1.43982107224915,
-0.275385435934625));
#57038=CARTESIAN_POINT('Ctrl Pts',(-24.4658191855211,-1.45706032484753,
-0.185251986877209));
#57039=CARTESIAN_POINT('Ctrl Pts',(-24.4708320698391,-1.46499486014087,
-0.093338883610889));
#57040=CARTESIAN_POINT('Ctrl Pts',(-24.4758449541571,-1.46414968530619,
-0.00128056012016223));
#57041=CARTESIAN_POINT('Ctrl Pts',(-24.5471550458428,-1.46457278513142,
-0.00117677452095056));
#57042=CARTESIAN_POINT('Ctrl Pts',(-24.5429231450397,-1.46525246084723,
-0.0788348068074314));
#57043=CARTESIAN_POINT('Ctrl Pts',(-24.5386912442366,-1.45961105333077,
-0.156393906155542));
#57044=CARTESIAN_POINT('Ctrl Pts',(-24.5344593434335,-1.44730388113662,
-0.232880441379075));
#57045=CARTESIAN_POINT('Ctrl Pts',(-24.5079448010278,-1.37019455031415,
-0.71209901856115));
#57046=CARTESIAN_POINT('Ctrl Pts',(-24.4814302586221,-1.03141922160774,
-1.14921386488522));
#57047=CARTESIAN_POINT('Ctrl Pts',(-24.4549157162164,-0.586590908797168,
-1.34344070581718));
#57048=CARTESIAN_POINT('Ctrl Pts',(-24.4284011738107,-0.141762595986587,
-1.53766754674914));
#57049=CARTESIAN_POINT('Ctrl Pts',(-24.401886631405,0.409118700928145,-1.48900638228895));
#57050=CARTESIAN_POINT('Ctrl Pts',(-24.3753720889993,0.813011241348171,
-1.21980922515431));
#57051=CARTESIAN_POINT('Ctrl Pts',(-24.3488575465936,1.2169037817682,-0.950612068019661));
#57052=CARTESIAN_POINT('Ctrl Pts',(-24.322343004188,1.4738075656935,-0.460878918210565));
#57053=CARTESIAN_POINT('Ctrl Pts',(-24.2958284617823,1.46571644367779,0.0244362653153989));
#57054=CARTESIAN_POINT('Ctrl Pts',(-24.2693139193766,1.45762532166208,0.509751448841349));
#57055=CARTESIAN_POINT('Ctrl Pts',(-24.2427993769709,1.18453929370534,0.9906486660842));
#57056=CARTESIAN_POINT('Ctrl Pts',(-24.2162848345652,0.771897659043956,
1.24623265415913));
#57057=CARTESIAN_POINT('Ctrl Pts',(-24.1897702921595,0.359256024382572,
1.50181664223405));
#57058=CARTESIAN_POINT('Ctrl Pts',(-24.1632557497538,-0.192941216983452,
1.5320874011411));
#57059=CARTESIAN_POINT('Ctrl Pts',(-24.1367412073481,-0.631047858708569,
1.32314036456809));
#57060=CARTESIAN_POINT('Ctrl Pts',(-24.1102266649425,-1.06915450043368,
1.11419332799508));
#57061=CARTESIAN_POINT('Ctrl Pts',(-24.0837121225368,-1.39317054251788,
0.666028495942013));
#57062=CARTESIAN_POINT('Ctrl Pts',(-24.0571975801311,-1.45426249990707,
0.184505841896889));
#57063=CARTESIAN_POINT('Ctrl Pts',(-24.0538500687017,-1.46197547577055,
0.12371269060351));
#57064=CARTESIAN_POINT('Ctrl Pts',(-24.0505025572722,-1.46549756189357,
0.0623878308737869));
#57065=CARTESIAN_POINT('Ctrl Pts',(-24.0471550458428,-1.46501532673864,
0.00100720506673913));
#57066=CARTESIAN_POINT('Origin',(-17.3,0.,0.));
#57067=CARTESIAN_POINT('',(-23.4758449541571,-1.4616124403278,0.000876453398841459));
#57068=CARTESIAN_POINT('',(-23.5471550458428,-1.46138107708475,0.000680708301427907));
#57069=CARTESIAN_POINT('',(-17.3,-1.4635,-1.79227059055215E-16));
#57070=CARTESIAN_POINT('Ctrl Pts',(-23.4758449541571,-1.4616124403278,0.000876453398841459));
#57071=CARTESIAN_POINT('Ctrl Pts',(-23.4859908943042,-1.46263037628344,
0.188022186505176));
#57072=CARTESIAN_POINT('Ctrl Pts',(-23.4961368344513,-1.4293109343094,0.374819137226617));
#57073=CARTESIAN_POINT('Ctrl Pts',(-23.5062827745985,-1.35998845779505,
0.547131842504017));
#57074=CARTESIAN_POINT('Ctrl Pts',(-23.5327973170041,-1.17882695708114,
0.997439301927659));
#57075=CARTESIAN_POINT('Ctrl Pts',(-23.5593118594098,-0.751785692236323,
1.3488277980231));
#57076=CARTESIAN_POINT('Ctrl Pts',(-23.5858264018155,-0.275021740237209,
1.43989058640388));
#57077=CARTESIAN_POINT('Ctrl Pts',(-23.6123409442212,0.201742211761891,
1.53095337478465));
#57078=CARTESIAN_POINT('Ctrl Pts',(-23.6388554866269,0.728228850915275,
1.36169045545076));
#57079=CARTESIAN_POINT('Ctrl Pts',(-23.6653700290326,1.06260187542882,1.00985103493177));
#57080=CARTESIAN_POINT('Ctrl Pts',(-23.6918845714383,1.39697489994238,0.658011614412757));
#57081=CARTESIAN_POINT('Ctrl Pts',(-23.718399113844,1.53923430981608,0.123595692708635));
#57082=CARTESIAN_POINT('Ctrl Pts',(-23.7449136562497,1.42403468691244,-0.34791819280944));
#57083=CARTESIAN_POINT('Ctrl Pts',(-23.7714281986553,1.30883506400881,-0.819432078327503));
#57084=CARTESIAN_POINT('Ctrl Pts',(-23.797942741061,0.936176408327837,-1.22804392765955));
#57085=CARTESIAN_POINT('Ctrl Pts',(-23.8244572834667,0.477235696490234,
-1.38606202906403));
#57086=CARTESIAN_POINT('Ctrl Pts',(-23.8509718258724,0.0182949846526319,
-1.54408013046851));
#57087=CARTESIAN_POINT('Ctrl Pts',(-23.8774863682781,-0.526927783341603,
-1.45150448394547));
#57088=CARTESIAN_POINT('Ctrl Pts',(-23.9040009106838,-0.90799005480451,
-1.15085877447831));
#57089=CARTESIAN_POINT('Ctrl Pts',(-23.9279489251749,-1.25216664512165,
-0.879314664953531));
#57090=CARTESIAN_POINT('Ctrl Pts',(-23.951896939666,-1.46242509540613,-0.438032059172249));
#57091=CARTESIAN_POINT('Ctrl Pts',(-23.9758449541571,-1.46535571869621,
0.000815875462887895));
#57092=CARTESIAN_POINT('Ctrl Pts',(-24.0471550458428,-1.46501532673864,
0.00100720506673913));
#57093=CARTESIAN_POINT('Ctrl Pts',(-24.0239880148665,-1.46167793506498,
-0.423788016516127));
#57094=CARTESIAN_POINT('Ctrl Pts',(-24.0008209838903,-1.26655073000452,
-0.85125419400408));
#57095=CARTESIAN_POINT('Ctrl Pts',(-23.977653952914,-0.941475660114631,
-1.12363045782044));
#57096=CARTESIAN_POINT('Ctrl Pts',(-23.9511394105083,-0.569428990238878,
-1.43536362745538));
#57097=CARTESIAN_POINT('Ctrl Pts',(-23.9246248681026,-0.0271677777932092,
-1.54394949068812));
#57098=CARTESIAN_POINT('Ctrl Pts',(-23.898110325697,0.436225785060499,-1.39951023175195));
#57099=CARTESIAN_POINT('Ctrl Pts',(-23.8715957832913,0.899619347914234,
-1.25507097281577));
#57100=CARTESIAN_POINT('Ctrl Pts',(-23.8450812408856,1.28414526117601,-0.85760659171064));
#57101=CARTESIAN_POINT('Ctrl Pts',(-23.8185666984799,1.41317544372912,-0.389688323626757));
#57102=CARTESIAN_POINT('Ctrl Pts',(-23.7920521560742,1.54220562628224,0.0782299444571254));
#57103=CARTESIAN_POINT('Ctrl Pts',(-23.7655376136685,1.4157400781267,0.61660209951974));
#57104=CARTESIAN_POINT('Ctrl Pts',(-23.7390230712628,1.0918694670893,0.978132348492866));
#57105=CARTESIAN_POINT('Ctrl Pts',(-23.7125085288571,0.767998856051899,
1.33966259746599));
#57106=CARTESIAN_POINT('Ctrl Pts',(-23.6859939864515,0.246723182132623,
1.5243509403496));
#57107=CARTESIAN_POINT('Ctrl Pts',(-23.6594794440458,-0.232514856941934,
1.44736265864203));
#57108=CARTESIAN_POINT('Ctrl Pts',(-23.6329649016401,-0.711752896016477,
1.37037437693446));
#57109=CARTESIAN_POINT('Ctrl Pts',(-23.6064503592344,-1.14895330024632,
1.03170947063572));
#57110=CARTESIAN_POINT('Ctrl Pts',(-23.5799358168287,-1.34329249494042,
0.586930232111769));
#57111=CARTESIAN_POINT('Ctrl Pts',(-23.5690088931667,-1.42338173474176,
0.403631998583174));
#57112=CARTESIAN_POINT('Ctrl Pts',(-23.5580819695048,-1.4622246078077,0.202311822928828));
#57113=CARTESIAN_POINT('Ctrl Pts',(-23.5471550458428,-1.46138107708475,
0.000680708301427907));
#57114=CARTESIAN_POINT('Origin',(-17.3,0.,0.));
#57115=CARTESIAN_POINT('',(-22.9758449541571,-1.46214569129651,-0.00114913864106017));
#57116=CARTESIAN_POINT('',(-23.0471550458428,-1.4625153155714,-0.00125827208086059));
#57117=CARTESIAN_POINT('',(-17.3,-1.4635,-1.79227059055215E-16));
#57118=CARTESIAN_POINT('Ctrl Pts',(-22.9758449541571,-1.46214569129651,
-0.00114913864106017));
#57119=CARTESIAN_POINT('Ctrl Pts',(-22.9935703065368,-1.45975965690007,
0.32550238069992));
#57120=CARTESIAN_POINT('Ctrl Pts',(-23.0112956589164,-1.35167970161975,
0.653585897788354));
#57121=CARTESIAN_POINT('Ctrl Pts',(-23.0290210112961,-1.15062938697513,
0.908280723260628));
#57122=CARTESIAN_POINT('Ctrl Pts',(-23.0555355537018,-0.849887433916146,
1.28926704194381));
#57123=CARTESIAN_POINT('Ctrl Pts',(-23.0820500961075,-0.341116890136462,
1.506040312553));
#57124=CARTESIAN_POINT('Ctrl Pts',(-23.1085646385132,0.141983651428446,
1.45902793021404));
#57125=CARTESIAN_POINT('Ctrl Pts',(-23.1350791809189,0.625084192993341,
1.41201554787508));
#57126=CARTESIAN_POINT('Ctrl Pts',(-23.1615937233246,1.08251473234346,1.10121751258798));
#57127=CARTESIAN_POINT('Ctrl Pts',(-23.1881082657302,1.30415918725112,0.669395751948055));
#57128=CARTESIAN_POINT('Ctrl Pts',(-23.2146228081359,1.52580364215879,0.237573991308118));
#57129=CARTESIAN_POINT('Ctrl Pts',(-23.2411373505416,1.51166201262399,-0.315271494684653));
#57130=CARTESIAN_POINT('Ctrl Pts',(-23.2676518929473,1.26823011284921,-0.735196735085295));
#57131=CARTESIAN_POINT('Ctrl Pts',(-23.294166435353,1.02479821307445,-1.15512197548593));
#57132=CARTESIAN_POINT('Ctrl Pts',(-23.3206809777587,0.552076043059725,
-1.44212697029443));
#57133=CARTESIAN_POINT('Ctrl Pts',(-23.3471955201643,0.0672037405990306,
-1.46437888391874));
#57134=CARTESIAN_POINT('Ctrl Pts',(-23.37371006257,-0.417668561861677,-1.48663079754305));
#57135=CARTESIAN_POINT('Ctrl Pts',(-23.4002246049757,-0.914690996768357,
-1.24412962998315));
#57136=CARTESIAN_POINT('Ctrl Pts',(-23.4267391473814,-1.19556134593018,
-0.848265834827282));
#57137=CARTESIAN_POINT('Ctrl Pts',(-23.44310774964,-1.36895506177522,-0.603881567796481));
#57138=CARTESIAN_POINT('Ctrl Pts',(-23.4594763518985,-1.45997018849692,
-0.301048654100674));
#57139=CARTESIAN_POINT('Ctrl Pts',(-23.4758449541571,-1.4616124403278,0.000876453398841459));
#57140=CARTESIAN_POINT('Ctrl Pts',(-23.5471550458428,-1.46138107708475,
0.000680708301427907));
#57141=CARTESIAN_POINT('Ctrl Pts',(-23.5315674270991,-1.46017775255219,
-0.286952759169412));
#57142=CARTESIAN_POINT('Ctrl Pts',(-23.5159798083554,-1.37821272310039,
-0.575218986457016));
#57143=CARTESIAN_POINT('Ctrl Pts',(-23.5003921896117,-1.2200145461662,-0.812703101675466));
#57144=CARTESIAN_POINT('Ctrl Pts',(-23.473877647206,-0.950919417539503,
-1.21666362618954));
#57145=CARTESIAN_POINT('Ctrl Pts',(-23.4473631048003,-0.461251175127714,
-1.47369110446852));
#57146=CARTESIAN_POINT('Ctrl Pts',(-23.4208485623946,0.0240660366666584,
-1.46572256931836));
#57147=CARTESIAN_POINT('Ctrl Pts',(-23.3943340199889,0.509383248461031,
-1.45775403416819));
#57148=CARTESIAN_POINT('Ctrl Pts',(-23.3678194775832,0.990349429638006,
-1.1847894855889));
#57149=CARTESIAN_POINT('Ctrl Pts',(-23.3413049351775,1.24603763942864,-0.772212422496003));
#57150=CARTESIAN_POINT('Ctrl Pts',(-23.3147903927719,1.50172584921927,-0.3596353594031));
#57151=CARTESIAN_POINT('Ctrl Pts',(-23.2882758503662,1.53213608762356,0.192554218203404));
#57152=CARTESIAN_POINT('Ctrl Pts',(-23.2617613079605,1.32329971983588,0.630713624248227));
#57153=CARTESIAN_POINT('Ctrl Pts',(-23.2352467655548,1.11446335204819,1.06887303029306));
#57154=CARTESIAN_POINT('Ctrl Pts',(-23.2087322231491,0.666380378068528,
1.39300226477619));
#57155=CARTESIAN_POINT('Ctrl Pts',(-23.1822176807434,0.184873170708501,
1.45421584886227));
#57156=CARTESIAN_POINT('Ctrl Pts',(-23.1557031383377,-0.296634036651499,
1.51542943294835));
#57157=CARTESIAN_POINT('Ctrl Pts',(-23.1291885959321,-0.811565477391885,
1.31372736663739));
#57158=CARTESIAN_POINT('Ctrl Pts',(-23.1026740535264,-1.12339261299846,
0.941759449854651));
#57159=CARTESIAN_POINT('Ctrl Pts',(-23.0841677176319,-1.34103837222996,
0.682137273290514));
#57160=CARTESIAN_POINT('Ctrl Pts',(-23.0656613817373,-1.45973961344624,
0.339568196618657));
#57161=CARTESIAN_POINT('Ctrl Pts',(-23.0471550458428,-1.4625153155714,-0.00125827208086059));
#57162=CARTESIAN_POINT('Origin',(-17.3,0.,0.));
#57163=CARTESIAN_POINT('',(-22.4758449541571,-1.46578197197304,-0.000409560824215643));
#57164=CARTESIAN_POINT('',(-22.5471550458428,-1.46590183802103,-0.000147589276300086));
#57165=CARTESIAN_POINT('',(-17.3,-1.4635,-1.79227059055215E-16));
#57166=CARTESIAN_POINT('Ctrl Pts',(-22.4758449541571,-1.46578197197304,
-0.000409560824215643));
#57167=CARTESIAN_POINT('Ctrl Pts',(-22.5011497187693,-1.46406545630175,
0.462943637033072));
#57168=CARTESIAN_POINT('Ctrl Pts',(-22.5264544833815,-1.225833251475,0.927815920084082));
#57169=CARTESIAN_POINT('Ctrl Pts',(-22.5517592479938,-0.847963818843918,
1.1957755727348));
#57170=CARTESIAN_POINT('Ctrl Pts',(-22.5782737903995,-0.452029090785964,
1.47654592101102));
#57171=CARTESIAN_POINT('Ctrl Pts',(-22.6047883328051,0.0972136617436899,
1.54112545230473));
#57172=CARTESIAN_POINT('Ctrl Pts',(-22.6313028752108,0.547475346902943,
1.35985021342467));
#57173=CARTESIAN_POINT('Ctrl Pts',(-22.6578174176165,0.997737032062196,
1.1785749745446));
#57174=CARTESIAN_POINT('Ctrl Pts',(-22.6843319600222,1.34901764985106,0.751444965490751));
#57175=CARTESIAN_POINT('Ctrl Pts',(-22.7108465024279,1.43996000868985,0.274658026992733));
#57176=CARTESIAN_POINT('Ctrl Pts',(-22.7373610448335,1.53090236752864,-0.202128911505298));
#57177=CARTESIAN_POINT('Ctrl Pts',(-22.7638755872392,1.36150646741735,-0.728572779447481));
#57178=CARTESIAN_POINT('Ctrl Pts',(-22.7903901296449,1.00958259825787,-1.06285692156211));
#57179=CARTESIAN_POINT('Ctrl Pts',(-22.8169046720506,0.657658729098401,
-1.39714106367674));
#57180=CARTESIAN_POINT('Ctrl Pts',(-22.8434192144563,0.123206890890731,
-1.53926547996378));
#57181=CARTESIAN_POINT('Ctrl Pts',(-22.869933756862,-0.348277881112059,
-1.42394676022164));
#57182=CARTESIAN_POINT('Ctrl Pts',(-22.8964482992677,-0.819762653114848,
-1.3086280404795));
#57183=CARTESIAN_POINT('Ctrl Pts',(-22.9229628416734,-1.22828035891277,
-0.935866184708164));
#57184=CARTESIAN_POINT('Ctrl Pts',(-22.9494773840791,-1.38618253064258,
-0.47688557344392));
#57185=CARTESIAN_POINT('Ctrl Pts',(-22.9582665741051,-1.43852483290143,
-0.324740092336465));
#57186=CARTESIAN_POINT('Ctrl Pts',(-22.9670557641311,-1.46332881641976,
-0.163120659109465));
#57187=CARTESIAN_POINT('Ctrl Pts',(-22.9758449541571,-1.46214569129651,
-0.00114913864106017));
#57188=CARTESIAN_POINT('Ctrl Pts',(-23.0471550458428,-1.4625153155714,-0.00125827208086059));
#57189=CARTESIAN_POINT('Ctrl Pts',(-23.0391468393317,-1.4637164391195,-0.148743369151091));
#57190=CARTESIAN_POINT('Ctrl Pts',(-23.0311386328205,-1.44321011457532,
-0.295902157002481));
#57191=CARTESIAN_POINT('Ctrl Pts',(-23.0231304263093,-1.39962037413654,
-0.435872266417514));
#57192=CARTESIAN_POINT('Ctrl Pts',(-22.9966158839036,-1.25529816919524,
-0.899302298652362));
#57193=CARTESIAN_POINT('Ctrl Pts',(-22.9701013414979,-0.857930928839858,
-1.28392859586752));
#57194=CARTESIAN_POINT('Ctrl Pts',(-22.9435867990922,-0.390045267641704,
-1.41307696659466));
#57195=CARTESIAN_POINT('Ctrl Pts',(-22.9170722566866,0.0778403935564494,
-1.5422253373218));
#57196=CARTESIAN_POINT('Ctrl Pts',(-22.8905577142809,0.616244475597355,
-1.41589578156095));
#57197=CARTESIAN_POINT('Ctrl Pts',(-22.8640431718752,0.977856520078891,
-1.09211650041067));
#57198=CARTESIAN_POINT('Ctrl Pts',(-22.8375286294695,1.33946856456042,-0.768337219260394));
#57199=CARTESIAN_POINT('Ctrl Pts',(-22.8110140870638,1.52428857148255,-0.247108212720685));
#57200=CARTESIAN_POINT('Ctrl Pts',(-22.7844995446581,1.44742134380195,0.232149257669704));
#57201=CARTESIAN_POINT('Ctrl Pts',(-22.7579850022524,1.37055411612135,0.711406728060106));
#57202=CARTESIAN_POINT('Ctrl Pts',(-22.7314704598468,1.03199965383798,1.14869266230121));
#57203=CARTESIAN_POINT('Ctrl Pts',(-22.7049559174411,0.587269517978703,
1.34314419835813));
#57204=CARTESIAN_POINT('Ctrl Pts',(-22.6784413750354,0.142539382119435,
1.53759573441505));
#57205=CARTESIAN_POINT('Ctrl Pts',(-22.6519268326297,-0.408366427315716,
1.48921287228782));
#57206=CARTESIAN_POINT('Ctrl Pts',(-22.625412290224,-0.812394910150128,
1.22021978933805));
#57207=CARTESIAN_POINT('Ctrl Pts',(-22.599326542097,-1.2098894276161,0.95557687367356));
#57208=CARTESIAN_POINT('Ctrl Pts',(-22.5732407939699,-1.46521881735637,
0.477401475176739));
#57209=CARTESIAN_POINT('Ctrl Pts',(-22.5471550458428,-1.46590183802103,
-0.000147589276300086));
#57210=CARTESIAN_POINT('Origin',(-17.3,0.,0.));
#57211=CARTESIAN_POINT('',(-21.9758449541571,-1.46338908451446,0.00135254369621918));
#57212=CARTESIAN_POINT('',(-22.0471550458428,-1.46296023813343,0.0013315397042942));
#57213=CARTESIAN_POINT('',(-17.3,-1.4635,-1.79227059055215E-16));
#57214=CARTESIAN_POINT('Ctrl Pts',(-21.9758449541571,-1.46338908451446,
0.00135254369621918));
#57215=CARTESIAN_POINT('Ctrl Pts',(-21.9822145885962,-1.46446593650969,
0.118482680034951));
#57216=CARTESIAN_POINT('Ctrl Pts',(-21.9885842230352,-1.45159056750017,
0.235378945131374));
#57217=CARTESIAN_POINT('Ctrl Pts',(-21.9949538574743,-1.42385874267934,
0.348637547193684));
#57218=CARTESIAN_POINT('Ctrl Pts',(-22.02146839988,-1.3084209334563,0.820093175599227));
#57219=CARTESIAN_POINT('Ctrl Pts',(-22.0479829422857,-0.935555901377785,
1.22851671179854));
#57220=CARTESIAN_POINT('Ctrl Pts',(-22.0744974846914,-0.476535419971068,
1.3863029437791));
#57221=CARTESIAN_POINT('Ctrl Pts',(-22.1010120270971,-0.017514938564339,
1.54408917575967));
#57222=CARTESIAN_POINT('Ctrl Pts',(-22.1275265695028,0.527660992170594,
1.45123810352149));
#57223=CARTESIAN_POINT('Ctrl Pts',(-22.1540411119085,0.908571333766114,
1.15039992605879));
#57224=CARTESIAN_POINT('Ctrl Pts',(-22.1805556543141,1.28948167536163,0.849561748596095));
#57225=CARTESIAN_POINT('Ctrl Pts',(-22.2070701967198,1.50612642781774,0.340736465908889));
#57226=CARTESIAN_POINT('Ctrl Pts',(-22.2335847391255,1.45899201977136,-0.142352185304953));
#57227=CARTESIAN_POINT('Ctrl Pts',(-22.2600992815312,1.41185761172498,-0.625440836518782));
#57228=CARTESIAN_POINT('Ctrl Pts',(-22.2866138239369,1.10094404317614,-1.08279285625925));
#57229=CARTESIAN_POINT('Ctrl Pts',(-22.3131283663426,0.669066310753002,
-1.30432822948558));
#57230=CARTESIAN_POINT('Ctrl Pts',(-22.3396429087483,0.237188578329877,
-1.5258636027119));
#57231=CARTESIAN_POINT('Ctrl Pts',(-22.3661574511539,-0.315653317967536,
-1.51158232942409));
#57232=CARTESIAN_POINT('Ctrl Pts',(-22.3926719935596,-0.735517056084479,
-1.26804436776732));
#57233=CARTESIAN_POINT('Ctrl Pts',(-22.4191865359653,-1.15538079420146,
-1.02450640611054));
#57234=CARTESIAN_POINT('Ctrl Pts',(-22.445701078371,-1.44226637413794,-0.551711756084745));
#57235=CARTESIAN_POINT('Ctrl Pts',(-22.4722156207767,-1.46439581231304,
-0.0668338484424606));
#57236=CARTESIAN_POINT('Ctrl Pts',(-22.4734253985702,-1.46540551115968,
-0.0447103466963747));
#57237=CARTESIAN_POINT('Ctrl Pts',(-22.4746351763636,-1.46586403567025,
-0.0225616897963809));
#57238=CARTESIAN_POINT('Ctrl Pts',(-22.4758449541571,-1.46578197197304,
-0.000409560824215643));
#57239=CARTESIAN_POINT('Ctrl Pts',(-22.5471550458428,-1.46590183802103,
-0.000147589276300086));
#57240=CARTESIAN_POINT('Ctrl Pts',(-22.5467262515642,-1.46591306542964,
-0.00799748131699719));
#57241=CARTESIAN_POINT('Ctrl Pts',(-22.5462974572856,-1.46585548643462,
-0.0158472041198875));
#57242=CARTESIAN_POINT('Ctrl Pts',(-22.5458686630069,-1.46572860144202,
-0.023695806482401));
#57243=CARTESIAN_POINT('Ctrl Pts',(-22.5193541206012,-1.45788265366583,
-0.509015015580697));
#57244=CARTESIAN_POINT('Ctrl Pts',(-22.4928395781956,-1.18503960187983,
-0.990050130004957));
#57245=CARTESIAN_POINT('Ctrl Pts',(-22.4663250357899,-0.772527136678897,
-1.24584254519772));
#57246=CARTESIAN_POINT('Ctrl Pts',(-22.4398104933842,-0.360014671477961,
-1.50163496039049));
#57247=CARTESIAN_POINT('Ctrl Pts',(-22.4132959509785,0.1921672071379,-1.53218467635176));
#57248=CARTESIAN_POINT('Ctrl Pts',(-22.3867814085728,0.630379349546724,
-1.32345899067372));
#57249=CARTESIAN_POINT('Ctrl Pts',(-22.3602668661672,1.06859149195557,-1.11473330499566));
#57250=CARTESIAN_POINT('Ctrl Pts',(-22.3337523237614,1.39283389815735,-0.666732217678252));
#57251=CARTESIAN_POINT('Ctrl Pts',(-22.3072377813558,1.45416910503474,-0.185240487724726));
#57252=CARTESIAN_POINT('Ctrl Pts',(-22.2807232389501,1.51550431191213,0.296251242228773));
#57253=CARTESIAN_POINT('Ctrl Pts',(-22.2542086965444,1.31393231946513,0.811233614818408));
#57254=CARTESIAN_POINT('Ctrl Pts',(-22.2276941541387,0.942043179507886,
1.12315469650121));
#57255=CARTESIAN_POINT('Ctrl Pts',(-22.201179611733,0.570154039550644,1.435075778184));
#57256=CARTESIAN_POINT('Ctrl Pts',(-22.1746650693273,0.0279477520831708,
1.54393556896));
#57257=CARTESIAN_POINT('Ctrl Pts',(-22.1481505269216,-0.43551871996475,
1.39973042722172));
#57258=CARTESIAN_POINT('Ctrl Pts',(-22.121635984516,-0.898985192012657,
1.25552528548345));
#57259=CARTESIAN_POINT('Ctrl Pts',(-22.0951214421103,-1.283711848641,0.858255211230917));
#57260=CARTESIAN_POINT('Ctrl Pts',(-22.0686068997046,-1.41297839930219,
0.390402186770835));
#57261=CARTESIAN_POINT('Ctrl Pts',(-22.0614562817507,-1.44783986150876,
0.264228474801143));
#57262=CARTESIAN_POINT('Ctrl Pts',(-22.0543056637967,-1.46412148390715,
0.132921202336442));
#57263=CARTESIAN_POINT('Ctrl Pts',(-22.0471550458428,-1.46296023813343,
0.0013315397042942));
#57264=CARTESIAN_POINT('Origin',(-17.3,0.,0.));
#57265=CARTESIAN_POINT('',(-21.4758449541571,-1.46110336159793,-0.000210604951717125));
#57266=CARTESIAN_POINT('',(-21.5471550458428,-1.46119914789583,-0.000442129891295945));
#57267=CARTESIAN_POINT('',(-17.3,-1.4635,-1.79227059055215E-16));
#57268=CARTESIAN_POINT('Ctrl Pts',(-21.4758449541571,-1.46110336159793,
-0.000210604951717125));
#57269=CARTESIAN_POINT('Ctrl Pts',(-21.4897940008287,-1.46077376388658,
0.25730895082503));
#57270=CARTESIAN_POINT('Ctrl Pts',(-21.5037430475004,-1.39603731955723,
0.514983410928407));
#57271=CARTESIAN_POINT('Ctrl Pts',(-21.517692094172,-1.26785854178086,0.735837330155876));
#57272=CARTESIAN_POINT('Ctrl Pts',(-21.5442066365777,-1.0242145337804,1.15563953920073));
#57273=CARTESIAN_POINT('Ctrl Pts',(-21.5707211789834,-0.551347433909141,
1.44240568596109));
#57274=CARTESIAN_POINT('Ctrl Pts',(-21.597235721389,-0.0664639520217993,
1.4644126472751));
#57275=CARTESIAN_POINT('Ctrl Pts',(-21.6237502637947,0.418419529865584,
1.4864196085891));
#57276=CARTESIAN_POINT('Ctrl Pts',(-21.6502648062004,0.915319393769039,
1.24366738445671));
#57277=CARTESIAN_POINT('Ctrl Pts',(-21.6767793486061,1.19598972324583,0.847661748758301));
#57278=CARTESIAN_POINT('Ctrl Pts',(-21.7032938910118,1.47666005272259,0.451656113059926));
#57279=CARTESIAN_POINT('Ctrl Pts',(-21.7298084334175,1.54110084777271,-0.097602934204468));
#57280=CARTESIAN_POINT('Ctrl Pts',(-21.7563229758231,1.35971188229233,-0.547818816371488));
#57281=CARTESIAN_POINT('Ctrl Pts',(-21.7828375182288,1.17832291681194,-0.998034698538546));
#57282=CARTESIAN_POINT('Ctrl Pts',(-21.8093520606345,0.751104190801025,
-1.34920741560824));
#57283=CARTESIAN_POINT('Ctrl Pts',(-21.8358666030402,0.274294296224285,
-1.44002933910266));
#57284=CARTESIAN_POINT('Ctrl Pts',(-21.8623811454459,-0.202515598352415,
-1.53085126259707));
#57285=CARTESIAN_POINT('Ctrl Pts',(-21.8888956878516,-0.728916661494918,
-1.36132239251625));
#57286=CARTESIAN_POINT('Ctrl Pts',(-21.9154102302573,-1.06311189988241,
-1.00931409716997));
#57287=CARTESIAN_POINT('Ctrl Pts',(-21.9355551382239,-1.3170228374044,-0.741869364210416));
#57288=CARTESIAN_POINT('Ctrl Pts',(-21.9557000461905,-1.45998338132298,
-0.369088780563025));
#57289=CARTESIAN_POINT('Ctrl Pts',(-21.9758449541571,-1.46338908451446,
0.00135254369621918));
#57290=CARTESIAN_POINT('Ctrl Pts',(-22.0471550458428,-1.46296023813343,
0.0013315397042942));
#57291=CARTESIAN_POINT('Ctrl Pts',(-22.0277911213911,-1.45981557629061,
-0.355014205832619));
#57292=CARTESIAN_POINT('Ctrl Pts',(-22.0084271969393,-1.32875708300604,
-0.713430803933623));
#57293=CARTESIAN_POINT('Ctrl Pts',(-21.9890632724875,-1.09236346405217,
-0.97758062927514));
#57294=CARTESIAN_POINT('Ctrl Pts',(-21.9625487300818,-0.768675533446972,
-1.33927444619329));
#57295=CARTESIAN_POINT('Ctrl Pts',(-21.9360341876762,-0.24749322754258,
-1.52422610536196));
#57296=CARTESIAN_POINT('Ctrl Pts',(-21.9095196452705,0.23178364358579,-1.44747993661264));
#57297=CARTESIAN_POINT('Ctrl Pts',(-21.8830051028648,0.711060514714174,
-1.37073376786332));
#57298=CARTESIAN_POINT('Ctrl Pts',(-21.8564905604591,1.14843195106653,-1.03228977119599));
#57299=CARTESIAN_POINT('Ctrl Pts',(-21.8299760180534,1.34299581607976,-0.587608766376321));
#57300=CARTESIAN_POINT('Ctrl Pts',(-21.8034614756477,1.53755968109297,-0.142927761556679));
#57301=CARTESIAN_POINT('Ctrl Pts',(-21.7769469332421,1.48931597476708,0.40799025141529));
#57302=CARTESIAN_POINT('Ctrl Pts',(-21.7504323908364,1.22042495465668,0.812086666791963));
#57303=CARTESIAN_POINT('Ctrl Pts',(-21.7239178484307,0.95153393454626,1.21618308216867));
#57304=CARTESIAN_POINT('Ctrl Pts',(-21.697403306025,0.461995600651293,1.47345789995005));
#57305=CARTESIAN_POINT('Ctrl Pts',(-21.6708887636193,-0.0233255747863311,
1.46573454004841));
#57306=CARTESIAN_POINT('Ctrl Pts',(-21.6443742212136,-0.508646750223927,
1.45801118014677));
#57307=CARTESIAN_POINT('Ctrl Pts',(-21.6178596788079,-0.98975076720418,
1.18528964256214));
#57308=CARTESIAN_POINT('Ctrl Pts',(-21.5913451364022,-1.24564737147885,
0.772841801572525));
#57309=CARTESIAN_POINT('Ctrl Pts',(-21.5766151062158,-1.38780953471398,
0.543708330016934));
#57310=CARTESIAN_POINT('Ctrl Pts',(-21.5618850760293,-1.46046579618679,
0.271451043834622));
#57311=CARTESIAN_POINT('Ctrl Pts',(-21.5471550458428,-1.46119914789583,
-0.000442129891295945));
#57312=CARTESIAN_POINT('Origin',(-17.3,0.,0.));
#57313=CARTESIAN_POINT('',(-20.9758449541571,-1.46416452657485,-0.00127774293595062));
#57314=CARTESIAN_POINT('',(-21.0471550458428,-1.46458686986414,-0.00117242835359658));
#57315=CARTESIAN_POINT('',(-17.3,-1.4635,-1.79227059055215E-16));
#57316=CARTESIAN_POINT('Ctrl Pts',(-20.9758449541571,-1.46416452657485,
-0.00127774293595062));
#57317=CARTESIAN_POINT('Ctrl Pts',(-20.9973734130613,-1.46053861299378,
0.394067914350929));
#57318=CARTESIAN_POINT('Ctrl Pts',(-21.0189018719655,-1.29492688262452,
0.792089489186256));
#57319=CARTESIAN_POINT('Ctrl Pts',(-21.0404303308696,-1.00904553168518,
1.06336681037344));
#57320=CARTESIAN_POINT('Ctrl Pts',(-21.0669448732753,-0.656952832611104,
1.39747312371126));
#57321=CARTESIAN_POINT('Ctrl Pts',(-21.093459415681,-0.12242926369691,1.53932752562985));
#57322=CARTESIAN_POINT('Ctrl Pts',(-21.1199739580867,0.348997191031295,
1.42377063429117));
#57323=CARTESIAN_POINT('Ctrl Pts',(-21.1464885004924,0.820423645759539,
1.30821374295248));
#57324=CARTESIAN_POINT('Ctrl Pts',(-21.1730030428981,1.2287529863018,0.935245558356483));
#57325=CARTESIAN_POINT('Ctrl Pts',(-21.1995175853037,1.38642326846593,0.476185236093947));
#57326=CARTESIAN_POINT('Ctrl Pts',(-21.2260321277094,1.54409355063006,0.0171249138314507));
#57327=CARTESIAN_POINT('Ctrl Pts',(-21.2525466701151,1.45110477441612,-0.528027546097545));
#57328=CARTESIAN_POINT('Ctrl Pts',(-21.2790612125208,1.15017039174401,-0.908861886302333));
#57329=CARTESIAN_POINT('Ctrl Pts',(-21.3055757549265,0.849236009071873,
-1.28969622650715));
#57330=CARTESIAN_POINT('Ctrl Pts',(-21.3320902973322,0.340356019941503,
-1.50621244698771));
#57331=CARTESIAN_POINT('Ctrl Pts',(-21.3586048397379,-0.14272071009898,
-1.45895601624122));
#57332=CARTESIAN_POINT('Ctrl Pts',(-21.3851193821435,-0.625797440139435,
-1.41169958549474));
#57333=CARTESIAN_POINT('Ctrl Pts',(-21.4116339245492,-1.08307091109002,
-1.10067050352125));
#57334=CARTESIAN_POINT('Ctrl Pts',(-21.4381484669549,-1.30449718850049,
-0.668736826869823));
#57335=CARTESIAN_POINT('Ctrl Pts',(-21.450713962689,-1.4094332232862,-0.464039318298204));
#57336=CARTESIAN_POINT('Ctrl Pts',(-21.4632794584231,-1.46140026781191,
-0.232187811403527));
#57337=CARTESIAN_POINT('Ctrl Pts',(-21.4758449541571,-1.46110336159793,
-0.000210604951717125));
#57338=CARTESIAN_POINT('Ctrl Pts',(-21.5471550458428,-1.46119914789583,
-0.000442129891295945));
#57339=CARTESIAN_POINT('Ctrl Pts',(-21.5353705336236,-1.46178585356219,
-0.217965677876684));
#57340=CARTESIAN_POINT('Ctrl Pts',(-21.5235860214044,-1.41633808391013,
-0.435256174586171));
#57341=CARTESIAN_POINT('Ctrl Pts',(-21.5118015091852,-1.32361817707143,
-0.630045034625424));
#57342=CARTESIAN_POINT('Ctrl Pts',(-21.4852869667795,-1.11500318682023,
-1.06830988543918));
#57343=CARTESIAN_POINT('Ctrl Pts',(-21.4587724243738,-0.66708401474874,
-1.39266544267209));
#57344=CARTESIAN_POINT('Ctrl Pts',(-21.4322578819681,-0.185607792922169,
-1.45412226842745));
#57345=CARTESIAN_POINT('Ctrl Pts',(-21.4057433395624,0.295868428904401,
-1.51557909418281));
#57346=CARTESIAN_POINT('Ctrl Pts',(-21.3792287971567,0.810901700486049,
-1.31413718846062));
#57347=CARTESIAN_POINT('Ctrl Pts',(-21.3527142547511,1.12291670834372,-0.942326849056391));
#57348=CARTESIAN_POINT('Ctrl Pts',(-21.3261997123454,1.43493171620138,-0.570516509652169));
#57349=CARTESIAN_POINT('Ctrl Pts',(-21.2996851699397,1.54392846033508,-0.0283377365659148));
#57350=CARTESIAN_POINT('Ctrl Pts',(-21.273170627534,1.3998403910005,0.435165145724725));
#57351=CARTESIAN_POINT('Ctrl Pts',(-21.2466560851283,1.2557523216659,0.898668028015379));
#57352=CARTESIAN_POINT('Ctrl Pts',(-21.2201415427226,0.858579438863007,
1.28349501951041));
#57353=CARTESIAN_POINT('Ctrl Pts',(-21.1936270003169,0.390759080991175,
1.41287974185809));
#57354=CARTESIAN_POINT('Ctrl Pts',(-21.1671124579112,-0.0770612768806438,
1.54226446420576));
#57355=CARTESIAN_POINT('Ctrl Pts',(-21.1405979155056,-0.615529109821396,
1.41620691740608));
#57356=CARTESIAN_POINT('Ctrl Pts',(-21.1140833730999,-0.977304676099182,
1.09261035799809));
#57357=CARTESIAN_POINT('Ctrl Pts',(-21.0917739306809,-1.2817040898621,0.820334913879643));
#57358=CARTESIAN_POINT('Ctrl Pts',(-21.0694644882619,-1.46101232011646,
0.408209609079869));
#57359=CARTESIAN_POINT('Ctrl Pts',(-21.0471550458428,-1.46458686986414,
-0.00117242835359658));
#57360=CARTESIAN_POINT('Origin',(-17.3,0.,0.));
#57361=CARTESIAN_POINT('',(-20.4758449541571,-1.46534501698659,0.00082302614468642));
#57362=CARTESIAN_POINT('',(-20.5471550458428,-1.46500269836855,0.00101311012710306));
#57363=CARTESIAN_POINT('',(-17.3,-1.4635,-1.79227059055215E-16));
#57364=CARTESIAN_POINT('Ctrl Pts',(-20.4758449541571,-1.46534501698659,
0.00082302614468642));
#57365=CARTESIAN_POINT('Ctrl Pts',(-20.4784382828881,-1.46566459987453,
0.0483467506841562));
#57366=CARTESIAN_POINT('Ctrl Pts',(-20.4810316116192,-1.46355390104093,
0.0958417285952254));
#57367=CARTESIAN_POINT('Ctrl Pts',(-20.4836249403502,-1.45891991962591,
0.143089225787058));
#57368=CARTESIAN_POINT('Ctrl Pts',(-20.5101394827559,-1.4115414691944,0.626154003832599));
#57369=CARTESIAN_POINT('Ctrl Pts',(-20.5366540251616,-1.10039689364073,
1.08334889681806));
#57370=CARTESIAN_POINT('Ctrl Pts',(-20.5631685675672,-0.668407300319506,
1.30466606428511));
#57371=CARTESIAN_POINT('Ctrl Pts',(-20.5896831099729,-0.236417706998265,
1.52598323175217));
#57372=CARTESIAN_POINT('Ctrl Pts',(-20.6161976523786,0.316416904090545,
1.51142267370079));
#57373=CARTESIAN_POINT('Ctrl Pts',(-20.6427121947843,0.736157557278878,
1.26767263490177));
#57374=CARTESIAN_POINT('Ctrl Pts',(-20.66922673719,1.15589821046721,1.02392259610275));
#57375=CARTESIAN_POINT('Ctrl Pts',(-20.6957412795957,1.44254490575507,0.550983076556086));
#57376=CARTESIAN_POINT('Ctrl Pts',(-20.7222558220014,1.46442938880383,0.0660940513604433));
#57377=CARTESIAN_POINT('Ctrl Pts',(-20.7487703644071,1.4863138718526,-0.418794973835186));
#57378=CARTESIAN_POINT('Ctrl Pts',(-20.7752849068128,1.2434361426623,-0.915633504679789));
#57379=CARTESIAN_POINT('Ctrl Pts',(-20.8017994492184,0.84735962458967,-1.19620379744961));
#57380=CARTESIAN_POINT('Ctrl Pts',(-20.8283139916241,0.451283106517042,
-1.47677409021943));
#57381=CARTESIAN_POINT('Ctrl Pts',(-20.8548285340298,-0.09799220043791,
-1.54107614491446));
#57382=CARTESIAN_POINT('Ctrl Pts',(-20.8813430764355,-0.548162250887773,
-1.35957346440686));
#57383=CARTESIAN_POINT('Ctrl Pts',(-20.9078576188412,-0.998332301337649,
-1.17807078389924));
#57384=CARTESIAN_POINT('Ctrl Pts',(-20.9343721612469,-1.34939709528243,
-0.75076336818897));
#57385=CARTESIAN_POINT('Ctrl Pts',(-20.9608867036526,-1.44009857763784,
-0.273930547955271));
#57386=CARTESIAN_POINT('Ctrl Pts',(-20.9658727871541,-1.45715507281757,
-0.184261708057138));
#57387=CARTESIAN_POINT('Ctrl Pts',(-20.9708588706556,-1.46500430372587,
-0.0928414943390442));
#57388=CARTESIAN_POINT('Ctrl Pts',(-20.9758449541571,-1.46416452657485,
-0.00127774293595062));
#57389=CARTESIAN_POINT('Ctrl Pts',(-21.0471550458428,-1.46458686986414,
-0.00117242835359658));
#57390=CARTESIAN_POINT('Ctrl Pts',(-21.0429499458562,-1.46526063565416,
-0.0783367235349625));
#57391=CARTESIAN_POINT('Ctrl Pts',(-21.0387448458695,-1.45969087111027,
-0.155403554912202));
#57392=CARTESIAN_POINT('Ctrl Pts',(-21.0345397458828,-1.44753843707036,
-0.231418014713479));
#57393=CARTESIAN_POINT('Ctrl Pts',(-21.0080252034771,-1.37091333214893,
-0.710714256000721));
#57394=CARTESIAN_POINT('Ctrl Pts',(-20.9815106610714,-1.03257982269125,
-1.14817116655891));
#57395=CARTESIAN_POINT('Ctrl Pts',(-20.9549961186658,-0.587947977283016,
-1.34284734811476));
#57396=CARTESIAN_POINT('Ctrl Pts',(-20.9284815762601,-0.143316131874758,
-1.53752352967063));
#57397=CARTESIAN_POINT('Ctrl Pts',(-20.9019670338544,0.407614049484076,
-1.48941898222413));
#57398=CARTESIAN_POINT('Ctrl Pts',(-20.8754524914487,0.811778371620634,
-1.22063004210899));
#57399=CARTESIAN_POINT('Ctrl Pts',(-20.848937949043,1.21594269375717,-0.951841101993865));
#57400=CARTESIAN_POINT('Ctrl Pts',(-20.8224234066373,1.47334115667146,-0.462367769210122));
#57401=CARTESIAN_POINT('Ctrl Pts',(-20.7959088642316,1.46574038513714,0.0229553416020292));
#57402=CARTESIAN_POINT('Ctrl Pts',(-20.7693943218259,1.45813961360282,0.508278452414194));
#57403=CARTESIAN_POINT('Ctrl Pts',(-20.7428797794203,1.1855396076199,0.989451341254735));
#57404=CARTESIAN_POINT('Ctrl Pts',(-20.7163652370146,0.773156417156846,
1.24545211828445));
#57405=CARTESIAN_POINT('Ctrl Pts',(-20.6898506946089,0.3607732266938,1.50145289531416));
#57406=CARTESIAN_POINT('Ctrl Pts',(-20.6633361522032,-0.19139314824938,
1.53228156053303));
#57407=CARTESIAN_POINT('Ctrl Pts',(-20.6368216097975,-0.629710679505619,
1.32377727901887));
#57408=CARTESIAN_POINT('Ctrl Pts',(-20.6103070673918,-1.06802821076187,
1.11527299750471));
#57409=CARTESIAN_POINT('Ctrl Pts',(-20.5837925249862,-1.39249689833119,
0.667435769257517));
#57410=CARTESIAN_POINT('Ctrl Pts',(-20.5572779825805,-1.4540753390434,0.185975086277314));
#57411=CARTESIAN_POINT('Ctrl Pts',(-20.5539036703346,-1.46191197764716,
0.124703099997769));
#57412=CARTESIAN_POINT('Ctrl Pts',(-20.5505293580887,-1.46549089978,0.0628865551477272));
#57413=CARTESIAN_POINT('Ctrl Pts',(-20.5471550458428,-1.46500269836855,
0.00101311012710306));
#57414=CARTESIAN_POINT('Origin',(-17.3,0.,0.));
#57415=CARTESIAN_POINT('',(-19.9758449541571,-1.46160352170699,0.000870148659567124));
#57416=CARTESIAN_POINT('',(-20.0471550458428,-1.46137421934213,0.000673585972547344));
#57417=CARTESIAN_POINT('',(-17.3,-1.4635,-1.79227059055215E-16));
#57418=CARTESIAN_POINT('Ctrl Pts',(-19.9758449541571,-1.46160352170699,
0.000870148659567124));
#57419=CARTESIAN_POINT('Ctrl Pts',(-19.9860176951207,-1.46261643292029,
0.188513100842206));
#57420=CARTESIAN_POINT('Ctrl Pts',(-19.9961904360843,-1.42911507721764,
0.375808090111529));
#57421=CARTESIAN_POINT('Ctrl Pts',(-20.0063631770478,-1.35943495977707,
0.548505650429889));
#57422=CARTESIAN_POINT('Ctrl Pts',(-20.0328777194535,-1.17781857582257,
0.998629840440597));
#57423=CARTESIAN_POINT('Ctrl Pts',(-20.0593922618592,-0.750422497676223,
1.34958668886163));
#57424=CARTESIAN_POINT('Ctrl Pts',(-20.0859068042649,-0.273566782208699,
1.44016772429102));
#57425=CARTESIAN_POINT('Ctrl Pts',(-20.1124213466706,0.203288933258798,
1.53074875972041));
#57426=CARTESIAN_POINT('Ctrl Pts',(-20.1389358890763,0.729604286047465,
1.3609539821582));
#57427=CARTESIAN_POINT('Ctrl Pts',(-20.165450431482,1.06362165301883,1.00877690182077));
#57428=CARTESIAN_POINT('Ctrl Pts',(-20.1919649738876,1.39763901999021,0.656599821483317));
#57429=CARTESIAN_POINT('Ctrl Pts',(-20.2184795162933,1.53935840114426,0.122040438370631));
#57430=CARTESIAN_POINT('Ctrl Pts',(-20.244994058699,1.42368243506273,-0.349356812602059));
#57431=CARTESIAN_POINT('Ctrl Pts',(-20.2715086011047,1.3080064689812,-0.820754063574708));
#57432=CARTESIAN_POINT('Ctrl Pts',(-20.2980231435104,0.934935155664138,
-1.22898918240737));
#57433=CARTESIAN_POINT('Ctrl Pts',(-20.3245376859161,0.475835021835091,
-1.38654350469533));
#57434=CARTESIAN_POINT('Ctrl Pts',(-20.3510522283218,0.0167348880060186,
-1.54409782698329));
#57435=CARTESIAN_POINT('Ctrl Pts',(-20.3775667707274,-0.528394066335047,
-1.45097135272652));
#57436=CARTESIAN_POINT('Ctrl Pts',(-20.4040813131331,-0.909152380850908,
-1.14994078404531));
#57437=CARTESIAN_POINT('Ctrl Pts',(-20.4280025268078,-1.2526695670265,-0.878353349276634));
#57438=CARTESIAN_POINT('Ctrl Pts',(-20.4519237404825,-1.46239714136337,
-0.437542212986177));
#57439=CARTESIAN_POINT('Ctrl Pts',(-20.4758449541571,-1.46534501698659,
0.00082302614468642));
#57440=CARTESIAN_POINT('Ctrl Pts',(-20.5471550458428,-1.46500269836855,
0.00101311012710306));
#57441=CARTESIAN_POINT('Ctrl Pts',(-20.524014815683,-1.46165472930044,-0.423300247448411));
#57442=CARTESIAN_POINT('Ctrl Pts',(-20.5008745855232,-1.26703441745964,
-0.850289557404769));
#57443=CARTESIAN_POINT('Ctrl Pts',(-20.4777343553634,-0.942610458482033,
-1.12267864854122));
#57444=CARTESIAN_POINT('Ctrl Pts',(-20.4512198129577,-0.570878943353276,
-1.43478756266641));
#57445=CARTESIAN_POINT('Ctrl Pts',(-20.424705270552,-0.0287277192406266,
-1.54392125320354));
#57446=CARTESIAN_POINT('Ctrl Pts',(-20.3981907281463,0.434811543720077,
-1.39995026546581));
#57447=CARTESIAN_POINT('Ctrl Pts',(-20.3716761857407,0.898350806680754,
-1.25597927772809));
#57448=CARTESIAN_POINT('Ctrl Pts',(-20.345161643335,1.28327810848951,-0.858903611715504));
#57449=CARTESIAN_POINT('Ctrl Pts',(-20.3186471009293,1.41278099426858,-0.391115950280114));
#57450=CARTESIAN_POINT('Ctrl Pts',(-20.2921325585236,1.54228388004766,0.0766717111552901));
#57451=CARTESIAN_POINT('Ctrl Pts',(-20.2656180161179,1.41636234979709,0.615171368013523));
#57452=CARTESIAN_POINT('Ctrl Pts',(-20.2391034737122,1.09285718223258,0.977028660568718));
#57453=CARTESIAN_POINT('Ctrl Pts',(-20.2125889313065,0.769352014668082,
1.3388859531239));
#57454=CARTESIAN_POINT('Ctrl Pts',(-20.1860743889009,0.248263209789676,
1.52410088137606));
#57455=CARTESIAN_POINT('Ctrl Pts',(-20.1595598464952,-0.231052371076101,
1.44759684517139));
#57456=CARTESIAN_POINT('Ctrl Pts',(-20.1330453040895,-0.710367951941878,
1.37109280896672));
#57457=CARTESIAN_POINT('Ctrl Pts',(-20.1065307616838,-1.14791030879501,
1.03286980830523));
#57458=CARTESIAN_POINT('Ctrl Pts',(-20.0800162192781,-1.34269879447265,
0.58828715067707));
#57459=CARTESIAN_POINT('Ctrl Pts',(-20.0690624947997,-1.4231700834369,0.404620547458549));
#57460=CARTESIAN_POINT('Ctrl Pts',(-20.0581087703212,-1.4622107443168,0.202801618307486));
#57461=CARTESIAN_POINT('Ctrl Pts',(-20.0471550458428,-1.46137421934213,
0.000673585972547344));
#57462=CARTESIAN_POINT('Origin',(-17.3,0.,0.));
#57463=CARTESIAN_POINT('',(-19.4758449541571,-1.46215770122242,-0.00115350946124346));
#57464=CARTESIAN_POINT('',(-19.5471550458428,-1.46252866632904,-0.00126132249279813));
#57465=CARTESIAN_POINT('',(-17.3,-1.4635,-1.79227059055215E-16));
#57466=CARTESIAN_POINT('Ctrl Pts',(-19.4758449541571,-1.46215770122242,
-0.00115350946124346));
#57467=CARTESIAN_POINT('Ctrl Pts',(-19.4935971073532,-1.45975765968372,
0.325985142341861));
#57468=CARTESIAN_POINT('Ctrl Pts',(-19.5113492605494,-1.35132302816047,
0.654566464045283));
#57469=CARTESIAN_POINT('Ctrl Pts',(-19.5291014137455,-1.14971110297745,
0.909442817393143));
#57470=CARTESIAN_POINT('Ctrl Pts',(-19.5556159561512,-0.848584367493725,
1.2901250819267));
#57471=CARTESIAN_POINT('Ctrl Pts',(-19.5821304985569,-0.339595062884128,
1.5063841970214));
#57472=CARTESIAN_POINT('Ctrl Pts',(-19.6086450409625,0.143457732345712,
1.45888372992773));
#57473=CARTESIAN_POINT('Ctrl Pts',(-19.6351595833682,0.626510527575551,
1.41138326283405));
#57474=CARTESIAN_POINT('Ctrl Pts',(-19.6616741257739,1.08362681342564,1.10012321355205));
#57475=CARTESIAN_POINT('Ctrl Pts',(-19.6881886681796,1.30483485682866,0.668077731123071));
#57476=CARTESIAN_POINT('Ctrl Pts',(-19.7147032105853,1.52604290023169,0.236032248694066));
#57477=CARTESIAN_POINT('Ctrl Pts',(-19.741217752991,1.51134270118758,-0.316798666881903));
#57478=CARTESIAN_POINT('Ctrl Pts',(-19.7677322953967,1.26748664714187,-0.736477737433156));
#57479=CARTESIAN_POINT('Ctrl Pts',(-19.7942468378024,1.02363059309619,-1.15615680798437));
#57480=CARTESIAN_POINT('Ctrl Pts',(-19.820761380208,0.550618684048914,-1.44268403351091));
#57481=CARTESIAN_POINT('Ctrl Pts',(-19.8472759226137,0.0657241464821964,
-1.46444603689818));
#57482=CARTESIAN_POINT('Ctrl Pts',(-19.8737904650194,-0.419170391084549,
-1.48620804028545));
#57483=CARTESIAN_POINT('Ctrl Pts',(-19.9003050074251,-0.915947557170757,
-1.24320482153345));
#57484=CARTESIAN_POINT('Ctrl Pts',(-19.9268195498308,-1.19641779533251,
-0.847057446357269));
#57485=CARTESIAN_POINT('Ctrl Pts',(-19.9431613512729,-1.36928100648401,
-0.602898537337132));
#57486=CARTESIAN_POINT('Ctrl Pts',(-19.959503152715,-1.45997635023122,-0.300565214489629));
#57487=CARTESIAN_POINT('Ctrl Pts',(-19.9758449541571,-1.46160352170699,
0.000870148659567124));
#57488=CARTESIAN_POINT('Ctrl Pts',(-20.0471550458428,-1.46137421934213,
0.000673585972547344));
#57489=CARTESIAN_POINT('Ctrl Pts',(-20.0315942279156,-1.46018585525209,
-0.286468702055025));
#57490=CARTESIAN_POINT('Ctrl Pts',(-20.0160334099883,-1.37852161398207,
-0.574234789112791));
#57491=CARTESIAN_POINT('Ctrl Pts',(-20.000472592061,-1.22083505168199,-0.811470024655674));
#57492=CARTESIAN_POINT('Ctrl Pts',(-19.9739580496554,-0.952148208711604,
-1.21570222776534));
#57493=CARTESIAN_POINT('Ctrl Pts',(-19.9474435072497,-0.462739908268787,
-1.47322431938986));
#57494=CARTESIAN_POINT('Ctrl Pts',(-19.920928964844,0.0225851069530342,
-1.46574613670784));
#57495=CARTESIAN_POINT('Ctrl Pts',(-19.8944144224383,0.507910122174897,
-1.45826795402582));
#57496=CARTESIAN_POINT('Ctrl Pts',(-19.8678998800326,0.98915185217573,-1.18578949703718));
#57497=CARTESIAN_POINT('Ctrl Pts',(-19.8413853376269,1.24525678562698,-0.773470983411786));
#57498=CARTESIAN_POINT('Ctrl Pts',(-19.8148707952212,1.50136171907822,-0.361152469786414));
#57499=CARTESIAN_POINT('Ctrl Pts',(-19.7883562528155,1.53232985597991,0.191006100475701));
#57500=CARTESIAN_POINT('Ctrl Pts',(-19.7618417104099,1.3239362965059,0.629376284208643));
#57501=CARTESIAN_POINT('Ctrl Pts',(-19.7353271680042,1.11554273703188,1.06774646794161));
#57502=CARTESIAN_POINT('Ctrl Pts',(-19.7088126255985,0.667787481182143,
1.39232826514539));
#57503=CARTESIAN_POINT('Ctrl Pts',(-19.6822980831928,0.186342367766726,
1.45402831688559));
#57504=CARTESIAN_POINT('Ctrl Pts',(-19.6557835407871,-0.295102745648651,
1.51572836862577));
#57505=CARTESIAN_POINT('Ctrl Pts',(-19.6292689983814,-0.8102377166297,1.31454667490242));
#57506=CARTESIAN_POINT('Ctrl Pts',(-19.6027544559757,-1.12244051710899,
0.942894007766594));
#57507=CARTESIAN_POINT('Ctrl Pts',(-19.5842213192648,-1.340664052492,0.683116200417021));
#57508=CARTESIAN_POINT('Ctrl Pts',(-19.5656881825538,-1.45974038043436,
0.340050854567538));
#57509=CARTESIAN_POINT('Ctrl Pts',(-19.5471550458428,-1.46252866632904,
-0.00126132249279813));
#57510=CARTESIAN_POINT('Origin',(-17.3,0.,0.));
#57511=CARTESIAN_POINT('',(-18.9758449541571,-1.46578778306489,-0.000400814154694062));
#57512=CARTESIAN_POINT('',(-19.0471550458428,-1.46590402480283,-0.00013840560174719));
#57513=CARTESIAN_POINT('',(-17.3,-1.4635,-1.79227059055215E-16));
#57514=CARTESIAN_POINT('Ctrl Pts',(-18.9758449541571,-1.46578778306489,
-0.000400814154694062));
#57515=CARTESIAN_POINT('Ctrl Pts',(-19.0011765195858,-1.4641024380076,0.463438220880033));
#57516=CARTESIAN_POINT('Ctrl Pts',(-19.0265080850145,-1.22529568750056,
0.928770590448006));
#57517=CARTESIAN_POINT('Ctrl Pts',(-19.0518396504431,-0.846755214080442,
1.19663171688084));
#57518=CARTESIAN_POINT('Ctrl Pts',(-19.0783541928488,-0.450537007075949,
1.47700188253981));
#57519=CARTESIAN_POINT('Ctrl Pts',(-19.1048687352545,0.0987707141235838,
1.54102644422561));
#57520=CARTESIAN_POINT('Ctrl Pts',(-19.1313832776602,0.548849014975999,
1.35929636841179));
#57521=CARTESIAN_POINT('Ctrl Pts',(-19.1578978200659,0.998927315828401,
1.17756629259798));
#57522=CARTESIAN_POINT('Ctrl Pts',(-19.1844123624716,1.34977619633369,0.750081579284574));
#57523=CARTESIAN_POINT('Ctrl Pts',(-19.2109269048772,1.44023677905777,0.273202999007897));
#57524=CARTESIAN_POINT('Ctrl Pts',(-19.2374414472829,1.53069736178185,-0.203675581268794));
#57525=CARTESIAN_POINT('Ctrl Pts',(-19.2639559896886,1.36076964672472,-0.72994802850872));
#57526=CARTESIAN_POINT('Ctrl Pts',(-19.2904705320943,1.00850820759375,-1.06387642780243));
#57527=CARTESIAN_POINT('Ctrl Pts',(-19.3169850745,0.656246768462777,-1.39780482709613));
#57528=CARTESIAN_POINT('Ctrl Pts',(-19.3434996169057,0.121651605257916,
-1.5393891784436));
#57529=CARTESIAN_POINT('Ctrl Pts',(-19.3700141593114,-0.349716411882835,
-1.42359414499969));
#57530=CARTESIAN_POINT('Ctrl Pts',(-19.3965287017171,-0.821084429023599,
-1.30779911155578));
#57531=CARTESIAN_POINT('Ctrl Pts',(-19.4230432441227,-1.22922530010029,
-0.934624693320504));
#57532=CARTESIAN_POINT('Ctrl Pts',(-19.4495577865284,-1.38666365245969,
-0.475484777216653));
#57533=CARTESIAN_POINT('Ctrl Pts',(-19.458320175738,-1.43869306706458,-0.323750586032459));
#57534=CARTESIAN_POINT('Ctrl Pts',(-19.4670825649475,-1.46334235177432,
-0.162627791533922));
#57535=CARTESIAN_POINT('Ctrl Pts',(-19.4758449541571,-1.46215770122242,
-0.00115350946124346));
#57536=CARTESIAN_POINT('Ctrl Pts',(-19.5471550458428,-1.46252866632904,
-0.00126132249279813));
#57537=CARTESIAN_POINT('Ctrl Pts',(-19.5391736401481,-1.46372945825462,
-0.148249444155522));
#57538=CARTESIAN_POINT('Ctrl Pts',(-19.5311922344534,-1.4433629405794,-0.294912415154495));
#57539=CARTESIAN_POINT('Ctrl Pts',(-19.5232108287587,-1.40006005061068,
-0.434457913973326));
#57540=CARTESIAN_POINT('Ctrl Pts',(-19.496696286353,-1.25620615365555,-0.898033528029032));
#57541=CARTESIAN_POINT('Ctrl Pts',(-19.4701817439473,-0.85922772976778,
-1.2830611155921));
#57542=CARTESIAN_POINT('Ctrl Pts',(-19.4436672015416,-0.391472794614882,
-1.41268215653998));
#57543=CARTESIAN_POINT('Ctrl Pts',(-19.4171526591359,0.0762821405380149,
-1.54230319748786));
#57544=CARTESIAN_POINT('Ctrl Pts',(-19.3906381167303,0.614813586956024,
-1.41651769182055));
#57545=CARTESIAN_POINT('Ctrl Pts',(-19.3641235743246,0.976752582701203,
-1.09310393674004));
#57546=CARTESIAN_POINT('Ctrl Pts',(-19.3376090319189,1.33869157844639,-0.769690181659522));
#57547=CARTESIAN_POINT('Ctrl Pts',(-19.3110944895132,1.52403812351873,-0.248648177165766));
#57548=CARTESIAN_POINT('Ctrl Pts',(-19.2845799471075,1.44765516091198,0.230686712696983));
#57549=CARTESIAN_POINT('Ctrl Pts',(-19.2580654047018,1.37127219830524,0.710021602559718));
#57550=CARTESIAN_POINT('Ctrl Pts',(-19.2315508622961,1.03315972801944,1.14764937779147));
#57551=CARTESIAN_POINT('Ctrl Pts',(-19.2050363198904,0.588626286536881,
1.34255015516287));
#57552=CARTESIAN_POINT('Ctrl Pts',(-19.1785217774848,0.144092845054323,
1.53745093253427));
#57553=CARTESIAN_POINT('Ctrl Pts',(-19.1520072350791,-0.406861567624983,
1.48962471204531));
#57554=CARTESIAN_POINT('Ctrl Pts',(-19.1254926926734,-0.811161625916757,
1.22103998336259));
#57555=CARTESIAN_POINT('Ctrl Pts',(-19.0993801437299,-1.20933199214373,
0.956527333440112));
#57556=CARTESIAN_POINT('Ctrl Pts',(-19.0732675947863,-1.46526121859312,
0.477899378505275));
#57557=CARTESIAN_POINT('Ctrl Pts',(-19.0471550458428,-1.46590402480283,
-0.00013840560174719));
#57558=CARTESIAN_POINT('Origin',(-17.3,0.,0.));
#57559=CARTESIAN_POINT('',(-18.4758449541571,-1.46337413104549,0.00135256974678304));
#57560=CARTESIAN_POINT('',(-18.5471550458428,-1.46294584879644,0.00133002991220975));
#57561=CARTESIAN_POINT('',(-17.3,-1.4635,-1.79227059055215E-16));
#57562=CARTESIAN_POINT('Ctrl Pts',(-18.4758449541571,-1.46337413104549,
0.00135256974678304));
#57563=CARTESIAN_POINT('Ctrl Pts',(-18.4822413894126,-1.46445455751735,
0.11897860929348));
#57564=CARTESIAN_POINT('Ctrl Pts',(-18.4886378246682,-1.45146917310825,
0.236369036177189));
#57565=CARTESIAN_POINT('Ctrl Pts',(-18.4950342599237,-1.42350576410765,
0.350075988850877));
#57566=CARTESIAN_POINT('Ctrl Pts',(-18.5215488023294,-1.30759167068936,
0.821414742085207));
#57567=CARTESIAN_POINT('Ctrl Pts',(-18.5480633447351,-0.934314171345385,
1.22946133936544));
#57568=CARTESIAN_POINT('Ctrl Pts',(-18.5745778871408,-0.475134502261091,
1.3867837117513));
#57569=CARTESIAN_POINT('Ctrl Pts',(-18.6010924295465,-0.0159548331767707,
1.54410608413717));
#57570=CARTESIAN_POINT('Ctrl Pts',(-18.6276069719521,0.529127005647898,
1.45070423162863));
#57571=CARTESIAN_POINT('Ctrl Pts',(-18.6541215143578,0.909733195910636,
1.149481348555));
#57572=CARTESIAN_POINT('Ctrl Pts',(-18.6806360567635,1.29033938617334,0.848258465481405));
#57573=CARTESIAN_POINT('Ctrl Pts',(-18.7071505991692,1.50646992787416,0.339214551842755));
#57574=CARTESIAN_POINT('Ctrl Pts',(-18.7336651415749,1.45884744714899,-0.143826229751351));
#57575=CARTESIAN_POINT('Ctrl Pts',(-18.7601796839806,1.41122496642381,-0.626867011345499));
#57576=CARTESIAN_POINT('Ctrl Pts',(-18.7866942263863,1.09984946327261,-1.08390466089507));
#57577=CARTESIAN_POINT('Ctrl Pts',(-18.8132087687919,0.667748119301473,
-1.3050035661204));
#57578=CARTESIAN_POINT('Ctrl Pts',(-18.8397233111976,0.235646775330358,
-1.52610247134571));
#57579=CARTESIAN_POINT('Ctrl Pts',(-18.8662378536033,-0.317180409460681,
-1.51126263224677));
#57580=CARTESIAN_POINT('Ctrl Pts',(-18.892752396009,-0.736797870598213,
-1.26730057851306));
#57581=CARTESIAN_POINT('Ctrl Pts',(-18.9192669384147,-1.15641533173576,
-1.02333852477935));
#57582=CARTESIAN_POINT('Ctrl Pts',(-18.9457814808204,-1.4428230692198,-0.550254256410852));
#57583=CARTESIAN_POINT('Ctrl Pts',(-18.9722960232261,-1.46446259155709,
-0.065354237410539));
#57584=CARTESIAN_POINT('Ctrl Pts',(-18.9734790002031,-1.46542806387514,
-0.0437198622117143));
#57585=CARTESIAN_POINT('Ctrl Pts',(-18.9746619771801,-1.4658664882048,-0.0220619665627543));
#57586=CARTESIAN_POINT('Ctrl Pts',(-18.9758449541571,-1.46578778306489,
-0.000400814154694062));
#57587=CARTESIAN_POINT('Ctrl Pts',(-19.0471550458428,-1.46590402480283,
-0.00013840560174719));
#57588=CARTESIAN_POINT('Ctrl Pts',(-19.0467530523807,-1.46591392057724,
-0.00749762833770351));
#57589=CARTESIAN_POINT('Ctrl Pts',(-19.0463510589185,-1.46586331470994,
-0.0148567112060816));
#57590=CARTESIAN_POINT('Ctrl Pts',(-19.0459490654563,-1.46575179476014,
-0.0222148708632159));
#57591=CARTESIAN_POINT('Ctrl Pts',(-19.0194345230506,-1.45839620140749,
-0.507541759529738));
#57592=CARTESIAN_POINT('Ctrl Pts',(-18.9929199806449,-1.18603931079801,
-0.988852299986267));
#57593=CARTESIAN_POINT('Ctrl Pts',(-18.9664054382393,-0.773785500317309,
-1.24506137351889));
#57594=CARTESIAN_POINT('Ctrl Pts',(-18.9398908958336,-0.361531689836588,
-1.50127044705152));
#57595=CARTESIAN_POINT('Ctrl Pts',(-18.9133763534279,0.190619040515314,
-1.53237805366019));
#57596=CARTESIAN_POINT('Ctrl Pts',(-18.8868618110222,0.62904184875583,-1.32409522952237));
#57597=CARTESIAN_POINT('Ctrl Pts',(-18.8603472686165,1.06746465699632,-1.11581240538456));
#57598=CARTESIAN_POINT('Ctrl Pts',(-18.8338327262108,1.39215954312542,-0.66813915050023));
#57599=CARTESIAN_POINT('Ctrl Pts',(-18.8073181838051,1.45398120195699,-0.186709637367093));
#57600=CARTESIAN_POINT('Ctrl Pts',(-18.7808036413995,1.51580286078856,0.294719875766044));
#57601=CARTESIAN_POINT('Ctrl Pts',(-18.7542890989938,1.31475129232266,0.809905647148002));
#57602=CARTESIAN_POINT('Ctrl Pts',(-18.7277745565881,0.943177496892139,
1.12220231406209));
#57603=CARTESIAN_POINT('Ctrl Pts',(-18.7012600141824,0.571603701461615,
1.43449898097619));
#57604=CARTESIAN_POINT('Ctrl Pts',(-18.6747454717767,0.0295076790664164,
1.54390654342238));
#57605=CARTESIAN_POINT('Ctrl Pts',(-18.648230929371,-0.434104256506996,
1.40016974642811));
#57606=CARTESIAN_POINT('Ctrl Pts',(-18.6217163869653,-0.897716192080435,
1.25643294943382));
#57607=CARTESIAN_POINT('Ctrl Pts',(-18.5952018445597,-1.2828440408321,0.859551792999085));
#57608=CARTESIAN_POINT('Ctrl Pts',(-18.568687302154,-1.41258322867861,0.391829613972634));
#57609=CARTESIAN_POINT('Ctrl Pts',(-18.5615098833836,-1.44770329478633,
0.265218417154564));
#57610=CARTESIAN_POINT('Ctrl Pts',(-18.5543324646132,-1.46410921932681,
0.133416195328377));
#57611=CARTESIAN_POINT('Ctrl Pts',(-18.5471550458428,-1.46294584879644,
0.00133002991220975));
#57612=CARTESIAN_POINT('Origin',(-17.3,0.,0.));
#57613=CARTESIAN_POINT('',(-17.9758449541571,-1.46110551485691,-0.000218695958779103));
#57614=CARTESIAN_POINT('',(-18.0471550458428,-1.46120363688599,-0.000449877262721942));
#57615=CARTESIAN_POINT('',(-17.3,-1.4635,-1.79227059055215E-16));
#57616=CARTESIAN_POINT('Ctrl Pts',(-17.9758449541571,-1.46110551485691,
-0.000218695958779103));
#57617=CARTESIAN_POINT('Ctrl Pts',(-17.9898208016452,-1.4607625691127,0.257794693658319));
#57618=CARTESIAN_POINT('Ctrl Pts',(-18.0037966491333,-1.39576298805581,
0.515969572122497));
#57619=CARTESIAN_POINT('Ctrl Pts',(-18.0177724966213,-1.26711442902716,
0.737117956753728));
#57620=CARTESIAN_POINT('Ctrl Pts',(-18.044287039027,-1.02304639117082,1.15667378170486));
#57621=CARTESIAN_POINT('Ctrl Pts',(-18.0708015814327,-0.549889793665136,
1.44296201287282));
#57622=CARTESIAN_POINT('Ctrl Pts',(-18.0973161238384,-0.0649843241691522,
1.46447905277948));
#57623=CARTESIAN_POINT('Ctrl Pts',(-18.1238306662441,0.419921145326859,
1.48599609268614));
#57624=CARTESIAN_POINT('Ctrl Pts',(-18.1503452086498,0.916575486813129,
1.2427419413315));
#57625=CARTESIAN_POINT('Ctrl Pts',(-18.1768597510555,1.19684556208097,0.84645292777844));
#57626=CARTESIAN_POINT('Ctrl Pts',(-18.2033742934612,1.4771156373488,0.450163914225396));
#57627=CARTESIAN_POINT('Ctrl Pts',(-18.2298888358668,1.54100144639816,-0.0991599615260736));
#57628=CARTESIAN_POINT('Ctrl Pts',(-18.2564033782725,1.35915769031991,-0.549192344504046));
#57629=CARTESIAN_POINT('Ctrl Pts',(-18.2829179206782,1.17731393424166,-0.99922472748203));
#57630=CARTESIAN_POINT('Ctrl Pts',(-18.3094324630839,0.749740613035781,
-1.34996561768655));
#57631=CARTESIAN_POINT('Ctrl Pts',(-18.3359470054896,0.272839198375997,
-1.44030574193369));
#57632=CARTESIAN_POINT('Ctrl Pts',(-18.3624615478953,-0.204062216283761,
-1.53064586618082));
#57633=CARTESIAN_POINT('Ctrl Pts',(-18.388976090301,-0.730291724397424,
-1.3605852244706));
#57634=CARTESIAN_POINT('Ctrl Pts',(-18.4154906327066,-1.06413113470796,
-1.00823944902129));
#57635=CARTESIAN_POINT('Ctrl Pts',(-18.4356087398568,-1.31743428151736,
-0.740894459395029));
#57636=CARTESIAN_POINT('Ctrl Pts',(-18.455726847007,-1.45997596712131,-0.368605566732589));
#57637=CARTESIAN_POINT('Ctrl Pts',(-18.4758449541571,-1.46337413104549,
0.00135256974678304));
#57638=CARTESIAN_POINT('Ctrl Pts',(-18.5471550458428,-1.46294584879644,
0.00133002991220975));
#57639=CARTESIAN_POINT('Ctrl Pts',(-18.5278179222075,-1.45981154097644,
-0.354531400621349));
#57640=CARTESIAN_POINT('Ctrl Pts',(-18.5084807985722,-1.3291504183923,-0.712453837100621));
#57641=CARTESIAN_POINT('Ctrl Pts',(-18.4891436749369,-1.09335062150458,
-0.976476442514407));
#57642=CARTESIAN_POINT('Ctrl Pts',(-18.4626291325312,-0.770028299542674,
-1.33849711835691));
#57643=CARTESIAN_POINT('Ctrl Pts',(-18.4361145901255,-0.249033128677468,
-1.52397526842382));
#57644=CARTESIAN_POINT('Ctrl Pts',(-18.4096000477198,0.230321039599414,
-1.44771338428844));
#57645=CARTESIAN_POINT('Ctrl Pts',(-18.3830855053142,0.709675207876324,
-1.37145150015305));
#57646=CARTESIAN_POINT('Ctrl Pts',(-18.3565709629085,1.14738837356491,-1.03344958181541));
#57647=CARTESIAN_POINT('Ctrl Pts',(-18.3300564205028,1.34240143019492,-0.588965384840811));
#57648=CARTESIAN_POINT('Ctrl Pts',(-18.3035418780971,1.53741448682491,-0.144481187866252));
#57649=CARTESIAN_POINT('Ctrl Pts',(-18.2770273356914,1.48972743439631,0.406485287745245));
#57650=CARTESIAN_POINT('Ctrl Pts',(-18.2505127932857,1.22124483713764,0.810853175423698));
#57651=CARTESIAN_POINT('Ctrl Pts',(-18.22399825088,0.952762239878958,1.21522106310218));
#57652=CARTESIAN_POINT('Ctrl Pts',(-18.1974837084743,0.463484097790187,
1.47299036284763));
#57653=CARTESIAN_POINT('Ctrl Pts',(-18.1709691660687,-0.0218446333559495,
1.46575735929368));
#57654=CARTESIAN_POINT('Ctrl Pts',(-18.144454623663,-0.507173364502044,
1.45852435573973));
#57655=CARTESIAN_POINT('Ctrl Pts',(-18.1179400812573,-0.988552684705489,
1.18628904888644));
#57656=CARTESIAN_POINT('Ctrl Pts',(-18.0914255388516,-1.24486588197267,
0.774099967853279));
#57657=CARTESIAN_POINT('Ctrl Pts',(-18.0766687078487,-1.38751856207629,
0.544693609750165));
#57658=CARTESIAN_POINT('Ctrl Pts',(-18.0619118768458,-1.46045594798573,
0.271935909324877));
#57659=CARTESIAN_POINT('Ctrl Pts',(-18.0471550458428,-1.46120363688599,
-0.000449877262721942));
#57660=CARTESIAN_POINT('Origin',(-17.3,0.,0.));
#57661=CARTESIAN_POINT('',(-17.4758449541571,-1.46417935052163,-0.00127487220091121));
#57662=CARTESIAN_POINT('',(-17.5471550458428,-1.46460091918832,-0.00116803120312899));
#57663=CARTESIAN_POINT('',(-17.3,-1.4635,-1.79227059055215E-16));
#57664=CARTESIAN_POINT('Ctrl Pts',(-17.4758449541571,-1.46417935052163,
-0.00127487220091121));
#57665=CARTESIAN_POINT('Ctrl Pts',(-17.4974002138777,-1.46055286990098,
0.394552617929168));
#57666=CARTESIAN_POINT('Ctrl Pts',(-17.5189554735984,-1.29448215597133,
0.793060082165337));
#57667=CARTESIAN_POINT('Ctrl Pts',(-17.540510733319,-1.00797062612048,1.06438577371923));
#57668=CARTESIAN_POINT('Ctrl Pts',(-17.5670252757247,-0.655540536833363,
1.39813617374679));
#57669=CARTESIAN_POINT('Ctrl Pts',(-17.5935398181304,-0.120873915772161,
1.5394504383893));
#57670=CARTESIAN_POINT('Ctrl Pts',(-17.6200543605361,0.350435543483126,
1.42341729239225));
#57671=CARTESIAN_POINT('Ctrl Pts',(-17.6465689029417,0.821745002738413,
1.30738414639521));
#57672=CARTESIAN_POINT('Ctrl Pts',(-17.6730834453474,1.22969730018777,0.934003589758628));
#57673=CARTESIAN_POINT('Ctrl Pts',(-17.6995979877531,1.38690368256252,0.474784196990721));
#57674=CARTESIAN_POINT('Ctrl Pts',(-17.7261125301588,1.54411006493728,0.0155648042228135));
#57675=CARTESIAN_POINT('Ctrl Pts',(-17.7526270725645,1.4505705322374,-0.529493424676442));
#57676=CARTESIAN_POINT('Ctrl Pts',(-17.7791416149702,1.14925152079274,-0.9100235163847));
#57677=CARTESIAN_POINT('Ctrl Pts',(-17.8056561573759,0.847932509348076,
-1.29055360809297));
#57678=CARTESIAN_POINT('Ctrl Pts',(-17.8321706997815,0.338834019158619,
-1.50655556261026));
#57679=CARTESIAN_POINT('Ctrl Pts',(-17.8586852421872,-0.144194717980545,
-1.458811071292));
#57680=CARTESIAN_POINT('Ctrl Pts',(-17.8851997845929,-0.627223455119695,
-1.41106657997374));
#57681=CARTESIAN_POINT('Ctrl Pts',(-17.9117143269986,-1.08418243920854,
-1.09957564281995));
#57682=CARTESIAN_POINT('Ctrl Pts',(-17.9382288694043,-1.3051721921495,-0.66741846487589));
#57683=CARTESIAN_POINT('Ctrl Pts',(-17.9507675643219,-1.40967797805547,
-0.463051860022404));
#57684=CARTESIAN_POINT('Ctrl Pts',(-17.9633062592395,-1.46141319509337,
-0.231700270140578));
#57685=CARTESIAN_POINT('Ctrl Pts',(-17.9758449541571,-1.46110551485691,
-0.000218695958779103));
#57686=CARTESIAN_POINT('Ctrl Pts',(-18.0471550458428,-1.46120363688599,
-0.000449877262721942));
#57687=CARTESIAN_POINT('Ctrl Pts',(-18.0353973344401,-1.46179936847,-0.217477060692192));
#57688=CARTESIAN_POINT('Ctrl Pts',(-18.0236396230373,-1.41656670969026,
-0.434268141003884));
#57689=CARTESIAN_POINT('Ctrl Pts',(-18.0118819116345,-1.32425407805813,
-0.628707373168519));
#57690=CARTESIAN_POINT('Ctrl Pts',(-17.9853673692289,-1.1160820025455,-1.06718277794405));
#57691=CARTESIAN_POINT('Ctrl Pts',(-17.9588528268232,-0.668490777189342,
-1.39199073228205));
#57692=CARTESIAN_POINT('Ctrl Pts',(-17.9323382844175,-0.187076895054903,
-1.45393399426063));
#57693=CARTESIAN_POINT('Ctrl Pts',(-17.9058237420118,0.294336987079563,
-1.5158772562392));
#57694=CARTESIAN_POINT('Ctrl Pts',(-17.8793091996061,0.80957352599233,-1.31495582585831));
#57695=CARTESIAN_POINT('Ctrl Pts',(-17.8527946572004,1.12196403941587,-0.943460925840423));
#57696=CARTESIAN_POINT('Ctrl Pts',(-17.8262801147947,1.43435455283938,-0.571966025822565));
#57697=CARTESIAN_POINT('Ctrl Pts',(-17.7997655723891,1.54389904077372,-0.0298976561677314));
#57698=CARTESIAN_POINT('Ctrl Pts',(-17.7732510299834,1.40027935291106,0.433750571343731));
#57699=CARTESIAN_POINT('Ctrl Pts',(-17.7467364875777,1.2566596650484,0.897398798855233));
#57700=CARTESIAN_POINT('Ctrl Pts',(-17.720221945172,0.859875801388736,1.28262688422333));
#57701=CARTESIAN_POINT('Ctrl Pts',(-17.6937074027663,0.39218640833064,1.41248421069078));
#57702=CARTESIAN_POINT('Ctrl Pts',(-17.6671928603606,-0.0755029847274155,
1.54234153715822));
#57703=CARTESIAN_POINT('Ctrl Pts',(-17.6406783179549,-0.61409790718388,
1.41682810472502));
#57704=CARTESIAN_POINT('Ctrl Pts',(-17.6141637755493,-0.976200240025855,
1.09359723651055));
#57705=CARTESIAN_POINT('Ctrl Pts',(-17.5918275323138,-1.28124060839204,
0.821302765680679));
#57706=CARTESIAN_POINT('Ctrl Pts',(-17.5694912890783,-1.4610307665805,0.408695602734371));
#57707=CARTESIAN_POINT('Ctrl Pts',(-17.5471550458428,-1.46460091918832,
-0.00116803120312899));
#57708=CARTESIAN_POINT('Origin',(-17.3,0.,0.));
#57709=CARTESIAN_POINT('',(-16.9758449541571,-1.46533423939264,0.000830137543336423));
#57710=CARTESIAN_POINT('',(-17.0471550458428,-1.46499001420292,0.00101896910938441));
#57711=CARTESIAN_POINT('',(-17.3,-1.4635,-1.79227059055215E-16));
#57712=CARTESIAN_POINT('Ctrl Pts',(-16.9758449541571,-1.46533423939264,
0.000830137543336423));
#57713=CARTESIAN_POINT('Ctrl Pts',(-16.9784650837046,-1.46565935231474,
0.0488459268207528));
#57714=CARTESIAN_POINT('Ctrl Pts',(-16.9810852132521,-1.46350470201884,
0.0968321742252827));
#57715=CARTESIAN_POINT('Ctrl Pts',(-16.9837053427996,-1.4587746023591,0.144563197009661));
#57716=CARTESIAN_POINT('Ctrl Pts',(-17.0102198852053,-1.41090810349401,
0.627579858875393));
#57717=CARTESIAN_POINT('Ctrl Pts',(-17.0367344276109,-1.09930175221151,
1.0844601483484));
#57718=CARTESIAN_POINT('Ctrl Pts',(-17.0632489700166,-0.667088767867208,
1.30534073490527));
#57719=CARTESIAN_POINT('Ctrl Pts',(-17.0897635124223,-0.234875783522952,
1.52622132146211));
#57720=CARTESIAN_POINT('Ctrl Pts',(-17.116278054828,0.317943833883089,1.51110220510288));
#57721=CARTESIAN_POINT('Ctrl Pts',(-17.1427925972337,0.737437995879103,
1.26692819869613));
#57722=CARTESIAN_POINT('Ctrl Pts',(-17.1693071396394,1.15693215787514,1.02275419228936));
#57723=CARTESIAN_POINT('Ctrl Pts',(-17.1958216820451,1.44310086446115,0.549525295835037));
#57724=CARTESIAN_POINT('Ctrl Pts',(-17.2223362244507,1.46449542056432,0.0646144067815574));
#57725=CARTESIAN_POINT('Ctrl Pts',(-17.2488507668564,1.4858899766675,-0.420296482271922));
#57726=CARTESIAN_POINT('Ctrl Pts',(-17.2753653092621,1.24251038228787,-0.916889363924539));
#57727=CARTESIAN_POINT('Ctrl Pts',(-17.3018798516678,0.846150587470515,
-1.19705933091928));
#57728=CARTESIAN_POINT('Ctrl Pts',(-17.3283943940735,0.449790792653172,
-1.47722929791401));
#57729=CARTESIAN_POINT('Ctrl Pts',(-17.3549089364792,-0.0995492026018883,
-1.54097635025084));
#57730=CARTESIAN_POINT('Ctrl Pts',(-17.3814234788849,-0.549535638992197,
-1.35901892551025));
#57731=CARTESIAN_POINT('Ctrl Pts',(-17.4079380212906,-0.999522075382518,
-1.17706150076966));
#57732=CARTESIAN_POINT('Ctrl Pts',(-17.4344525636963,-1.35015495290811,
-0.749399598951582));
#57733=CARTESIAN_POINT('Ctrl Pts',(-17.4609671061019,-1.44037461291437,
-0.272475380336248));
#57734=CARTESIAN_POINT('Ctrl Pts',(-17.465926388787,-1.45724930721892,-0.183271426397507));
#57735=CARTESIAN_POINT('Ctrl Pts',(-17.4708856714721,-1.4650137056991,-0.0923440796015177));
#57736=CARTESIAN_POINT('Ctrl Pts',(-17.4758449541571,-1.46417935052163,
-0.00127487220091121));
#57737=CARTESIAN_POINT('Ctrl Pts',(-17.5471550458428,-1.46460091918832,
-0.00116803120312899));
#57738=CARTESIAN_POINT('Ctrl Pts',(-17.5429767466726,-1.46526876496353,
-0.0778386182632508));
#57739=CARTESIAN_POINT('Ctrl Pts',(-17.5387984475024,-1.45977017776411,
-0.154413201537133));
#57740=CARTESIAN_POINT('Ctrl Pts',(-17.5346201483322,-1.44777151529703,
-0.229955351806808));
#57741=CARTESIAN_POINT('Ctrl Pts',(-17.5081056059265,-1.3716307144987,-0.709328767913805));
#57742=CARTESIAN_POINT('Ctrl Pts',(-17.4815910635208,-1.0337393696746,-1.147127296132));
#57743=CARTESIAN_POINT('Ctrl Pts',(-17.4550765211151,-0.589304445567263,
-1.34225261957826));
#57744=CARTESIAN_POINT('Ctrl Pts',(-17.4285619787094,-0.144869521459913,
-1.53737794302453));
#57745=CARTESIAN_POINT('Ctrl Pts',(-17.4020474363038,0.406108981930661,
-1.48983006169885));
#57746=CARTESIAN_POINT('Ctrl Pts',(-17.3755328938981,0.810544673196106,
-1.22144961299411));
#57747=CARTESIAN_POINT('Ctrl Pts',(-17.3490183514924,1.21498036446153,-0.953069164289384));
#57748=CARTESIAN_POINT('Ctrl Pts',(-17.3225038090867,1.47287324360184,-0.46385614820559));
#57749=CARTESIAN_POINT('Ctrl Pts',(-17.295989266681,1.46576283030811,0.0214743944548562));
#57750=CARTESIAN_POINT('Ctrl Pts',(-17.2694747242753,1.45865241701438,0.506804937115344));
#57751=CARTESIAN_POINT('Ctrl Pts',(-17.2429601818696,1.18653871128658,0.988253006352498));
#57752=CARTESIAN_POINT('Ctrl Pts',(-17.216445639464,0.774414385999632,1.24467031100081));
#57753=CARTESIAN_POINT('Ctrl Pts',(-17.1899310970583,0.362290060712716,
1.5010876156491));
#57754=CARTESIAN_POINT('Ctrl Pts',(-17.1634165546526,-0.189844884133316,
1.53247415570858));
#57755=CARTESIAN_POINT('Ctrl Pts',(-17.1369020122469,-0.628372857468012,
1.32441284210307));
#57756=CARTESIAN_POINT('Ctrl Pts',(-17.1103874698412,-1.06690083080273,
1.11635152849754));
#57757=CARTESIAN_POINT('Ctrl Pts',(-17.0838729274355,-1.3918218326261,0.66884236122699));
#57758=CARTESIAN_POINT('Ctrl Pts',(-17.0573583850298,-1.45388669379952,
0.187444140806682));
#57759=CARTESIAN_POINT('Ctrl Pts',(-17.0539572719675,-1.46184797055169,
0.125693507867038));
#57760=CARTESIAN_POINT('Ctrl Pts',(-17.0505561589052,-1.46548418873406,
0.0633852614001415));
#57761=CARTESIAN_POINT('Ctrl Pts',(-17.0471550458428,-1.46499001420292,
0.00101896910938441));
#57762=CARTESIAN_POINT('Origin',(-17.3,0.,0.));
#57763=CARTESIAN_POINT('',(-16.4758449541571,-1.46159467054894,0.00086381236336773));
#57764=CARTESIAN_POINT('',(-16.5471550458428,-1.46136743550077,0.000666439445737842));
#57765=CARTESIAN_POINT('',(-17.3,-1.4635,-1.79227059055215E-16));
#57766=CARTESIAN_POINT('Ctrl Pts',(-16.4758449541571,-1.46159467054894,
0.00086381236336773));
#57767=CARTESIAN_POINT('Ctrl Pts',(-16.4860444959372,-1.46260248845685,
0.189003976803686));
#57768=CARTESIAN_POINT('Ctrl Pts',(-16.4962440377172,-1.42891868062783,
0.376797030316824));
#57769=CARTESIAN_POINT('Ctrl Pts',(-16.5064435794972,-1.35888007399166,
0.549878898418593));
#57770=CARTESIAN_POINT('Ctrl Pts',(-16.5329581219029,-1.17680899219806,
0.99981935951095));
#57771=CARTESIAN_POINT('Ctrl Pts',(-16.5594726643086,-0.749058537053789,
1.35034420198627));
#57772=CARTESIAN_POINT('Ctrl Pts',(-16.5859872067143,-0.272111544911907,
1.44044339199542));
#57773=CARTESIAN_POINT('Ctrl Pts',(-16.61250174912,0.204835447229961,1.53054258200456));
#57774=CARTESIAN_POINT('Ctrl Pts',(-16.6390162915256,0.730978976369435,
1.36021611954754));
#57775=CARTESIAN_POINT('Ctrl Pts',(-16.6655308339313,1.06464034481988,1.0077017389086));
#57776=CARTESIAN_POINT('Ctrl Pts',(-16.692045376337,1.39830171327034,0.655187358269641));
#57777=CARTESIAN_POINT('Ctrl Pts',(-16.7185599187427,1.53948092103175,0.120485059448733));
#57778=CARTESIAN_POINT('Ctrl Pts',(-16.7450744611484,1.42332872985914,-0.350795075756759));
#57779=CARTESIAN_POINT('Ctrl Pts',(-16.7715890035541,1.30717653868653,-0.822075210962224));
#57780=CARTESIAN_POINT('Ctrl Pts',(-16.7981035459598,0.933692948579942,
-1.22993318255228));
#57781=CARTESIAN_POINT('Ctrl Pts',(-16.8246180883655,0.474433861427808,
-1.38702356488573));
#57782=CARTESIAN_POINT('Ctrl Pts',(-16.8511326307711,0.0151747742756748,
-1.54411394721917));
#57783=CARTESIAN_POINT('Ctrl Pts',(-16.8776471731768,-0.529859809922002,
-1.45043674029601));
#57784=CARTESIAN_POINT('Ctrl Pts',(-16.9041617155825,-0.91031377879697,
-1.14902161970521));
#57785=CARTESIAN_POINT('Ctrl Pts',(-16.9280561284407,-1.2531718250248,-0.877391914658694));
#57786=CARTESIAN_POINT('Ctrl Pts',(-16.9519505412989,-1.46236935454806,
-0.437052444944582));
#57787=CARTESIAN_POINT('Ctrl Pts',(-16.9758449541571,-1.46533423939264,
0.000830137543336423));
#57788=CARTESIAN_POINT('Ctrl Pts',(-17.0471550458428,-1.46499001420292,
0.00101896910938441));
#57789=CARTESIAN_POINT('Ctrl Pts',(-17.0240416164995,-1.4616316818278,-0.4228125424722));
#57790=CARTESIAN_POINT('Ctrl Pts',(-17.0009281871561,-1.267517448972,-0.849324812075515));
#57791=CARTESIAN_POINT('Ctrl Pts',(-16.9778147578128,-0.943744294593583,
-1.12172569318533));
#57792=CARTESIAN_POINT('Ctrl Pts',(-16.9513002154071,-0.572328313690735,
-1.434210033187));
#57793=CARTESIAN_POINT('Ctrl Pts',(-16.9247856730014,-0.0302876313615806,
-1.5438914396203));
#57794=CARTESIAN_POINT('Ctrl Pts',(-16.8982711305957,0.433396858506015,
-1.40038887005259));
#57795=CARTESIAN_POINT('Ctrl Pts',(-16.87175658819,0.897081348373612,-1.25688630048487));
#57796=CARTESIAN_POINT('Ctrl Pts',(-16.8452420457843,1.28240964577962,-0.860199754916109));
#57797=CARTESIAN_POINT('Ctrl Pts',(-16.8187275033787,1.41238510258278,-0.39254317766618));
#57798=CARTESIAN_POINT('Ctrl Pts',(-16.792212960973,1.54236055938594,0.0751133995837501));
#57799=CARTESIAN_POINT('Ctrl Pts',(-16.7656984185673,1.41698317558626,0.61374000851487));
#57800=CARTESIAN_POINT('Ctrl Pts',(-16.7391838761616,1.09384378174213,0.975923975253261));
#57801=CARTESIAN_POINT('Ctrl Pts',(-16.7126693337559,0.770704387898002,
1.33810794199164));
#57802=CARTESIAN_POINT('Ctrl Pts',(-16.6861547913502,0.249802984009428,
1.52384926653732));
#57803=CARTESIAN_POINT('Ctrl Pts',(-16.6596402489445,-0.229589649342414,
1.44782955393405));
#57804=CARTESIAN_POINT('Ctrl Pts',(-16.6331257065389,-0.708982282694284,
1.37180984133078));
#57805=CARTESIAN_POINT('Ctrl Pts',(-16.6066111641332,-1.1468661455094,1.03402909157855));
#57806=CARTESIAN_POINT('Ctrl Pts',(-16.5800966217275,-1.34210372332243,
0.589643468694527));
#57807=CARTESIAN_POINT('Ctrl Pts',(-16.5691160964326,-1.422957887384,0.40560908114604));
#57808=CARTESIAN_POINT('Ctrl Pts',(-16.5581355711377,-1.46219688775553,
0.203291375369544));
#57809=CARTESIAN_POINT('Ctrl Pts',(-16.5471550458428,-1.46136743550077,
0.000666439445737842));
#57810=CARTESIAN_POINT('Origin',(-17.3,0.,0.));
#57811=CARTESIAN_POINT('',(-15.9758449541571,-1.46216976248559,-0.00115783740885875));
#57812=CARTESIAN_POINT('',(-16.0471550458428,-1.46254205711415,-0.00126432517610342));
#57813=CARTESIAN_POINT('',(-17.3,-1.4635,-1.79227059055215E-16));
#57814=CARTESIAN_POINT('Ctrl Pts',(-15.9758449541571,-1.46216976248559,
-0.00115783740885875));
#57815=CARTESIAN_POINT('Ctrl Pts',(-15.9936239081697,-1.45975575237227,
0.326467896832275));
#57816=CARTESIAN_POINT('Ctrl Pts',(-16.0114028621823,-1.35096575277778,
0.655546977160496));
#57817=CARTESIAN_POINT('Ctrl Pts',(-16.0291818161949,-1.14879164530715,
0.910603983128834));
#57818=CARTESIAN_POINT('Ctrl Pts',(-16.0556963586006,-0.847280434801294,
1.29098180489658));
#57819=CARTESIAN_POINT('Ctrl Pts',(-16.0822109010062,-0.338072888959171,
1.50672654371053));
#57820=CARTESIAN_POINT('Ctrl Pts',(-16.1087254434119,0.144931666815352,
1.4587380403526));
#57821=CARTESIAN_POINT('Ctrl Pts',(-16.1352399858176,0.627936222589903,
1.41074953699466));
#57822=CARTESIAN_POINT('Ctrl Pts',(-16.1617545282233,1.08473778829685,1.09902779146479));
#57823=CARTESIAN_POINT('Ctrl Pts',(-16.188269070629,1.30550919437688,0.666759028296608));
#57824=CARTESIAN_POINT('Ctrl Pts',(-16.2147836130347,1.5262806004569,0.234490265128449));
#57825=CARTESIAN_POINT('Ctrl Pts',(-16.2412981554403,1.51102184691004,-0.318325515678011));
#57826=CARTESIAN_POINT('Ctrl Pts',(-16.267812697846,1.26674188753176,-0.737757987954096));
#57827=CARTESIAN_POINT('Ctrl Pts',(-16.2943272402517,1.02246192815349,-1.15719046023018));
#57828=CARTESIAN_POINT('Ctrl Pts',(-16.3208417826574,0.549160762943808,
-1.44323962397589));
#57829=CARTESIAN_POINT('Ctrl Pts',(-16.3473563250631,0.0642444852714359,
-1.46451169491057));
#57830=CARTESIAN_POINT('Ctrl Pts',(-16.3738708674688,-0.420671792400949,
-1.48578376584524));
#57831=CARTESIAN_POINT('Ctrl Pts',(-16.4003854098745,-0.917203182536025,
-1.24227874396888));
#57832=CARTESIAN_POINT('Ctrl Pts',(-16.4268999522802,-1.1972730233821,-0.845848193175995));
#57833=CARTESIAN_POINT('Ctrl Pts',(-16.4432149529058,-1.36960636252544,
-0.601915464288857));
#57834=CARTESIAN_POINT('Ctrl Pts',(-16.4595299535315,-1.45998258344223,
-0.300081756246599));
#57835=CARTESIAN_POINT('Ctrl Pts',(-16.4758449541571,-1.46159467054894,
0.00086381236336773));
#57836=CARTESIAN_POINT('Ctrl Pts',(-16.5471550458428,-1.46136743550077,
0.000666439445737842));
#57837=CARTESIAN_POINT('Ctrl Pts',(-16.531621028732,-1.46019401936885,-0.285984621153708));
#57838=CARTESIAN_POINT('Ctrl Pts',(-16.5160870116212,-1.37882992327694,
-0.573250554372443));
#57839=CARTESIAN_POINT('Ctrl Pts',(-16.5005529945104,-1.22165431091895,
-0.810236119253631));
#57840=CARTESIAN_POINT('Ctrl Pts',(-16.4740384521047,-0.953376027891525,
-1.21473958830201));
#57841=CARTESIAN_POINT('Ctrl Pts',(-16.447523909699,-0.464228169025754,
-1.47275603038295));
#57842=CARTESIAN_POINT('Ctrl Pts',(-16.4210093672934,0.021104154183723,
-1.46576820780307));
#57843=CARTESIAN_POINT('Ctrl Pts',(-16.3944948248877,0.506436477393186,
-1.45878038522319));
#57844=CARTESIAN_POINT('Ctrl Pts',(-16.367980282482,0.987953264946341,-1.1867882979825));
#57845=CARTESIAN_POINT('Ctrl Pts',(-16.3414657400763,1.2444746606157,-0.774728754736447));
#57846=CARTESIAN_POINT('Ctrl Pts',(-16.3149511976706,1.50099605628506,-0.362669211490377));
#57847=CARTESIAN_POINT('Ctrl Pts',(-16.2884366552649,1.5325220600706,0.189457787761057));
#57848=CARTESIAN_POINT('Ctrl Pts',(-16.2619221128592,1.32457152164702,0.628038301675728));
#57849=CARTESIAN_POINT('Ctrl Pts',(-16.2354075704535,1.11662098322344,1.0666188155904));
#57850=CARTESIAN_POINT('Ctrl Pts',(-16.2088930280479,0.669193902590743,
1.3916528441683));
#57851=CARTESIAN_POINT('Ctrl Pts',(-16.1823784856422,0.187811374599038,
1.45383930057667));
#57852=CARTESIAN_POINT('Ctrl Pts',(-16.1558639432365,-0.293571153392639,
1.51602575698503));
#57853=CARTESIAN_POINT('Ctrl Pts',(-16.1293494008308,-0.808909128743352,
1.31536464122387));
#57854=CARTESIAN_POINT('Ctrl Pts',(-16.1028348584251,-1.12148727538583,
0.944027603133352));
#57855=CARTESIAN_POINT('Ctrl Pts',(-16.0842749208977,-1.34028912326836,
0.68409506788046));
#57856=CARTESIAN_POINT('Ctrl Pts',(-16.0657149833703,-1.45974124758651,
0.340533512961544));
#57857=CARTESIAN_POINT('Ctrl Pts',(-16.0471550458428,-1.46254205711415,
-0.00126432517610342));
#57858=CARTESIAN_POINT('Origin',(-17.3,0.,0.));
#57859=CARTESIAN_POINT('',(-15.4758449541571,-1.46579348024391,-0.000392046237105565));
#57860=CARTESIAN_POINT('',(-15.5471550458428,-1.46590607594638,-0.000129214056304876));
#57861=CARTESIAN_POINT('',(-17.3,-1.4635,-1.79227059055215E-16));
#57862=CARTESIAN_POINT('Ctrl Pts',(-15.4758449541571,-1.46579348024391,
-0.000392046237105564));
#57863=CARTESIAN_POINT('Ctrl Pts',(-15.5012033204023,-1.4641396019743,0.463932910653296));
#57864=CARTESIAN_POINT('Ctrl Pts',(-15.5265616866474,-1.22475744536399,
0.929725121980544));
#57865=CARTESIAN_POINT('Ctrl Pts',(-15.5519200528925,-0.845545744914202,
1.19748663945578));
#57866=CARTESIAN_POINT('Ctrl Pts',(-15.5784345952982,-0.449044463439101,
1.47745633628402));
#57867=CARTESIAN_POINT('Ctrl Pts',(-15.6049491377039,0.100327665674265,
1.54092586300297));
#57868=CARTESIAN_POINT('Ctrl Pts',(-15.6314636801096,0.550222122761289,
1.35874113577299));
#57869=CARTESIAN_POINT('Ctrl Pts',(-15.6579782225153,1.0001165798483,1.17655640854301));
#57870=CARTESIAN_POINT('Ctrl Pts',(-15.6844927649209,1.35053336490898,0.748717427364106));
#57871=CARTESIAN_POINT('Ctrl Pts',(-15.7110073073266,1.44051207917245,0.271747692126144));
#57872=CARTESIAN_POINT('Ctrl Pts',(-15.7375218497323,1.53049079343592,-0.205222043111832));
#57873=CARTESIAN_POINT('Ctrl Pts',(-15.764036392138,1.36003143690217,-0.731322532408869));
#57874=CARTESIAN_POINT('Ctrl Pts',(-15.7905509345437,1.00743278740271,-1.06489484799374));
#57875=CARTESIAN_POINT('Ctrl Pts',(-15.8170654769494,0.654834137903267,
-1.3984671635786));
#57876=CARTESIAN_POINT('Ctrl Pts',(-15.8435800193551,0.120096195438124,
-1.5395113054513));
#57877=CARTESIAN_POINT('Ctrl Pts',(-15.8700945617607,-0.35115458564864,
-1.42324007651399));
#57878=CARTESIAN_POINT('Ctrl Pts',(-15.8966091041664,-0.822405366735417,
-1.30696884757667));
#57879=CARTESIAN_POINT('Ctrl Pts',(-15.9231236465721,-1.23016898644384,
-0.933382247829284));
#57880=CARTESIAN_POINT('Ctrl Pts',(-15.9496381889778,-1.38714335871322,
-0.474083495594829));
#57881=CARTESIAN_POINT('Ctrl Pts',(-15.9583737773709,-1.43886077036718,
-0.322761070806314));
#57882=CARTESIAN_POINT('Ctrl Pts',(-15.967109365764,-1.46335587268711,-0.162134886975079));
#57883=CARTESIAN_POINT('Ctrl Pts',(-15.9758449541571,-1.46216976248559,
-0.00115783740885875));
#57884=CARTESIAN_POINT('Ctrl Pts',(-16.0471550458428,-1.46254205711415,
-0.00126432517610342));
#57885=CARTESIAN_POINT('Ctrl Pts',(-16.0392004409646,-1.46374245625874,
-0.14775548370561));
#57886=CARTESIAN_POINT('Ctrl Pts',(-16.0312458360863,-1.44351524001586,
-0.293922666076689));
#57887=CARTESIAN_POINT('Ctrl Pts',(-16.0232912312081,-1.40049829784565,
-0.433043118016538));
#57888=CARTESIAN_POINT('Ctrl Pts',(-15.9967766888024,-1.25711285572868,
-0.896763840655955));
#57889=CARTESIAN_POINT('Ctrl Pts',(-15.9702621463967,-0.860523653560479,
-1.28219232551488));
#57890=CARTESIAN_POINT('Ctrl Pts',(-15.943747603991,-0.392899921956407,
-1.41228590436097));
#57891=CARTESIAN_POINT('Ctrl Pts',(-15.9172330615853,0.074723809647678,
-1.54237948320706));
#57892=CARTESIAN_POINT('Ctrl Pts',(-15.8907185191796,0.613382070687635,
-1.4171381560403));
#57893=CARTESIAN_POINT('Ctrl Pts',(-15.8642039767739,0.975647648214161,
-1.09409025718367));
#57894=CARTESIAN_POINT('Ctrl Pts',(-15.8376894343682,1.33791322574068,-0.77104235832704));
#57895=CARTESIAN_POINT('Ctrl Pts',(-15.8111748919626,1.52378611975377,-0.250187887780555));
#57896=CARTESIAN_POINT('Ctrl Pts',(-15.7846603495569,1.44788750019579,0.229223932229647));
#57897=CARTESIAN_POINT('Ctrl Pts',(-15.7581458071512,1.37198888063781,0.708635752239876));
#57898=CARTESIAN_POINT('Ctrl Pts',(-15.7316312647455,1.03431874750873,1.14660492171382));
#57899=CARTESIAN_POINT('Ctrl Pts',(-15.7051167223398,0.589982454200974,
1.34195474143692));
#57900=CARTESIAN_POINT('Ctrl Pts',(-15.6786021799341,0.145646160893255,
1.53730456116001));
#57901=CARTESIAN_POINT('Ctrl Pts',(-15.6520876375285,-0.405356292593118,
1.49003503113232));
#57902=CARTESIAN_POINT('Ctrl Pts',(-15.6255730951228,-0.809927513616029,
1.22185893089906));
#57903=CARTESIAN_POINT('Ctrl Pts',(-15.5994337453628,-1.20877387073326,
0.957477642547655));
#57904=CARTESIAN_POINT('Ctrl Pts',(-15.5732943956028,-1.46530380969871,
0.478397404464385));
#57905=CARTESIAN_POINT('Ctrl Pts',(-15.5471550458428,-1.46590607594638,
-0.000129214056304876));
#57906=CARTESIAN_POINT('Origin',(-17.3,0.,0.));
#57907=CARTESIAN_POINT('',(-14.9758449541571,-1.46335918983354,0.00135254215526508));
#57908=CARTESIAN_POINT('',(-15.0471550458428,-1.46293148617486,0.00132846867353373));
#57909=CARTESIAN_POINT('',(-17.3,-1.4635,-1.79227059055215E-16));
#57910=CARTESIAN_POINT('Ctrl Pts',(-14.9758449541571,-1.46335918983354,
0.00135254215526508));
#57911=CARTESIAN_POINT('Ctrl Pts',(-14.9822681902291,-1.46444314548935,
0.119474507650463));
#57912=CARTESIAN_POINT('Ctrl Pts',(-14.9886914263011,-1.45134725973014,
0.237359122688176));
#57913=CARTESIAN_POINT('Ctrl Pts',(-14.9951146623731,-1.42315133236242,
0.351514073136027));
#57914=CARTESIAN_POINT('Ctrl Pts',(-15.0216292047788,-1.30676107307877,
0.822735470037065));
#57915=CARTESIAN_POINT('Ctrl Pts',(-15.0481437471844,-0.933071487526462,
1.23040471184739));
#57916=CARTESIAN_POINT('Ctrl Pts',(-15.0746582895901,-0.473733099514172,
1.38726306403735));
#57917=CARTESIAN_POINT('Ctrl Pts',(-15.1011728319958,-0.0143947115018555,
1.54412141622733));
#57918=CARTESIAN_POINT('Ctrl Pts',(-15.1276873744015,0.530592478970439,
1.45016887879692));
#57919=CARTESIAN_POINT('Ctrl Pts',(-15.1542019168072,0.910894129361871,
1.14856159761316));
#57920=CARTESIAN_POINT('Ctrl Pts',(-15.1807164592129,1.29119577975329,0.846954316429403));
#57921=CARTESIAN_POINT('Ctrl Pts',(-15.2072310016186,1.50681189006386,0.337692291492272));
#57922=CARTESIAN_POINT('Ctrl Pts',(-15.2337455440243,1.45870138527481,-0.145300127374153));
#57923=CARTESIAN_POINT('Ctrl Pts',(-15.2602600864299,1.41059088048578,-0.628292546240537));
#57924=CARTESIAN_POINT('Ctrl Pts',(-15.2867746288357,1.09875376059722,-1.08501535903624));
#57925=CARTESIAN_POINT('Ctrl Pts',(-15.3132891712413,0.666429246185057,
-1.30567757055363));
#57926=CARTESIAN_POINT('Ctrl Pts',(-15.339803713647,0.234104731772872,-1.52633978207103));
#57927=CARTESIAN_POINT('Ctrl Pts',(-15.3663182560527,-0.318707177162912,
-1.51094139231009));
#57928=CARTESIAN_POINT('Ctrl Pts',(-15.3928327984584,-0.738077932958183,
-1.266555495546));
#57929=CARTESIAN_POINT('Ctrl Pts',(-15.4193473408641,-1.15744868875347,
-1.02216959878192));
#57930=CARTESIAN_POINT('Ctrl Pts',(-15.4458618832698,-1.44337829140822,
-0.548796195014686));
#57931=CARTESIAN_POINT('Ctrl Pts',(-15.4723764256755,-1.46452787581717,
-0.06387455966231));
#57932=CARTESIAN_POINT('Ctrl Pts',(-15.473532601836,-1.46545011105417,-0.0427293772958018));
#57933=CARTESIAN_POINT('Ctrl Pts',(-15.4746887779966,-1.46586888630947,
-0.021562236805336));
#57934=CARTESIAN_POINT('Ctrl Pts',(-15.4758449541571,-1.46579348024391,
-0.000392046237105564));
#57935=CARTESIAN_POINT('Ctrl Pts',(-15.5471550458428,-1.46590607594638,
-0.000129214056304876));
#57936=CARTESIAN_POINT('Ctrl Pts',(-15.5467798531971,-1.46591472060927,
-0.00699777313276096));
#57937=CARTESIAN_POINT('Ctrl Pts',(-15.5464046605514,-1.46587063787642,
-0.0138662181499694));
#57938=CARTESIAN_POINT('Ctrl Pts',(-15.5460294679057,-1.46577349177823,
-0.0207339125660903));
#57939=CARTESIAN_POINT('Ctrl Pts',(-15.5195149255,-1.45890826035804,-0.506067985359095));
#57940=CARTESIAN_POINT('Ctrl Pts',(-15.4930003830943,-1.18703780895822,
-0.987653460506266));
#57941=CARTESIAN_POINT('Ctrl Pts',(-15.4664858406886,-0.775043074043492,
-1.24427893082992));
#57942=CARTESIAN_POINT('Ctrl Pts',(-15.439971298283,-0.363048339128761,
-1.50090440115358));
#57943=CARTESIAN_POINT('Ctrl Pts',(-15.4134567558773,0.189070679300894,
-1.53256986665373));
#57944=CARTESIAN_POINT('Ctrl Pts',(-15.3869422134716,0.627703705812936,
-1.3247301166799));
#57945=CARTESIAN_POINT('Ctrl Pts',(-15.3604276710659,1.06633673232499,-1.11689036670607));
#57946=CARTESIAN_POINT('Ctrl Pts',(-15.3339131286602,1.39148376691944,-0.66954540125823));
#57947=CARTESIAN_POINT('Ctrl Pts',(-15.3073985862545,1.45379181459511,-0.188178596408585));
#57948=CARTESIAN_POINT('Ctrl Pts',(-15.2808840438488,1.51609986227078,0.293188208441046));
#57949=CARTESIAN_POINT('Ctrl Pts',(-15.2543695014432,1.31556892302771,0.808576852692463));
#57950=CARTESIAN_POINT('Ctrl Pts',(-15.2278549590375,0.944310851441779,
1.1212487860325));
#57951=CARTESIAN_POINT('Ctrl Pts',(-15.2013404166318,0.573052779855828,
1.43392071937255));
#57952=CARTESIAN_POINT('Ctrl Pts',(-15.1748258742261,0.0310675759269861,
1.54387594180115));
#57953=CARTESIAN_POINT('Ctrl Pts',(-15.1483113318204,-0.432689349897711,
1.40060763628332));
#57954=CARTESIAN_POINT('Ctrl Pts',(-15.1217967894147,-0.896446275722394,
1.25733933076549));
#57955=CARTESIAN_POINT('Ctrl Pts',(-15.095282247009,-1.28197492344295,0.860847497301233));
#57956=CARTESIAN_POINT('Ctrl Pts',(-15.0687677046033,-1.41218661603166,
0.393256641178603));
#57957=CARTESIAN_POINT('Ctrl Pts',(-15.0615634850165,-1.44756620553502,
0.266208353761034));
#57958=CARTESIAN_POINT('Ctrl Pts',(-15.0543592654297,-1.46409692728797,
0.133911154947905));
#57959=CARTESIAN_POINT('Ctrl Pts',(-15.0471550458428,-1.46293148617486,
0.00132846867353373));
#57960=CARTESIAN_POINT('Origin',(-17.3,0.,0.));
#57961=CARTESIAN_POINT('',(-14.4758449541571,-1.4611077494086,-0.000226779192605414));
#57962=CARTESIAN_POINT('',(-14.5471550458428,-1.46120820448801,-0.00045760858243725));
#57963=CARTESIAN_POINT('',(-17.3,-1.4635,-1.79227059055215E-16));
#57964=CARTESIAN_POINT('Ctrl Pts',(-14.4758449541571,-1.4611077494086,-0.000226779192605414));
#57965=CARTESIAN_POINT('Ctrl Pts',(-14.4898476024617,-1.46075141589656,
0.258280404757669));
#57966=CARTESIAN_POINT('Ctrl Pts',(-14.5038502507662,-1.39548808866609,
0.516955705114966));
#57967=CARTESIAN_POINT('Ctrl Pts',(-14.5178528990707,-1.26636902275068,
0.738397830871059));
#57968=CARTESIAN_POINT('Ctrl Pts',(-14.5443674414764,-1.02187720419323,
1.15770684342856));
#57969=CARTESIAN_POINT('Ctrl Pts',(-14.5708819838821,-0.548431592070911,
1.44351686674928));
#57970=CARTESIAN_POINT('Ctrl Pts',(-14.5973965262878,-0.0635046299778209,
1.46454396328311));
#57971=CARTESIAN_POINT('Ctrl Pts',(-14.6239110686935,0.42142233211527,1.48557105981693));
#57972=CARTESIAN_POINT('Ctrl Pts',(-14.6504256110992,0.917830644179146,
1.24181522956387));
#57973=CARTESIAN_POINT('Ctrl Pts',(-14.6769401535048,1.19770017912673,0.845243242704368));
#57974=CARTESIAN_POINT('Ctrl Pts',(-14.7034546959105,1.47756971407433,0.448671255844851));
#57975=CARTESIAN_POINT('Ctrl Pts',(-14.7299692383162,1.54090047190564,-0.100716887621091));
#57976=CARTESIAN_POINT('Ctrl Pts',(-14.7564837807219,1.35860211086313,-0.550565311998352));
#57977=CARTESIAN_POINT('Ctrl Pts',(-14.7829983231276,1.17630374982063,-1.00041373637563));
#57978=CARTESIAN_POINT('Ctrl Pts',(-14.8095128655333,0.748376269904274,
-1.35072244166419));
#57979=CARTESIAN_POINT('Ctrl Pts',(-14.836027407939,0.271383822002094,-1.44058067444109));
#57980=CARTESIAN_POINT('Ctrl Pts',(-14.8625419503447,-0.20560862590006,
-1.53043890721798));
#57981=CARTESIAN_POINT('Ctrl Pts',(-14.8890564927503,-0.731666041788053,
-1.35984666748324));
#57982=CARTESIAN_POINT('Ctrl Pts',(-14.915571035156,-1.06514928322455,-1.00716377162));
#57983=CARTESIAN_POINT('Ctrl Pts',(-14.9356623414897,-1.31784510042325,
-0.739919480127962));
#57984=CARTESIAN_POINT('Ctrl Pts',(-14.9557536478234,-1.45996867376205,
-0.368122371564781));
#57985=CARTESIAN_POINT('Ctrl Pts',(-14.9758449541571,-1.46335918983354,
0.00135254215526508));
#57986=CARTESIAN_POINT('Ctrl Pts',(-15.0471550458428,-1.46293148617486,
0.00132846867353373));
#57987=CARTESIAN_POINT('Ctrl Pts',(-15.027844723024,-1.45980761635813,-0.354048604622195));
#57988=CARTESIAN_POINT('Ctrl Pts',(-15.0085344002051,-1.32954313637262,
-0.711476803367705));
#57989=CARTESIAN_POINT('Ctrl Pts',(-14.9892240773863,-1.09433666281944,
-0.975371258926184));
#57990=CARTESIAN_POINT('Ctrl Pts',(-14.9627095349806,-0.771380279561598,
-1.33771842412738));
#57991=CARTESIAN_POINT('Ctrl Pts',(-14.9361949925749,-0.250572775588987,
-1.52372287574874));
#57992=CARTESIAN_POINT('Ctrl Pts',(-14.9096804501692,0.228858200491881,
-1.44794535407855));
#57993=CARTESIAN_POINT('Ctrl Pts',(-14.8831659077635,0.708289176572695,
-1.37216783240837));
#57994=CARTESIAN_POINT('Ctrl Pts',(-14.8566513653579,1.1463436247618,-1.03460833744674));
#57995=CARTESIAN_POINT('Ctrl Pts',(-14.8301368229522,1.34180567393118,-0.590321402065126));
#57996=CARTESIAN_POINT('Ctrl Pts',(-14.8036222805465,1.53726772310058,-0.146034466683465));
#57997=CARTESIAN_POINT('Ctrl Pts',(-14.7771077381408,1.4901373732502,0.404979909118181));
#57998=CARTESIAN_POINT('Ctrl Pts',(-14.7505931957351,1.22206347292139,0.809618856302988));
#57999=CARTESIAN_POINT('Ctrl Pts',(-14.7240786533294,0.9539895725926,1.21425780348776));
#58000=CARTESIAN_POINT('Ctrl Pts',(-14.6975641109237,0.464972121785394,
1.47252132205572));
#58001=CARTESIAN_POINT('Ctrl Pts',(-14.671049568518,-0.0203636696255808,
1.46577868223324));
#58002=CARTESIAN_POINT('Ctrl Pts',(-14.6445350261124,-0.50569946103657,
1.45903604241077));
#58003=CARTESIAN_POINT('Ctrl Pts',(-14.6180204837067,-0.987353593051334,
1.18728724419787));
#58004=CARTESIAN_POINT('Ctrl Pts',(-14.591505941301,-1.24408312165593,0.775357343900782));
#58005=CARTESIAN_POINT('Ctrl Pts',(-14.5767223094816,-1.38722701491958,
0.545678856970483));
#58006=CARTESIAN_POINT('Ctrl Pts',(-14.5619386776622,-1.46044615101826,
0.27242074658531));
#58007=CARTESIAN_POINT('Ctrl Pts',(-14.5471550458428,-1.46120820448801,
-0.00045760858243725));
#58008=CARTESIAN_POINT('Origin',(-17.3,0.,0.));
#58009=CARTESIAN_POINT('',(-13.9758449541571,-1.46419415654471,-0.00127194797176891));
#58010=CARTESIAN_POINT('',(-14.0471550458428,-1.46461493246388,-0.00116358319217421));
#58011=CARTESIAN_POINT('',(-17.3,-1.4635,-1.79227059055215E-16));
#58012=CARTESIAN_POINT('Ctrl Pts',(-13.9758449541571,-1.46419415654471,
-0.00127194797176891));
#58013=CARTESIAN_POINT('Ctrl Pts',(-13.9974270146942,-1.46056726591937,
0.395037360005112));
#58014=CARTESIAN_POINT('Ctrl Pts',(-14.0190090752313,-1.29403678955949,
0.794030585412455));
#58015=CARTESIAN_POINT('Ctrl Pts',(-14.0405911357684,-1.00689469157767,
1.06540365049606));
#58016=CARTESIAN_POINT('Ctrl Pts',(-14.0671056781741,-0.654127571852718,
1.39879779650711));
#58017=CARTESIAN_POINT('Ctrl Pts',(-14.0936202205797,-0.119318444454299,
1.53957177961409));
#58018=CARTESIAN_POINT('Ctrl Pts',(-14.1201347629854,0.351873538195867,
1.42306249741012));
#58019=CARTESIAN_POINT('Ctrl Pts',(-14.1466493053911,0.82306552084606,1.30655321520615));
#58020=CARTESIAN_POINT('Ctrl Pts',(-14.1731638477968,1.23064035874799,0.932760667691196));
#58021=CARTESIAN_POINT('Ctrl Pts',(-14.1996783902025,1.38738268085055,0.473382673208));
#58022=CARTESIAN_POINT('Ctrl Pts',(-14.2261929326082,1.5441250029531,0.0140046787248296));
#58023=CARTESIAN_POINT('Ctrl Pts',(-14.2527074750139,1.4500348092563,-0.530958762726577));
#58024=CARTESIAN_POINT('Ctrl Pts',(-14.2792220174195,1.14833147663801,-0.911184217477438));
#58025=CARTESIAN_POINT('Ctrl Pts',(-14.3057365598252,0.846628144019725,
-1.2914096722283));
#58026=CARTESIAN_POINT('Ctrl Pts',(-14.3322511022309,0.337311672479953,
-1.50689714027861));
#58027=CARTESIAN_POINT('Ctrl Pts',(-14.3587656446366,-0.14566857866218,
-1.45866463712813));
#58028=CARTESIAN_POINT('Ctrl Pts',(-14.3852801870423,-0.628648829804313,
-1.41043213397765));
#58029=CARTESIAN_POINT('Ctrl Pts',(-14.411794729448,-1.08529286054881,-1.09847965962638));
#58030=CARTESIAN_POINT('Ctrl Pts',(-14.4383092718537,-1.30584586342477,
-0.666099421553594));
#58031=CARTESIAN_POINT('Ctrl Pts',(-14.4508211659548,-1.40992217647036,
-0.462064380426998));
#58032=CARTESIAN_POINT('Ctrl Pts',(-14.463333060056,-1.46142614683388,-0.231212692687603));
#58033=CARTESIAN_POINT('Ctrl Pts',(-14.4758449541571,-1.4611077494086,-0.000226779192605414));
#58034=CARTESIAN_POINT('Ctrl Pts',(-14.5471550458428,-1.46120820448801,
-0.00045760858243725));
#58035=CARTESIAN_POINT('Ctrl Pts',(-14.5354241352565,-1.46181289900589,
-0.216988405920967));
#58036=CARTESIAN_POINT('Ctrl Pts',(-14.5236932246702,-1.41679478498902,
-0.433280089304781));
#58037=CARTESIAN_POINT('Ctrl Pts',(-14.5119623140839,-1.32488862719155,
-0.627369069901061));
#58038=CARTESIAN_POINT('Ctrl Pts',(-14.4854477716782,-1.11715967892816,
-1.06605458102458));
#58039=CARTESIAN_POINT('Ctrl Pts',(-14.4589332292726,-0.669896857206923,
-1.39131460089034));
#58040=CARTESIAN_POINT('Ctrl Pts',(-14.4324186868669,-0.188545806211767,
-1.45374423585788));
#58041=CARTESIAN_POINT('Ctrl Pts',(-14.4059041444612,0.292805244783348,
-1.5161738708254));
#58042=CARTESIAN_POINT('Ctrl Pts',(-14.3793896020555,0.808244525052368,
-1.31577312089478));
#58043=CARTESIAN_POINT('Ctrl Pts',(-14.3528750596498,1.12101022514064,-0.944594039500663));
#58044=CARTESIAN_POINT('Ctrl Pts',(-14.3263605172441,1.43377592522893,-0.573414958106515));
#58045=CARTESIAN_POINT('Ctrl Pts',(-14.2998459748384,1.5438680451364,-0.031457545248834));
#58046=CARTESIAN_POINT('Ctrl Pts',(-14.2733314324327,1.40071688535858,0.43233555417222));
#58047=CARTESIAN_POINT('Ctrl Pts',(-14.2468168900271,1.25756572558076,0.896128653593288));
#58048=CARTESIAN_POINT('Ctrl Pts',(-14.2203023476214,0.861171286117661,
1.28175743957772));
#58049=CARTESIAN_POINT('Ctrl Pts',(-14.1937878052157,0.393613335309966,
1.41208723760121));
#58050=CARTESIAN_POINT('Ctrl Pts',(-14.16727326281,-0.0739446154976886,
1.54241703562468));
#58051=CARTESIAN_POINT('Ctrl Pts',(-14.1407587204043,-0.612666077649932,
1.41744784568724));
#58052=CARTESIAN_POINT('Ctrl Pts',(-14.1142441779986,-0.975094807407056,
1.09458299863365));
#58053=CARTESIAN_POINT('Ctrl Pts',(-14.0918811339467,-1.28077647919425,
0.822270518674362));
#58054=CARTESIAN_POINT('Ctrl Pts',(-14.0695180898948,-1.46104936176178,
0.40918164700796));
#58055=CARTESIAN_POINT('Ctrl Pts',(-14.0471550458428,-1.46461493246388,
-0.00116358319217421));
#58056=CARTESIAN_POINT('Origin',(-17.3,0.,0.));
#58057=CARTESIAN_POINT('',(-13.4758449541571,-1.46532338661684,0.000837209389326979));
#58058=CARTESIAN_POINT('',(-13.5471550458428,-1.46497727491618,0.00102478181900469));
#58059=CARTESIAN_POINT('',(-17.3,-1.4635,-1.79227059055215E-16));
#58060=CARTESIAN_POINT('Ctrl Pts',(-13.4758449541571,-1.46532338661684,
0.000837209389326979));
#58061=CARTESIAN_POINT('Ctrl Pts',(-13.4784918845211,-1.46565405334147,
0.0493450887578976));
#58062=CARTESIAN_POINT('Ctrl Pts',(-13.481138814885,-1.4634549955769,0.0978226187749106));
#58063=CARTESIAN_POINT('Ctrl Pts',(-13.4837857452489,-1.45862779591486,
0.146037020656259));
#58064=CARTESIAN_POINT('Ctrl Pts',(-13.5103002876546,-1.41027329748027,
0.629005073258751));
#58065=CARTESIAN_POINT('Ctrl Pts',(-13.5368148300603,-1.09820548856963,
1.08557029281694));
#58066=CARTESIAN_POINT('Ctrl Pts',(-13.563329372466,-0.665769554423191,
1.3060140729796));
#58067=CARTESIAN_POINT('Ctrl Pts',(-13.5898439148717,-0.233333620276776,
1.52645785314224));
#58068=CARTESIAN_POINT('Ctrl Pts',(-13.6163584572774,0.319470439105424,
1.51078019390938));
#58069=CARTESIAN_POINT('Ctrl Pts',(-13.6428729996831,0.73871768167217,1.26618246915778));
#58070=CARTESIAN_POINT('Ctrl Pts',(-13.6693875420888,1.15796492423892,1.02158474440618));
#58071=CARTESIAN_POINT('Ctrl Pts',(-13.6959020844944,1.44365534999021,0.548066954135844));
#58072=CARTESIAN_POINT('Ctrl Pts',(-13.7224166269001,1.46455995730734,0.0631346962416146));
#58073=CARTESIAN_POINT('Ctrl Pts',(-13.7489311693058,1.48546456462448,-0.421797561652615));
#58074=CARTESIAN_POINT('Ctrl Pts',(-13.7754457117115,1.24158335350746,-0.918144287170734));
#58075=CARTESIAN_POINT('Ctrl Pts',(-13.8019602541172,0.844940686565861,
-1.1979136423813));
#58076=CARTESIAN_POINT('Ctrl Pts',(-13.8284747965229,0.448298019624239,
-1.47768299759187));
#58077=CARTESIAN_POINT('Ctrl Pts',(-13.8549893389286,-0.101106103141984,
-1.54087498249487));
#58078=CARTESIAN_POINT('Ctrl Pts',(-13.8815038813343,-0.550908466108,-1.35846299927092));
#58079=CARTESIAN_POINT('Ctrl Pts',(-13.9080184237399,-1.00071082907399,
-1.17605101604698));
#58080=CARTESIAN_POINT('Ctrl Pts',(-13.9345329661456,-1.35091143223979,
-0.748035064696129));
#58081=CARTESIAN_POINT('Ctrl Pts',(-13.9610475085513,-1.44064917779694,
-0.271019934563134));
#58082=CARTESIAN_POINT('Ctrl Pts',(-13.9659799904199,-1.45734302814206,
-0.18228114192513));
#58083=CARTESIAN_POINT('Ctrl Pts',(-13.9709124722885,-1.46502306591684,
-0.0918466395122355));
#58084=CARTESIAN_POINT('Ctrl Pts',(-13.9758449541571,-1.46419415654471,
-0.00127194797176891));
#58085=CARTESIAN_POINT('Ctrl Pts',(-14.0471550458428,-1.46461493246388,
-0.00116358319217421));
#58086=CARTESIAN_POINT('Ctrl Pts',(-14.0430035474891,-1.46527684865318,
-0.0773404911163755));
#58087=CARTESIAN_POINT('Ctrl Pts',(-14.0388520491353,-1.45984897336895,
-0.153422846052185));
#58088=CARTESIAN_POINT('Ctrl Pts',(-14.0347005507816,-1.44800311557867,
-0.228492454152207));
#58089=CARTESIAN_POINT('Ctrl Pts',(-14.0081860083759,-1.37234669663114,
-0.70794255571478));
#58090=CARTESIAN_POINT('Ctrl Pts',(-13.9816714659702,-1.03489786137402,
-1.14608225467017));
#58091=CARTESIAN_POINT('Ctrl Pts',(-13.9551569235645,-0.590660312265092,
-1.34165652081483));
#58092=CARTESIAN_POINT('Ctrl Pts',(-13.9286423811588,-0.146422763156193,
-1.53723078695948));
#58093=CARTESIAN_POINT('Ctrl Pts',(-13.9021278387531,0.4046034998045,-1.49023962029342));
#58094=CARTESIAN_POINT('Ctrl Pts',(-13.8756132963474,0.809310147334135,
-1.22226793697292));
#58095=CARTESIAN_POINT('Ctrl Pts',(-13.8490987539418,1.21401679486377,-0.954296253652418));
#58096=CARTESIAN_POINT('Ctrl Pts',(-13.8225842115361,1.47240382696235,-0.465344053677463));
#58097=CARTESIAN_POINT('Ctrl Pts',(-13.7960696691304,1.46578377916778,0.0199934253858157));
#58098=CARTESIAN_POINT('Ctrl Pts',(-13.7695551267247,1.45916373137321,0.505330904449067));
#58099=CARTESIAN_POINT('Ctrl Pts',(-13.743040584319,1.18753660368553,0.987053662600641));
#58100=CARTESIAN_POINT('Ctrl Pts',(-13.7165260419133,0.775671564288337,
1.24388723310617));
#58101=CARTESIAN_POINT('Ctrl Pts',(-13.6900114995076,0.363806524891071,
1.50072080361175));
#58102=CARTESIAN_POINT('Ctrl Pts',(-13.663496957102,-0.188296426215764,
1.53266518647119));
#58103=CARTESIAN_POINT('Ctrl Pts',(-13.6369824146963,-0.62703439396149,
1.32504705317184));
#58104=CARTESIAN_POINT('Ctrl Pts',(-13.6104678722906,-1.06577236170717,
1.11742891987252));
#58105=CARTESIAN_POINT('Ctrl Pts',(-13.5839533298849,-1.39114534609176,
0.67024827041447));
#58106=CARTESIAN_POINT('Ctrl Pts',(-13.5574387874792,-1.45369656436799,
0.18891300398528));
#58107=CARTESIAN_POINT('Ctrl Pts',(-13.5540108736004,-1.46178345442188,
0.126683914193862));
#58108=CARTESIAN_POINT('Ctrl Pts',(-13.5505829597216,-1.46547742885513,
0.0638839494987724));
#58109=CARTESIAN_POINT('Ctrl Pts',(-13.5471550458428,-1.46497727491618,
0.00102478181900469));
#58110=CARTESIAN_POINT('Origin',(-17.3,0.,0.));
#58111=CARTESIAN_POINT('',(-12.9758449541571,-1.46158588710458,0.000857444751660996));
#58112=CARTESIAN_POINT('',(-13.0471550458428,-1.46136072574925,0.000659268984059629));
#58113=CARTESIAN_POINT('',(-17.3,-1.4635,-1.79227059055215E-16));
#58114=CARTESIAN_POINT('Ctrl Pts',(-12.9758449541571,-1.46158588710458,
0.000857444751660996));
#58115=CARTESIAN_POINT('Ctrl Pts',(-12.9860712967536,-1.46258854316142,
0.18949481438138));
#58116=CARTESIAN_POINT('Ctrl Pts',(-12.9962976393501,-1.42872174436519,
0.377785957761628));
#58117=CARTESIAN_POINT('Ctrl Pts',(-13.0065239819466,-1.35832380100528,
0.551251585068185));
#58118=CARTESIAN_POINT('Ctrl Pts',(-13.0330385243523,-1.17579820723828,
1.00100785792437));
#58119=CARTESIAN_POINT('Ctrl Pts',(-13.059553066758,-0.747693811761432,
1.35110033662373));
#58120=CARTESIAN_POINT('Ctrl Pts',(-13.0860676091637,-0.270656029832401,
1.44071758923565));
#58121=CARTESIAN_POINT('Ctrl Pts',(-13.1125821515694,0.206381752096632,
1.53033484184757));
#58122=CARTESIAN_POINT('Ctrl Pts',(-13.139096693975,0.732352920477846,1.35947686837204));
#58123=CARTESIAN_POINT('Ctrl Pts',(-13.1656112363807,1.06565794979205,1.00662554729284));
#58124=CARTESIAN_POINT('Ctrl Pts',(-13.1921257787864,1.39896297910629,0.653774226213604));
#58125=CARTESIAN_POINT('Ctrl Pts',(-13.2186403211921,1.53960186935347,0.118929557530643));
#58126=CARTESIAN_POINT('Ctrl Pts',(-13.2451548635978,1.42297357166271,-0.352232980805425));
#58127=CARTESIAN_POINT('Ctrl Pts',(-13.2716694060035,1.30634527397197,-0.823395519141413));
#58128=CARTESIAN_POINT('Ctrl Pts',(-13.2981839484092,0.932449788343379,
-1.23087592713053));
#58129=CARTESIAN_POINT('Ctrl Pts',(-13.3246984908148,0.473032216698865,
-1.38750220914511));
#58130=CARTESIAN_POINT('Ctrl Pts',(-13.3512130332205,0.0136146450543249,
-1.5441284911597));
#58131=CARTESIAN_POINT('Ctrl Pts',(-13.3777275756262,-0.531325012606148,
-1.44990064719972));
#58132=CARTESIAN_POINT('Ctrl Pts',(-13.4042421180319,-0.911474247457094,
-1.14810128239635));
#58133=CARTESIAN_POINT('Ctrl Pts',(-13.4281097300736,-1.25367341938933,
-0.876430361459512));
#58134=CARTESIAN_POINT('Ctrl Pts',(-13.4519773421154,-1.46234173466025,
-0.436562754549332));
#58135=CARTESIAN_POINT('Ctrl Pts',(-13.4758449541571,-1.46532338661684,
0.000837209389326979));
#58136=CARTESIAN_POINT('Ctrl Pts',(-13.5471550458428,-1.46497727491618,
0.00102478181900469));
#58137=CARTESIAN_POINT('Ctrl Pts',(-13.5240684173159,-1.46160879233375,
-0.422324901121936));
#58138=CARTESIAN_POINT('Ctrl Pts',(-13.500981788789,-1.26799982481547,-0.848359958356493));
#58139=CARTESIAN_POINT('Ctrl Pts',(-13.4778951602621,-0.944877167291941,
-1.12077159272548));
#58140=CARTESIAN_POINT('Ctrl Pts',(-13.4513806178565,-0.573777099771778,
-1.43363103960672));
#58141=CARTESIAN_POINT('Ctrl Pts',(-13.4248660754508,-0.0318475125635945,
-1.54386004996886));
#58142=CARTESIAN_POINT('Ctrl Pts',(-13.3983515330451,0.431981730862603,
-1.40082604506448));
#58143=CARTESIAN_POINT('Ctrl Pts',(-13.3718369906394,0.895810974288801,
-1.2577920401601));
#58144=CARTESIAN_POINT('Ctrl Pts',(-13.3453224482337,1.28153987393298,-0.861495019989192));
#58145=CARTESIAN_POINT('Ctrl Pts',(-13.318807905828,1.41198776907589,-0.3939700043279));
#58146=CARTESIAN_POINT('Ctrl Pts',(-13.2922933634223,1.54243566421881,0.0735550113334183));
#58147=CARTESIAN_POINT('Ctrl Pts',(-13.2657788210166,1.41760255486038,0.612308022485182));
#58148=CARTESIAN_POINT('Ctrl Pts',(-13.239264278611,1.0948292646106,0.974818293674386));
#58149=CARTESIAN_POINT('Ctrl Pts',(-13.2127497362053,0.772055974360851,
1.33732856486357));
#58150=CARTESIAN_POINT('Ctrl Pts',(-13.1862351937996,0.251342503219808,
1.52359609609029));
#58151=CARTESIAN_POINT('Ctrl Pts',(-13.1597206513939,-0.228126693234285,
1.44806078469242));
#58152=CARTESIAN_POINT('Ctrl Pts',(-13.1332061089882,-0.707595889688351,
1.37252547329456));
#58153=CARTESIAN_POINT('Ctrl Pts',(-13.1066915665825,-1.14582081145544,
1.03518731927217));
#58154=CARTESIAN_POINT('Ctrl Pts',(-13.0801770241769,-1.34150728209725,
0.590999184779553));
#58155=CARTESIAN_POINT('Ctrl Pts',(-13.0691696980655,-1.42274514639728,
0.406597599553718));
#58156=CARTESIAN_POINT('Ctrl Pts',(-13.0581623719542,-1.46218303840703,
0.203781094128016));
#58157=CARTESIAN_POINT('Ctrl Pts',(-13.0471550458428,-1.46136072574925,
0.000659268984059629));
#58158=CARTESIAN_POINT('Origin',(-17.3,0.,0.));
#58159=CARTESIAN_POINT('',(-12.4758449541571,-1.46218187472528,-0.00116212229894885));
#58160=CARTESIAN_POINT('',(-12.5471550458428,-1.46255548750974,-0.00126727998485326));
#58161=CARTESIAN_POINT('',(-17.3,-1.4635,-1.79227059055215E-16));
#58162=CARTESIAN_POINT('Ctrl Pts',(-12.4758449541571,-1.46218187472528,
-0.00116212229894885));
#58163=CARTESIAN_POINT('Ctrl Pts',(-12.4936507089862,-1.45975393531768,
0.326950644416945));
#58164=CARTESIAN_POINT('Ctrl Pts',(-12.5114564638152,-1.35060787521459,
0.656527436918317));
#58165=CARTESIAN_POINT('Ctrl Pts',(-12.5292622186442,-1.14787101490285,
0.911764219282333));
#58166=CARTESIAN_POINT('Ctrl Pts',(-12.5557767610499,-0.845975637169948,
1.29183720997888));
#58167=CARTESIAN_POINT('Ctrl Pts',(-12.5822913034556,-0.336550369915331,
1.50706735227095));
#58168=CARTESIAN_POINT('Ctrl Pts',(-12.6088058458613,0.146405453332879,
1.45859086163736));
#58169=CARTESIAN_POINT('Ctrl Pts',(-12.635320388267,0.62936127658109,1.41011437100376));
#58170=CARTESIAN_POINT('Ctrl Pts',(-12.6618349306727,1.08584765582289,1.09793124744451));
#58171=CARTESIAN_POINT('Ctrl Pts',(-12.6883494730784,1.30618219920735,0.665439644814965));
#58172=CARTESIAN_POINT('Ctrl Pts',(-12.714864015484,1.52651674259176,0.232948042185496));
#58173=CARTESIAN_POINT('Ctrl Pts',(-12.7413785578897,1.51069945011893,-0.319852039514211));
#58174=CARTESIAN_POINT('Ctrl Pts',(-12.7678931002954,1.26599583477921,-0.739037485341109));
#58175=CARTESIAN_POINT('Ctrl Pts',(-12.7944076427011,1.02129221943944,-1.15822293116808));
#58176=CARTESIAN_POINT('Ctrl Pts',(-12.8209221851068,0.547702281232709,
-1.44379374112219));
#58177=CARTESIAN_POINT('Ctrl Pts',(-12.8474367275125,0.0627647584772496,
-1.46457585788886));
#58178=CARTESIAN_POINT('Ctrl Pts',(-12.8739512699182,-0.42217276427821,
-1.48535797465554));
#58179=CARTESIAN_POINT('Ctrl Pts',(-12.9004658123239,-0.918457871582393,
-1.24135139823478));
#58180=CARTESIAN_POINT('Ctrl Pts',(-12.9269803547296,-1.19812702920591,
-0.844638076517884));
#58181=CARTESIAN_POINT('Ctrl Pts',(-12.9432685545387,-1.36993113014577,
-0.600932348837367));
#58182=CARTESIAN_POINT('Ctrl Pts',(-12.9595567543479,-1.45998888778252,
-0.299598279180735));
#58183=CARTESIAN_POINT('Ctrl Pts',(-12.9758449541571,-1.46158588710458,
0.000857444751660996));
#58184=CARTESIAN_POINT('Ctrl Pts',(-13.0471550458428,-1.46136072574925,
0.000659268984059629));
#58185=CARTESIAN_POINT('Ctrl Pts',(-13.0316478295485,-1.46020224455984,
-0.285500516303598));
#58186=CARTESIAN_POINT('Ctrl Pts',(-13.0161406132541,-1.3791376512242,-0.572266282406523));
#58187=CARTESIAN_POINT('Ctrl Pts',(-13.0006333969598,-1.2224723230406,-0.809001386729198));
#58188=CARTESIAN_POINT('Ctrl Pts',(-12.9741188545541,-0.954602873825676,
-1.21377570878235));
#58189=CARTESIAN_POINT('Ctrl Pts',(-12.9476043121484,-0.465715955879361,
-1.4722862379258));
#58190=CARTESIAN_POINT('Ctrl Pts',(-12.9210897697427,0.0196231798704193,
-1.46578878258152));
#58191=CARTESIAN_POINT('Ctrl Pts',(-12.894575227337,0.5049623156202,-1.45929132723724));
#58192=CARTESIAN_POINT('Ctrl Pts',(-12.8680606849314,0.986753669173477,
-1.18778588740522));
#58193=CARTESIAN_POINT('Ctrl Pts',(-12.8415461425257,1.24369126519327,-0.775985735185896));
#58194=CARTESIAN_POINT('Ctrl Pts',(-12.81503160012,1.50062886121308,-0.364185582966545));
#58195=CARTESIAN_POINT('Ctrl Pts',(-12.7885170577143,1.53271269969942,0.187909281640078));
#58196=CARTESIAN_POINT('Ctrl Pts',(-12.7620025153086,1.32520539461077,0.62669967801535));
#58197=CARTESIAN_POINT('Ctrl Pts',(-12.7354879729029,1.11769808952214,1.0654900743906));
#58198=CARTESIAN_POINT('Ctrl Pts',(-12.7089734304972,0.670599640858534,
1.39097600253446));
#58199=CARTESIAN_POINT('Ctrl Pts',(-12.6824588880916,0.189280189705736,
1.45364880012849));
#58200=CARTESIAN_POINT('Ctrl Pts',(-12.6559443456859,-0.292039261447089,
1.51632159772253));
#58201=CARTESIAN_POINT('Ctrl Pts',(-12.6294298032802,-0.807579715089139,
1.31618126476671));
#58202=CARTESIAN_POINT('Ctrl Pts',(-12.6029152608745,-1.12053288880213,
0.945160234797672));
#58203=CARTESIAN_POINT('Ctrl Pts',(-12.5843285225306,-1.3399135842971,0.685073875448221));
#58204=CARTESIAN_POINT('Ctrl Pts',(-12.5657417841867,-1.45974221525453,
0.341016172077363));
#58205=CARTESIAN_POINT('Ctrl Pts',(-12.5471550458428,-1.46255548750974,
-0.00126727998485326));
#58206=CARTESIAN_POINT('Origin',(-17.3,0.,0.));
#58207=CARTESIAN_POINT('',(-11.9758449541571,-1.46579906277062,-0.000383257489619121));
#58208=CARTESIAN_POINT('',(-12.0471550458428,-1.4659079907007,-0.000120015143960721));
#58209=CARTESIAN_POINT('',(-17.3,-1.4635,-1.79227059055215E-16));
#58210=CARTESIAN_POINT('Ctrl Pts',(-11.9758449541571,-1.46579906277062,
-0.000383257489619121));
#58211=CARTESIAN_POINT('Ctrl Pts',(-12.0012301212187,-1.46417694847208,
0.464427706910453));
#58212=CARTESIAN_POINT('Ctrl Pts',(-12.0266152882803,-1.22421852479684,
0.930679514285422));
#58213=CARTESIAN_POINT('Ctrl Pts',(-12.0520004553419,-0.844335412579876,
1.19834033958687));
#58214=CARTESIAN_POINT('Ctrl Pts',(-12.0785149977476,-0.44755146139907,
1.47790928177972));
#58215=CARTESIAN_POINT('Ctrl Pts',(-12.1050295401533,0.10188451480633,1.54082370873951));
#58216=CARTESIAN_POINT('Ctrl Pts',(-12.1315440825589,0.55159466885709,1.35818451607506));
#58217=CARTESIAN_POINT('Ctrl Pts',(-12.1580586249646,1.00130482290782,1.17554532341062));
#58218=CARTESIAN_POINT('Ctrl Pts',(-12.1845731673703,1.35128915480393,0.747352511121983));
#58219=CARTESIAN_POINT('Ctrl Pts',(-12.211087709776,1.44078590875282,0.270292107833193));
#58220=CARTESIAN_POINT('Ctrl Pts',(-12.2376022521817,1.53028266270173,-0.206768295455678));
#58221=CARTESIAN_POINT('Ctrl Pts',(-12.2641167945874,1.35929183870333,-0.732696289744717));
#58222=CARTESIAN_POINT('Ctrl Pts',(-12.2906313369931,1.00635633878264,-1.06591218109636));
#58223=CARTESIAN_POINT('Ctrl Pts',(-12.3171458793988,0.653420838862003,
-1.39912807244797));
#58224=CARTESIAN_POINT('Ctrl Pts',(-12.3436604218044,0.118540663019128,
-1.53963186086222));
#58225=CARTESIAN_POINT('Ctrl Pts',(-12.3701749642101,-0.352592400941366,
-1.42288455512596));
#58226=CARTESIAN_POINT('Ctrl Pts',(-12.3966895066158,-0.823725464901861,
-1.3061372493897));
#58227=CARTESIAN_POINT('Ctrl Pts',(-12.4232040490215,-1.23111141697998,
-0.932138849502929));
#58228=CARTESIAN_POINT('Ctrl Pts',(-12.4497185914272,-1.38762164891344,
-0.472681730009051));
#58229=CARTESIAN_POINT('Ctrl Pts',(-12.4584273790038,-1.43902794296241,
-0.321771546720627));
#58230=CARTESIAN_POINT('Ctrl Pts',(-12.4671361665805,-1.46336937892,-0.161641945476957));
#58231=CARTESIAN_POINT('Ctrl Pts',(-12.4758449541571,-1.46218187472528,
-0.00116212229894885));
#58232=CARTESIAN_POINT('Ctrl Pts',(-12.5471550458428,-1.46255548750974,
-0.00126727998485326));
#58233=CARTESIAN_POINT('Ctrl Pts',(-12.539227241781,-1.46375543291163,-0.147261487862684));
#58234=CARTESIAN_POINT('Ctrl Pts',(-12.5312994377192,-1.4436670130256,-0.292932909822579));
#58235=CARTESIAN_POINT('Ctrl Pts',(-12.5233716336574,-1.40093511539405,
-0.431627879991432));
#58236=CARTESIAN_POINT('Ctrl Pts',(-12.4968570912518,-1.25801827448904,
-0.895493237829282));
#58237=CARTESIAN_POINT('Ctrl Pts',(-12.4703425488461,-0.861818698895064,
-1.28132222652273));
#58238=CARTESIAN_POINT('Ctrl Pts',(-12.4438280064404,-0.394326648209448,
-1.41188821046213));
#58239=CARTESIAN_POINT('Ctrl Pts',(-12.4173134640347,0.0731654024761946,
-1.54245419440153));
#58240=CARTESIAN_POINT('Ctrl Pts',(-12.390798921629,0.611949928253461,-1.41775717358684));
#58241=CARTESIAN_POINT('Ctrl Pts',(-12.3642843792233,0.974541717745663,
-1.09507546073473));
#58242=CARTESIAN_POINT('Ctrl Pts',(-12.3377698368176,1.33713350723782,-0.772393747882646));
#58243=CARTESIAN_POINT('Ctrl Pts',(-12.3112552944119,1.52353256044495,-0.251727342993118));
#58244=CARTESIAN_POINT('Ctrl Pts',(-12.2847407520063,1.44811836141617,0.227760917761126));
#58245=CARTESIAN_POINT('Ctrl Pts',(-12.2582262096006,1.37270416238738,0.707249178515397));
#58246=CARTESIAN_POINT('Ctrl Pts',(-12.2317116671949,1.0354767111227,1.14555929513442));
#58247=CARTESIAN_POINT('Ctrl Pts',(-12.2051971247892,0.591338019586661,
1.34135795778807));
#58248=CARTESIAN_POINT('Ctrl Pts',(-12.1786825823835,0.147199328050593,
1.53715662044173));
#58249=CARTESIAN_POINT('Ctrl Pts',(-12.1521680399778,-0.403850603756823,
1.49044382912997));
#58250=CARTESIAN_POINT('Ctrl Pts',(-12.1256534975721,-0.808692574507879,
1.22267663111137));
#58251=CARTESIAN_POINT('Ctrl Pts',(-12.0994873469957,-1.20821506311994,
0.958427800579785));
#58252=CARTESIAN_POINT('Ctrl Pts',(-12.0733211964193,-1.46534659092428,
0.478895553643603));
#58253=CARTESIAN_POINT('Ctrl Pts',(-12.0471550458428,-1.4659079907007,-0.000120015143960721));
#58254=CARTESIAN_POINT('Origin',(-17.3,0.,0.));
#58255=CARTESIAN_POINT('',(-11.4758449541571,-1.4633442613986,0.00135246097216248));
#58256=CARTESIAN_POINT('',(-11.5471550458429,-1.46291715073871,0.0013268560893039));
#58257=CARTESIAN_POINT('',(-17.3,-1.4635,-1.79227059055215E-16));
#58258=CARTESIAN_POINT('Ctrl Pts',(-11.4758449541571,-1.4633442613986,0.00135246097216248));
#58259=CARTESIAN_POINT('Ctrl Pts',(-11.4822949910456,-1.46443170060753,
0.119970375014325));
#58260=CARTESIAN_POINT('Ctrl Pts',(-11.488745027934,-1.45122482725057,0.238349204626237));
#58261=CARTESIAN_POINT('Ctrl Pts',(-11.4951950648225,-1.42279544780548,
0.352951798581079));
#58262=CARTESIAN_POINT('Ctrl Pts',(-11.5217096072281,-1.30592914147246,
0.824055358106536));
#58263=CARTESIAN_POINT('Ctrl Pts',(-11.5482241496338,-0.931827851189581,
1.23134682828133));
#58264=CARTESIAN_POINT('Ctrl Pts',(-11.5747386920395,-0.472331213160919,
1.38774100014792));
#58265=CARTESIAN_POINT('Ctrl Pts',(-11.6012532344452,-0.0128345751322309,
1.54413517201451));
#58266=CARTESIAN_POINT('Ctrl Pts',(-11.6277677768509,0.532057410642251,
1.44963204557287));
#58267=CARTESIAN_POINT('Ctrl Pts',(-11.6542823192566,0.912054132934719,
1.14764067417215));
#58268=CARTESIAN_POINT('Ctrl Pts',(-11.6807968616623,1.29205085522717,0.84564930277145));
#58269=CARTESIAN_POINT('Ctrl Pts',(-11.707311404068,1.50715231403762,0.336169686411701));
#58270=CARTESIAN_POINT('Ctrl Pts',(-11.7338259464736,1.45855383429798,-0.146773876668371));
#58271=CARTESIAN_POINT('Ctrl Pts',(-11.7603404888793,1.40995535455835,-0.629717439748443));
#58272=CARTESIAN_POINT('Ctrl Pts',(-11.786855031285,1.09765693626862,-1.08612494954884));
#58273=CARTESIAN_POINT('Ctrl Pts',(-11.8133695736907,0.665109692750116,
-1.30635024209722));
#58274=CARTESIAN_POINT('Ctrl Pts',(-11.8398841160964,0.232562449231607,
-1.52657553464559));
#58275=CARTESIAN_POINT('Ctrl Pts',(-11.8663986585021,-0.320233619515688,
-1.51061860994196));
#58276=CARTESIAN_POINT('Ctrl Pts',(-11.8929132009078,-0.739357241857687,
-1.26580911962673));
#58277=CARTESIAN_POINT('Ctrl Pts',(-11.9194277433135,-1.15848086419971,
-1.02099962931149));
#58278=CARTESIAN_POINT('Ctrl Pts',(-11.9459422857191,-1.44393204013642,
-0.547337573384642));
#58279=CARTESIAN_POINT('Ctrl Pts',(-11.9724568281248,-1.46459166502666,
-0.0623948167082485));
#58280=CARTESIAN_POINT('Ctrl Pts',(-11.9735862034689,-1.46547165271841,
-0.041738891959084));
#58281=CARTESIAN_POINT('Ctrl Pts',(-11.974715578813,-1.46587122994957,-0.0210625006707822));
#58282=CARTESIAN_POINT('Ctrl Pts',(-11.9758449541571,-1.46579906277062,
-0.000383257489619121));
#58283=CARTESIAN_POINT('Ctrl Pts',(-12.0471550458428,-1.4659079907007,-0.000120015143960721));
#58284=CARTESIAN_POINT('Ctrl Pts',(-12.0468066540136,-1.46591546551418,
-0.00649791585064298));
#58285=CARTESIAN_POINT('Ctrl Pts',(-12.0464582621843,-1.46587745594124,
-0.01287572496136));
#58286=CARTESIAN_POINT('Ctrl Pts',(-12.0461098703551,-1.46579369247414,
-0.0192529331030128));
#58287=CARTESIAN_POINT('Ctrl Pts',(-12.0195953279494,-1.4594188299947,-0.50459369457341));
#58288=CARTESIAN_POINT('Ctrl Pts',(-11.9930807855437,-1.18803509534114,
-0.986453612788815));
#58289=CARTESIAN_POINT('Ctrl Pts',(-11.966566243138,-0.776299856573628,
-1.24349521792961));
#58290=CARTESIAN_POINT('Ctrl Pts',(-11.9400517007323,-0.364564617806093,
-1.50053682307042));
#58291=CARTESIAN_POINT('Ctrl Pts',(-11.9135371583266,0.187522125075435,
-1.5327601151366));
#58292=CARTESIAN_POINT('Ctrl Pts',(-11.8870226159209,0.6263649220843,-1.3253636514981));
#58293=CARTESIAN_POINT('Ctrl Pts',(-11.8605080735153,1.06520771909314,-1.11796718785961));
#58294=CARTESIAN_POINT('Ctrl Pts',(-11.8339935311096,1.39080657022936,-0.670950968516453));
#58295=CARTESIAN_POINT('Ctrl Pts',(-11.8074789887039,1.45360094314246,-0.189647363349462));
#58296=CARTESIAN_POINT('Ctrl Pts',(-11.7809644462982,1.51639531605555,0.291656241817557));
#58297=CARTESIAN_POINT('Ctrl Pts',(-11.7544499038925,1.31638521074554,0.807247232808381));
#58298=CARTESIAN_POINT('Ctrl Pts',(-11.7279353614868,0.945443241999734,
1.12029411338589));
#58299=CARTESIAN_POINT('Ctrl Pts',(-11.7014208190811,0.574501273253951,
1.43334099396338));
#58300=CARTESIAN_POINT('Ctrl Pts',(-11.6749062766755,0.0326274410723951,
1.54384376412751));
#58301=CARTESIAN_POINT('Ctrl Pts',(-11.6483917342698,-0.431274001581286,
1.40104409634033));
#58302=CARTESIAN_POINT('Ctrl Pts',(-11.6218771918641,-0.895175444234968,
1.25824442855316));
#58303=CARTESIAN_POINT('Ctrl Pts',(-11.5953626494584,-1.2811044973608,0.862142322814663));
#58304=CARTESIAN_POINT('Ctrl Pts',(-11.5688481070527,-1.41178856176624,
0.394683266931935));
#58305=CARTESIAN_POINT('Ctrl Pts',(-11.5616170866494,-1.44742859362655,
0.26719828457506));
#58306=CARTESIAN_POINT('Ctrl Pts',(-11.5543860662461,-1.46408460799211,
0.134406081117774));
#58307=CARTESIAN_POINT('Ctrl Pts',(-11.5471550458429,-1.46291715073871,
0.0013268560893039));
#58308=CARTESIAN_POINT('Origin',(-17.3,0.,0.));
#58309=CARTESIAN_POINT('',(-10.9758449541571,-1.46111006519219,-0.000234854365275122));
#58310=CARTESIAN_POINT('',(-11.0471550458429,-1.46121285057659,-0.000465323571519086));
#58311=CARTESIAN_POINT('',(-17.3,-1.4635,-1.79227059055215E-16));
#58312=CARTESIAN_POINT('Ctrl Pts',(-10.9758449541571,-1.46111006519219,
-0.000234854365275122));
#58313=CARTESIAN_POINT('Ctrl Pts',(-10.9898744032781,-1.4607403045662,0.258766084230319));
#58314=CARTESIAN_POINT('Ctrl Pts',(-11.0039038523991,-1.39521262116459,
0.51794180976467));
#58315=CARTESIAN_POINT('Ctrl Pts',(-11.0179333015201,-1.2656223237124,0.739676951201287));
#58316=CARTESIAN_POINT('Ctrl Pts',(-11.0444478439258,-1.0207069740412,1.15873872331721));
#58317=CARTESIAN_POINT('Ctrl Pts',(-11.0709623863315,-0.546972830615103,
1.44407024702402));
#58318=CARTESIAN_POINT('Ctrl Pts',(-11.0974769287372,-0.0620248709583785,
1.4646073787197));
#58319=CARTESIAN_POINT('Ctrl Pts',(-11.1239914711428,0.422923088698319,
1.48514451041539));
#58320=CARTESIAN_POINT('Ctrl Pts',(-11.1505060135485,0.919084864585646,
1.24088725009997));
#58321=CARTESIAN_POINT('Ctrl Pts',(-11.1770205559542,1.19855357351062,0.844032694771085));
#58322=CARTESIAN_POINT('Ctrl Pts',(-11.2035350983599,1.47802228243559,0.447178139442197));
#58323=CARTESIAN_POINT('Ctrl Pts',(-11.2300496407656,1.5407979243982,-0.102273710900164));
#58324=CARTESIAN_POINT('Ctrl Pts',(-11.2565641831713,1.35804514448916,-0.551937717452828));
#58325=CARTESIAN_POINT('Ctrl Pts',(-11.283078725577,1.1752923645801,-1.00160172400552));
#58326=CARTESIAN_POINT('Ctrl Pts',(-11.3095932679827,0.747011162799363,
-1.3514778867685));
#58327=CARTESIAN_POINT('Ctrl Pts',(-11.3361078103883,0.269928168588406,
-1.44085413634418));
#58328=CARTESIAN_POINT('Ctrl Pts',(-11.362622352794,-0.207154825622524,
-1.53023038591984));
#58329=CARTESIAN_POINT('Ctrl Pts',(-11.3891368951997,-0.733039612263668,
-1.35910672230823));
#58330=CARTESIAN_POINT('Ctrl Pts',(-11.4156514376054,-1.06616634439266,
-1.00608706606436));
#58331=CARTESIAN_POINT('Ctrl Pts',(-11.4357159431226,-1.31825529439125,
-0.738944426677143));
#58332=CARTESIAN_POINT('Ctrl Pts',(-11.4557804486399,-1.459961500899,-0.367639194719911));
#58333=CARTESIAN_POINT('Ctrl Pts',(-11.4758449541571,-1.4633442613986,0.00135246097216248));
#58334=CARTESIAN_POINT('Ctrl Pts',(-11.5471550458429,-1.46291715073871,
0.0013268560893039));
#58335=CARTESIAN_POINT('Ctrl Pts',(-11.5278715238405,-1.45980380208567,
-0.3535658175273));
#58336=CARTESIAN_POINT('Ctrl Pts',(-11.5085880018381,-1.32993523721296,
-0.710499702984862));
#58337=CARTESIAN_POINT('Ctrl Pts',(-11.4893044798357,-1.09532158699014,
-0.974265079638717));
#58338=CARTESIAN_POINT('Ctrl Pts',(-11.46278993743,-0.772731472123592,-1.3369383642996));
#58339=CARTESIAN_POINT('Ctrl Pts',(-11.4362753950243,-0.252112166705467,
-1.52346892759434));
#58340=CARTESIAN_POINT('Ctrl Pts',(-11.4097608526186,0.227395127756395,
-1.44817584574619));
#58341=CARTESIAN_POINT('Ctrl Pts',(-11.3832463102129,0.706902422218231,
-1.37288276389804));
#58342=CARTESIAN_POINT('Ctrl Pts',(-11.3567317678072,1.14529770572381,-1.03576603690705));
#58343=CARTESIAN_POINT('Ctrl Pts',(-11.3302172254015,1.3412085478968,-0.591676816664797));
#58344=CARTESIAN_POINT('Ctrl Pts',(-11.3037026829959,1.53711939006979,-0.147587596422573));
#58345=CARTESIAN_POINT('Ctrl Pts',(-11.2771881405902,1.49054579091022,0.403474117070884));
#58346=CARTESIAN_POINT('Ctrl Pts',(-11.2506735981845,1.22288086117226,0.808383710689811));
#58347=CARTESIAN_POINT('Ctrl Pts',(-11.2241590557788,0.955215931434269,
1.21329330430878));
#58348=CARTESIAN_POINT('Ctrl Pts',(-11.1976445133731,0.466459671117826,
1.47205077805319));
#58349=CARTESIAN_POINT('Ctrl Pts',(-11.1711299709674,-0.0188826851072191,
1.46579850884533));
#58350=CARTESIAN_POINT('Ctrl Pts',(-11.1446154285617,-0.504225041332237,
1.45954623963746));
#58351=CARTESIAN_POINT('Ctrl Pts',(-11.118100886156,-0.986153493465858,
1.18828422747734));
#58352=CARTESIAN_POINT('Ctrl Pts',(-11.0915863437504,-1.24329909132773,
0.776613928431419));
#58353=CARTESIAN_POINT('Ctrl Pts',(-11.0767759111145,-1.38693489301208,
0.546664071522495));
#58354=CARTESIAN_POINT('Ctrl Pts',(-11.0619654784787,-1.46043640562047,
0.272905555750272));
#58355=CARTESIAN_POINT('Ctrl Pts',(-11.0471550458429,-1.46121285057659,
-0.000465323571519086));
#58356=CARTESIAN_POINT('Origin',(-17.3,0.,0.));
#58357=CARTESIAN_POINT('',(-10.4758449541571,-1.46420894404091,-0.00126897030766321));
#58358=CARTESIAN_POINT('',(-10.5471550458429,-1.4646289090495,-0.00115908444552544));
#58359=CARTESIAN_POINT('',(-17.3,-1.4635,-1.79227059055215E-16));
#58360=CARTESIAN_POINT('Ctrl Pts',(-10.4758449541571,-1.46420894404091,
-0.00126897030766321));
#58361=CARTESIAN_POINT('Ctrl Pts',(-10.4974538155107,-1.46058180138299,
0.395522140978942));
#58362=CARTESIAN_POINT('Ctrl Pts',(-10.5190626768642,-1.29359078311601,
0.795000998625229));
#58363=CARTESIAN_POINT('Ctrl Pts',(-10.5406715382178,-1.00581772915512,
1.06642043966479));
#58364=CARTESIAN_POINT('Ctrl Pts',(-10.5671860806234,-0.652713939111602,
1.39945799131682));
#58365=CARTESIAN_POINT('Ctrl Pts',(-10.5937006230291,-0.117762851331239,
1.53969154918036));
#58366=CARTESIAN_POINT('Ctrl Pts',(-10.6202151654348,0.353311173701554,
1.42270624970696));
#58367=CARTESIAN_POINT('Ctrl Pts',(-10.6467297078405,0.824385198734346,
1.30572095023355));
#58368=CARTESIAN_POINT('Ctrl Pts',(-10.6732442502462,1.23158216101957,0.931516793423203));
#58369=CARTESIAN_POINT('Ctrl Pts',(-10.6997587926519,1.38786026284093,0.471980666176833));
#58370=CARTESIAN_POINT('Ctrl Pts',(-10.7262733350576,1.54413836466229,0.0124445389304362));
#58371=CARTESIAN_POINT('Ctrl Pts',(-10.7527878774632,1.44949760601975,-0.532423558751993));
#58372=CARTESIAN_POINT('Ctrl Pts',(-10.7793024198689,1.14741026021906,-0.912343988395626));
#58373=CARTESIAN_POINT('Ctrl Pts',(-10.8058169622746,0.845322914418391,
-1.29226441803924));
#58374=CARTESIAN_POINT('Ctrl Pts',(-10.8323315046803,0.335788981459602,
-1.50723717964407));
#58375=CARTESIAN_POINT('Ctrl Pts',(-10.858846047086,-0.147142290639309,
-1.4585167138991));
#58376=CARTESIAN_POINT('Ctrl Pts',(-10.8853605894917,-0.630073562738247,
-1.40979624815412));
#58377=CARTESIAN_POINT('Ctrl Pts',(-10.9118751318974,-1.0864021739773,-1.09738255505932));
#58378=CARTESIAN_POINT('Ctrl Pts',(-10.938389674303,-1.30651820163863,-0.664779698249398));
#58379=CARTESIAN_POINT('Ctrl Pts',(-10.9508747675877,-1.41016581873719,
-0.461076879627928));
#58380=CARTESIAN_POINT('Ctrl Pts',(-10.9633598608724,-1.46143912272459,
-0.230725078985094));
#58381=CARTESIAN_POINT('Ctrl Pts',(-10.9758449541571,-1.46111006519219,
-0.000234854365275122));
#58382=CARTESIAN_POINT('Ctrl Pts',(-11.0471550458429,-1.46121285057659,
-0.000465323571519086));
#58383=CARTESIAN_POINT('Ctrl Pts',(-11.035450936073,-1.46182644487326,-0.216499713527323));
#58384=CARTESIAN_POINT('Ctrl Pts',(-11.0237468263032,-1.41702231000271,
-0.432292019592519));
#58385=CARTESIAN_POINT('Ctrl Pts',(-11.0120427165333,-1.32552182382382,
-0.62603012618947));
#58386=CARTESIAN_POINT('Ctrl Pts',(-10.9855281741276,-1.11823621486794,
-1.0649252958326));
#58387=CARTESIAN_POINT('Ctrl Pts',(-10.9590136317219,-0.671302253366116,
-1.39063704918714));
#58388=CARTESIAN_POINT('Ctrl Pts',(-10.9324990893162,-0.19001452489336,
-1.4535529934129));
#58389=CARTESIAN_POINT('Ctrl Pts',(-10.9059845469106,0.291273203579423,
-1.51646893763866));
#58390=CARTESIAN_POINT('Ctrl Pts',(-10.8794700045049,0.806914699023168,
-1.31658907273557));
#58391=CARTESIAN_POINT('Ctrl Pts',(-10.8529554620992,1.12005526649198,-0.945726188880069));
#58392=CARTESIAN_POINT('Ctrl Pts',(-10.8264409196935,1.4331958339608,-0.574863305024572));
#58393=CARTESIAN_POINT('Ctrl Pts',(-10.7999263772878,1.54383547345474,-0.0330174022166808));
#58394=CARTESIAN_POINT('Ctrl Pts',(-10.7734118348821,1.40115298789638,0.430920095654743));
#58395=CARTESIAN_POINT('Ctrl Pts',(-10.7468972924764,1.25847050233803,0.89485759352614));
#58396=CARTESIAN_POINT('Ctrl Pts',(-10.7203827500707,0.862465891727416,
1.28088668646104));
#58397=CARTESIAN_POINT('Ctrl Pts',(-10.6938682076651,0.395039860472687,
1.41168882299456));
#58398=CARTESIAN_POINT('Ctrl Pts',(-10.6673536652594,-0.0723861707820682,
1.54249095952808));
#58399=CARTESIAN_POINT('Ctrl Pts',(-10.6408391228537,-0.611233622681002,
1.41806613966014));
#58400=CARTESIAN_POINT('Ctrl Pts',(-10.614324580448,-0.973988379371074,
1.09556764336126));
#58401=CARTESIAN_POINT('Ctrl Pts',(-10.5919347355796,-1.28031170199486,
0.8232381725396));
#58402=CARTESIAN_POINT('Ctrl Pts',(-10.5695448907112,-1.46106810598496,
0.409667742333545));
#58403=CARTESIAN_POINT('Ctrl Pts',(-10.5471550458429,-1.4646289090495,-0.00115908444552544));
#58404=CARTESIAN_POINT('Origin',(-17.3,0.,0.));
#58405=CARTESIAN_POINT('',(-9.97584495415713,-1.46531245936081,0.000844241415329933));
#58406=CARTESIAN_POINT('',(-10.0471550458429,-1.46496448118167,0.00103054806325355));
#58407=CARTESIAN_POINT('',(-17.3,-1.4635,-1.79227059055215E-16));
#58408=CARTESIAN_POINT('Ctrl Pts',(-9.97584495415713,-1.46531245936081,
0.000844241415329933));
#58409=CARTESIAN_POINT('Ctrl Pts',(-9.97851868533753,-1.46564870303239,
0.0498442363565879));
#58410=CARTESIAN_POINT('Ctrl Pts',(-9.98119241651793,-1.46340478166659,
0.098813062229553));
#58411=CARTESIAN_POINT('Ctrl Pts',(-9.98386614769833,-1.45847950044308,
0.147510695222105));
#58412=CARTESIAN_POINT('Ctrl Pts',(-10.010380690104,-1.40963705180129,0.630429645527651));
#58413=CARTESIAN_POINT('Ctrl Pts',(-10.0368952325097,-1.09710810383422,
1.08667932909043));
#58414=CARTESIAN_POINT('Ctrl Pts',(-10.0634097749154,-0.664449661334089,
1.30668607782077));
#58415=CARTESIAN_POINT('Ctrl Pts',(-10.0899243173211,-0.231791218834003,
1.52669282655109));
#58416=CARTESIAN_POINT('Ctrl Pts',(-10.1164388597268,0.320996718199095,
1.51045664044901));
#58417=CARTESIAN_POINT('Ctrl Pts',(-10.1429534021325,0.739996613351653,
1.26543544704805));
#58418=CARTESIAN_POINT('Ctrl Pts',(-10.1694679445381,1.15899650850421,1.02041425364709));
#58419=CARTESIAN_POINT('Ctrl Pts',(-10.1959824869438,1.4442083617762,0.546608052947263));
#58420=CARTESIAN_POINT('Ctrl Pts',(-10.2224970293495,1.46462299896701,0.0616549212511626));
#58421=CARTESIAN_POINT('Ctrl Pts',(-10.2490115717552,1.48503763615782,-0.42329821044491));
#58422=CARTESIAN_POINT('Ctrl Pts',(-10.2755261141609,1.24065505726743,-0.919398273137288));
#58423=CARTESIAN_POINT('Ctrl Pts',(-10.3020406565666,0.843729923110822,
-1.19876673096354));
#58424=CARTESIAN_POINT('Ctrl Pts',(-10.3285551989723,0.446804788954149,
-1.47813518878984));
#58425=CARTESIAN_POINT('Ctrl Pts',(-10.355069741378,-0.102662900468787,
-1.54077204175001));
#58426=CARTESIAN_POINT('Ctrl Pts',(-10.3815842837836,-0.552280730833664,
-1.35790568625639));
#58427=CARTESIAN_POINT('Ctrl Pts',(-10.4080988261893,-1.00189856119844,
-1.17503933076282));
#58428=CARTESIAN_POINT('Ctrl Pts',(-10.434613368595,-1.35166653250518,-0.746669766815594));
#58429=CARTESIAN_POINT('Ctrl Pts',(-10.4611279110007,-1.44092227200526,
-0.269564212121746));
#58430=CARTESIAN_POINT('Ctrl Pts',(-10.4660335920528,-1.45743623567702,
-0.181290854666609));
#58431=CARTESIAN_POINT('Ctrl Pts',(-10.470939273105,-1.46503238423608,-0.0913491741857221));
#58432=CARTESIAN_POINT('Ctrl Pts',(-10.4758449541571,-1.46420894404091,
-0.00126897030766321));
#58433=CARTESIAN_POINT('Ctrl Pts',(-10.5471550458429,-1.4646289090495,-0.00115908444552544));
#58434=CARTESIAN_POINT('Ctrl Pts',(-10.5430303483055,-1.46528488660171,
-0.0768423422186303));
#58435=CARTESIAN_POINT('Ctrl Pts',(-10.5389056507682,-1.45992725800098,
-0.152432488479017));
#58436=CARTESIAN_POINT('Ctrl Pts',(-10.5347809532309,-1.44823323767887,
-0.227029323243103));
#58437=CARTESIAN_POINT('Ctrl Pts',(-10.5082664108253,-1.37306127781532,
-0.706555620818703));
#58438=CARTESIAN_POINT('Ctrl Pts',(-10.4817518684196,-1.03605529660695,
-1.14503604324013));
#58439=CARTESIAN_POINT('Ctrl Pts',(-10.4552373260139,-0.592015575992571,
-1.3410590524329));
#58440=CARTESIAN_POINT('Ctrl Pts',(-10.4287227836082,-0.147975855378186,
-1.53708206162567));
#58441=CARTESIAN_POINT('Ctrl Pts',(-10.4022082412025,0.403097604642181,
-1.49064765758984));
#58442=CARTESIAN_POINT('Ctrl Pts',(-10.3756936987968,0.808074795294769,
-1.22308501321018));
#58443=CARTESIAN_POINT('Ctrl Pts',(-10.3491791563911,1.21305198594738,-0.955522368830519));
#58444=CARTESIAN_POINT('Ctrl Pts',(-10.3226646139855,1.47193290723213,-0.466831484106978));
#58445=CARTESIAN_POINT('Ctrl Pts',(-10.2961500715798,1.46580323169478,0.0185124359065781));
#58446=CARTESIAN_POINT('Ctrl Pts',(-10.2696355291741,1.45967355615742,0.503856355920134));
#58447=CARTESIAN_POINT('Ctrl Pts',(-10.2431209867684,1.18853328379795,0.985853311223747));
#58448=CARTESIAN_POINT('Ctrl Pts',(-10.2166064443627,0.776927950739231,
1.24310288540015));
#58449=CARTESIAN_POINT('Ctrl Pts',(-10.190091901957,0.365322617680536,1.50035245957654));
#58450=CARTESIAN_POINT('Ctrl Pts',(-10.1635773595513,-0.186747776077338,
1.53285465262578));
#58451=CARTESIAN_POINT('Ctrl Pts',(-10.1370628171456,-0.625695290352148,
1.3256799115779));
#58452=CARTESIAN_POINT('Ctrl Pts',(-10.11054827474,-1.06464280462698,1.11850517053001));
#58453=CARTESIAN_POINT('Ctrl Pts',(-10.0840337323343,-1.39046743941869,
0.671653495384919));
#58454=CARTESIAN_POINT('Ctrl Pts',(-10.0575191899286,-1.4535049509429,0.190381674313756));
#58455=CARTESIAN_POINT('Ctrl Pts',(-10.0540644752333,-1.46171842919503,
0.127674318960563));
#58456=CARTESIAN_POINT('Ctrl Pts',(-10.0506097605381,-1.46547062024338,
0.0643826193112584));
#58457=CARTESIAN_POINT('Ctrl Pts',(-10.0471550458429,-1.46496448118167,
0.00103054806325355));
#58458=CARTESIAN_POINT('Origin',(-17.3,0.,0.));
#58459=CARTESIAN_POINT('',(-9.47584495415713,-1.46157717162269,0.000851046066846911));
#58460=CARTESIAN_POINT('',(-9.54715504584286,-1.46135409027402,0.000652074851629444));
#58461=CARTESIAN_POINT('',(-17.3,-1.4635,-1.79227059055215E-16));
#58462=CARTESIAN_POINT('Ctrl Pts',(-9.47584495415713,-1.46157717162269,
0.000851046066846911));
#58463=CARTESIAN_POINT('Ctrl Pts',(-9.48609809757008,-1.46257459730285,
0.18998561356786));
#58464=CARTESIAN_POINT('Ctrl Pts',(-9.49635124098303,-1.42852426825454,
0.378774872364767));
#58465=CARTESIAN_POINT('Ctrl Pts',(-9.50660438439598,-1.35776614138582,
0.552623708977331));
#58466=CARTESIAN_POINT('Ctrl Pts',(-9.53311892680166,-1.17478622197511,
1.00219533446756));
#58467=CARTESIAN_POINT('Ctrl Pts',(-9.55963346920735,-0.74632832319233,
1.3518550920021));
#58468=CARTESIAN_POINT('Ctrl Pts',(-9.58614801161304,-0.26920023845603,
1.4409903157318));
#58469=CARTESIAN_POINT('Ctrl Pts',(-9.61266255401872,0.207927846280298,
1.5301255394615));
#58470=CARTESIAN_POINT('Ctrl Pts',(-9.63917709642441,0.733726116970183,
1.35873622938633));
#58471=CARTESIAN_POINT('Ctrl Pts',(-9.6656916388301,1.06667446689659,1.00554832807205));
#58472=CARTESIAN_POINT('Ctrl Pts',(-9.69220618123579,1.39962281682299,0.652360426757773));
#58473=CARTESIAN_POINT('Ctrl Pts',(-9.71872072364148,1.53972124598593,0.117373934204458));
#58474=CARTESIAN_POINT('Ctrl Pts',(-9.74523526604717,1.42261696083608,-0.353670526279942));
#58475=CARTESIAN_POINT('Ctrl Pts',(-9.77174980845285,1.30551267568624,-0.824714986764287));
#58476=CARTESIAN_POINT('Ctrl Pts',(-9.79826435085853,0.931205676223611,
-1.23181741517969));
#58477=CARTESIAN_POINT('Ctrl Pts',(-9.82477889326421,0.471630089079157,
-1.38797943698485));
#58478=CARTESIAN_POINT('Ctrl Pts',(-9.8512934356699,0.0120545019346503,
-1.54414145879004));
#58479=CARTESIAN_POINT('Ctrl Pts',(-9.87780797807559,-0.532789672891738,
-1.44936307398492));
#58480=CARTESIAN_POINT('Ctrl Pts',(-9.90432252048128,-0.912633785646623,
-1.14717977305823));
#58481=CARTESIAN_POINT('Ctrl Pts',(-9.92816333170656,-1.25417435039281,
-0.875468690038308));
#58482=CARTESIAN_POINT('Ctrl Pts',(-9.95200414293184,-1.46231428139932,
-0.436073141303719));
#58483=CARTESIAN_POINT('Ctrl Pts',(-9.97584495415713,-1.46531245936081,
0.000844241415329933));
#58484=CARTESIAN_POINT('Ctrl Pts',(-10.0471550458429,-1.46496448118167,
0.00103054806325355));
#58485=CARTESIAN_POINT('Ctrl Pts',(-10.0240952181324,-1.46158606050438,
-0.421837322933612));
#58486=CARTESIAN_POINT('Ctrl Pts',(-10.001035390422,-1.26848154526367,-0.847394996587496));
#58487=CARTESIAN_POINT('Ctrl Pts',(-9.97797556271152,-0.946009075420625,
-1.11981634813565));
#58488=CARTESIAN_POINT('Ctrl Pts',(-9.95146102030583,-0.575225300117436,
-1.4330505825166));
#58489=CARTESIAN_POINT('Ctrl Pts',(-9.92494647790015,-0.0334073612543562,
-1.54382708428126));
#58490=CARTESIAN_POINT('Ctrl Pts',(-9.89843193549447,0.430566162234381,
-1.40126179005523));
#58491=CARTESIAN_POINT('Ctrl Pts',(-9.87191739308878,0.894539685723119,
-1.25869649582921));
#58492=CARTESIAN_POINT('Ctrl Pts',(-9.84540285068308,1.28066879383748,-0.862789405612513));
#58493=CARTESIAN_POINT('Ctrl Pts',(-9.8188883082774,1.41158899415352,-0.395396428808714));
#58494=CARTESIAN_POINT('Ctrl Pts',(-9.79237376587171,1.54250919446956,0.071996547995058));
#58495=CARTESIAN_POINT('Ctrl Pts',(-9.76585922346603,1.41822048698725,0.610875411385968));
#58496=CARTESIAN_POINT('Ctrl Pts',(-9.73934468106035,1.09581362983228,0.973711616960512));
#58497=CARTESIAN_POINT('Ctrl Pts',(-9.71283013865466,0.773406772677265,
1.3365478225351));
#58498=CARTESIAN_POINT('Ctrl Pts',(-9.68631559624897,0.252881765849561,
1.52334137029334));
#58499=CARTESIAN_POINT('Ctrl Pts',(-9.65980105384328,-0.226663504244833,
1.44829053721051));
#58500=CARTESIAN_POINT('Ctrl Pts',(-9.63328651143759,-0.706208774339227,
1.37323970412768));
#58501=CARTESIAN_POINT('Ctrl Pts',(-9.60677196903191,-1.14477430770028,
1.03634449020378));
#58502=CARTESIAN_POINT('Ctrl Pts',(-9.58025742662622,-1.34090947140602,
0.592354297548066));
#58503=CARTESIAN_POINT('Ctrl Pts',(-9.56922329969844,-1.42253186029052,
0.407586102589327));
#58504=CARTESIAN_POINT('Ctrl Pts',(-9.55818917277065,-1.46216919655488,
0.204270774596894));
#58505=CARTESIAN_POINT('Ctrl Pts',(-9.54715504584286,-1.46135409027402,
0.000652074851629444));
#58506=CARTESIAN_POINT('Origin',(-17.3,0.,0.));
#58507=CARTESIAN_POINT('',(-8.97584495415714,-1.46219403757879,-0.00116636394747058));
#58508=CARTESIAN_POINT('',(-9.04715504584287,-1.46256895709697,-0.00127018677453484));
#58509=CARTESIAN_POINT('',(-17.3,-1.4635,-1.79227059055215E-16));
#58510=CARTESIAN_POINT('Ctrl Pts',(-8.97584495415714,-1.46219403757879,
-0.00116636394747058));
#58511=CARTESIAN_POINT('Ctrl Pts',(-8.99367750980264,-1.45975220887188,
0.327433385342918));
#58512=CARTESIAN_POINT('Ctrl Pts',(-9.01151006544813,-1.35024939521357,
0.657507843102589));
#58513=CARTESIAN_POINT('Ctrl Pts',(-9.02934262109362,-1.14694921270435,
0.912923524669222));
#58514=CARTESIAN_POINT('Ctrl Pts',(-9.05585716349931,-0.844669975931715,
1.29269129630033));
#58515=CARTESIAN_POINT('Ctrl Pts',(-9.082371705905,-0.335027507307018,1.50740662235469));
#58516=CARTESIAN_POINT('Ctrl Pts',(-9.10888624831068,0.147879090393584,
1.45844219393227));
#58517=CARTESIAN_POINT('Ctrl Pts',(-9.13540079071637,0.63078568809416,1.40947776550986));
#58518=CARTESIAN_POINT('Ctrl Pts',(-9.16191533312205,1.08695641487064,1.09683358261071));
#58519=CARTESIAN_POINT('Ctrl Pts',(-9.18842987552774,1.30685387063295,0.664119582025169));
#58520=CARTESIAN_POINT('Ctrl Pts',(-9.21494441793343,1.52675132639526,0.231405581439627));
#58521=CARTESIAN_POINT('Ctrl Pts',(-9.24145896033911,1.51037551114339,-0.321378236832304));
#58522=CARTESIAN_POINT('Ctrl Pts',(-9.26797350274479,1.26524848964568,-0.740316228288248));
#58523=CARTESIAN_POINT('Ctrl Pts',(-9.29448804515048,1.02012146814797,-1.15925421974419));
#58524=CARTESIAN_POINT('Ctrl Pts',(-9.32100258755617,0.546243240404423,
-1.44434638438415));
#58525=CARTESIAN_POINT('Ctrl Pts',(-9.34751712996185,0.0612849676102023,
-1.46463852576758));
#58526=CARTESIAN_POINT('Ctrl Pts',(-9.37403167236754,-0.423673305184046,
-1.48493066715101));
#58527=CARTESIAN_POINT('Ctrl Pts',(-9.40054621477323,-0.919711623028967,
-1.24042278527788));
#58528=CARTESIAN_POINT('Ctrl Pts',(-9.42706075717892,-1.19897981193209,
-0.843427097618339));
#58529=CARTESIAN_POINT('Ctrl Pts',(-9.44332215617166,-1.37025530959104,
-0.599949191167883));
#58530=CARTESIAN_POINT('Ctrl Pts',(-9.45958355516439,-1.4599952629048,-0.299114783102133));
#58531=CARTESIAN_POINT('Ctrl Pts',(-9.47584495415713,-1.46157717162269,
0.000851046066846911));
#58532=CARTESIAN_POINT('Ctrl Pts',(-9.54715504584286,-1.46135409027402,
0.000652074851629444));
#58533=CARTESIAN_POINT('Ctrl Pts',(-9.53167463036496,-1.46021053048274,
-0.285016387343409));
#58534=CARTESIAN_POINT('Ctrl Pts',(-9.51619421488706,-1.37944479806305,
-0.571281973384492));
#58535=CARTESIAN_POINT('Ctrl Pts',(-9.50071379940916,-1.22328908721203,
-0.807765828342601));
#58536=CARTESIAN_POINT('Ctrl Pts',(-9.47419925700348,-0.955828745261837,
-1.21281059019021));
#58537=CARTESIAN_POINT('Ctrl Pts',(-9.44768471459779,-0.467203267310972,
-1.47181494249797));
#58538=CARTESIAN_POINT('Ctrl Pts',(-9.42117017219211,0.0181421855248795,
-1.46580786102218));
#58539=CARTESIAN_POINT('Ctrl Pts',(-9.39465562978642,0.503487638360758,
-1.4598007795464));
#58540=CARTESIAN_POINT('Ctrl Pts',(-9.36814108738073,0.985553066081652,
-1.18878226428704));
#58541=CARTESIAN_POINT('Ctrl Pts',(-9.34162654497504,1.24290660015939,-0.777241923477027));
#58542=CARTESIAN_POINT('Ctrl Pts',(-9.31511200256935,1.50026013423713,-0.365701582667018));
#58543=CARTESIAN_POINT('Ctrl Pts',(-9.28859746016367,1.53290177467173,0.186360583693584));
#58544=CARTESIAN_POINT('Ctrl Pts',(-9.26208291775799,1.32583791475006,0.625360414594071));
#58545=CARTESIAN_POINT('Ctrl Pts',(-9.2355683753523,1.11877405482839,1.06436024549453));
#58546=CARTESIAN_POINT('Ctrl Pts',(-9.20905383294662,0.672004694550432,
1.39029774093484));
#58547=CARTESIAN_POINT('Ctrl Pts',(-9.18253929054093,0.190748811587309,
1.45345681573553));
#58548=CARTESIAN_POINT('Ctrl Pts',(-9.15602474813524,-0.290507071375815,
1.51661589053622));
#58549=CARTESIAN_POINT('Ctrl Pts',(-9.12951020572955,-0.806249477024134,
1.31699654469731));
#58550=CARTESIAN_POINT('Ctrl Pts',(-9.10299566332387,-1.11957735833208,
0.946291901603416));
#58551=CARTESIAN_POINT('Ctrl Pts',(-9.08438212416354,-1.33953743531608,
0.686052622887204));
#58552=CARTESIAN_POINT('Ctrl Pts',(-9.0657685850032,-1.45974328379025,0.341498832192847));
#58553=CARTESIAN_POINT('Ctrl Pts',(-9.04715504584287,-1.46256895709697,
-0.00127018677453484));
#58554=CARTESIAN_POINT('Origin',(-17.3,0.,0.));
#58555=CARTESIAN_POINT('',(-8.47584495415715,-1.46580452990507,-0.000374448332874922));
#58556=CARTESIAN_POINT('',(-8.54715504584287,-1.46590976831451,-0.000110809370955516));
#58557=CARTESIAN_POINT('',(-17.3,-1.4635,-1.79227059055215E-16));
#58558=CARTESIAN_POINT('Ctrl Pts',(-8.47584495415715,-1.46580452990507,
-0.000374448332874922));
#58559=CARTESIAN_POINT('Ctrl Pts',(-8.50125692203519,-1.46421447777039,
0.464922610210453));
#58560=CARTESIAN_POINT('Ctrl Pts',(-8.52666888991322,-1.22367892553067,
0.931633766965713));
#58561=CARTESIAN_POINT('Ctrl Pts',(-8.55208085779126,-0.843124218313088,
1.19919281640258));
#58562=CARTESIAN_POINT('Ctrl Pts',(-8.57859540019694,-0.446058002480036,
1.47836071856452));
#58563=CARTESIAN_POINT('Ctrl Pts',(-8.60510994260263,0.103441259930457,
1.5407199815395));
#58564=CARTESIAN_POINT('Ctrl Pts',(-8.63162448500832,0.552966651862248,
1.35762650988623));
#58565=CARTESIAN_POINT('Ctrl Pts',(-8.65813902741401,1.00249204379404,1.17453303823295));
#58566=CARTESIAN_POINT('Ctrl Pts',(-8.68465356981969,1.35204356524713,0.745986831951424));
#58567=CARTESIAN_POINT('Ctrl Pts',(-8.71116811222538,1.44105826751941,0.268836247614723));
#58568=CARTESIAN_POINT('Ctrl Pts',(-8.73768265463107,1.5300729697917,-0.208314336722033));
#58569=CARTESIAN_POINT('Ctrl Pts',(-8.76419719703676,1.35855085288313,-0.73406929911397));
#58570=CARTESIAN_POINT('Ctrl Pts',(-8.79071173944245,1.00527886283239,-1.06692842607179));
#58571=CARTESIAN_POINT('Ctrl Pts',(-8.81722628184813,0.65200687278171,-1.39978755302956));
#58572=CARTESIAN_POINT('Ctrl Pts',(-8.84374082425381,0.116985009588939,
-1.53975084455328));
#58573=CARTESIAN_POINT('Ctrl Pts',(-8.8702553666595,-0.354029856293153,
-1.42252758119857));
#58574=CARTESIAN_POINT('Ctrl Pts',(-8.89676990906518,-0.825044722175272,
-1.30530431784386));
#58575=CARTESIAN_POINT('Ctrl Pts',(-8.92328445147087,-1.2320525907467,-0.930894499610681));
#58576=CARTESIAN_POINT('Ctrl Pts',(-8.94979899387656,-1.38809852257213,
-0.471279481890183));
#58577=CARTESIAN_POINT('Ctrl Pts',(-8.95848098063676,-1.43919458500314,
-0.320782013837325));
#58578=CARTESIAN_POINT('Ctrl Pts',(-8.96716296739695,-1.46338287023551,
-0.161148967083977));
#58579=CARTESIAN_POINT('Ctrl Pts',(-8.97584495415714,-1.46219403757879,
-0.00116636394747058));
#58580=CARTESIAN_POINT('Ctrl Pts',(-9.04715504584287,-1.46256895709697,
-0.00127018677453484));
#58581=CARTESIAN_POINT('Ctrl Pts',(-9.03925404259752,-1.46376838799371,
-0.146767456688621));
#58582=CARTESIAN_POINT('Ctrl Pts',(-9.03135303935216,-1.44381825974912,
-0.291943146445416));
#58583=CARTESIAN_POINT('Ctrl Pts',(-9.02345203610681,-1.40137050280996,
-0.430212201342784));
#58584=CARTESIAN_POINT('Ctrl Pts',(-8.99693749370113,-1.25892240901231,
-0.894221720846118));
#58585=CARTESIAN_POINT('Ctrl Pts',(-8.97042295129543,-0.863112864449447,
-1.2804508195039));
#58586=CARTESIAN_POINT('Ctrl Pts',(-8.94390840888975,-0.395752971917505,
-1.41148907524943));
#58587=CARTESIAN_POINT('Ctrl Pts',(-8.91739386648406,0.0716069206144383,
-1.54252733099497));
#58588=CARTESIAN_POINT('Ctrl Pts',(-8.89087932407838,0.610517161115462,
-1.41837474382825));
#58589=CARTESIAN_POINT('Ctrl Pts',(-8.86436478167269,0.973434792424628,
-1.09605954638754));
#58590=CARTESIAN_POINT('Ctrl Pts',(-8.837850239267,1.33635242373379,-0.773744348946829));
#58591=CARTESIAN_POINT('Ctrl Pts',(-8.81133569686132,1.5232774458511,-0.253266541232123));
#58592=CARTESIAN_POINT('Ctrl Pts',(-8.78482115445563,1.44834774433747,0.226297670784763));
#58593=CARTESIAN_POINT('Ctrl Pts',(-8.75830661204994,1.37341804282383,0.705861882801677));
#58594=CARTESIAN_POINT('Ctrl Pts',(-8.73179206964426,1.03663361767922,1.14451249912077));
#58595=CARTESIAN_POINT('Ctrl Pts',(-8.70527752723857,0.592692981309976,
1.34075980482558));
#58596=CARTESIAN_POINT('Ctrl Pts',(-8.67876298483288,0.148752344940759,
1.53700711053039));
#58597=CARTESIAN_POINT('Ctrl Pts',(-8.6522484424272,-0.402344502653075,
1.49085110562094));
#58598=CARTESIAN_POINT('Ctrl Pts',(-8.62573390002151,-0.807456809852813,
1.2234930831649));
#58599=CARTESIAN_POINT('Ctrl Pts',(-8.59954094862863,-1.20765556903883,
0.95937780711978));
#58600=CARTESIAN_POINT('Ctrl Pts',(-8.57334799723575,-1.46538956251999,
0.479393826634133));
#58601=CARTESIAN_POINT('Ctrl Pts',(-8.54715504584287,-1.46590976831451,
-0.000110809370955516));
#58602=CARTESIAN_POINT('Origin',(-17.3,0.,0.));
#58603=CARTESIAN_POINT('',(-7.97584495415714,-1.46332934625901,0.0013523262496782));
#58604=CARTESIAN_POINT('',(-8.04715504584285,-1.46290284295625,0.00132519226194577));
#58605=CARTESIAN_POINT('',(-17.3,-1.4635,-1.79227059055215E-16));
#58606=CARTESIAN_POINT('Ctrl Pts',(-7.97584495415714,-1.46332934625901,
0.0013523262496782));
#58607=CARTESIAN_POINT('Ctrl Pts',(-7.98232179186204,-1.4644202230544,0.120466211293856));
#58608=CARTESIAN_POINT('Ctrl Pts',(-7.98879862956694,-1.45110187555386,
0.239339281952935));
#58609=CARTESIAN_POINT('Ctrl Pts',(-7.99527546727184,-1.42243811080014,
0.354389163718262));
#58610=CARTESIAN_POINT('Ctrl Pts',(-8.02179000967753,-1.30509587671973,
0.825374404946185));
#58611=CARTESIAN_POINT('Ctrl Pts',(-8.04830455208321,-0.930583263604335,
1.23228768770552));
#58612=CARTESIAN_POINT('Ctrl Pts',(-8.0748190944889,-0.470928844632437,
1.3882175195951));
#58613=CARTESIAN_POINT('Ctrl Pts',(-8.10133363689458,-0.0112744256605388,
1.54414735148468));
#58614=CARTESIAN_POINT('Ctrl Pts',(-8.12784817930028,0.533521799167859,
1.44909373250449));
#58615=CARTESIAN_POINT('Ctrl Pts',(-8.15436272170597,0.913213205445003,
1.1467185791721));
#58616=CARTESIAN_POINT('Ctrl Pts',(-8.18087726411166,1.29290461172213,0.844343425839718));
#58617=CARTESIAN_POINT('Ctrl Pts',(-8.20739180651734,1.50749119944801,0.334646738155148));
#58618=CARTESIAN_POINT('Ctrl Pts',(-8.23390634892302,1.45840479436909,-0.148247476129831));
#58619=CARTESIAN_POINT('Ctrl Pts',(-8.26042089132871,1.40931838929016,-0.63114169041481));
#58620=CARTESIAN_POINT('Ctrl Pts',(-8.2869354337344,1.09655899140643,-1.0872334313002));
#58621=CARTESIAN_POINT('Ctrl Pts',(-8.31344997614009,0.663789460343703,
-1.30702158006447));
#58622=CARTESIAN_POINT('Ctrl Pts',(-8.33996451854577,0.231019929280951,
-1.52680972882876));
#58623=CARTESIAN_POINT('Ctrl Pts',(-8.36647906095145,-0.321759734960807,
-1.5102942854719));
#58624=CARTESIAN_POINT('Ctrl Pts',(-8.39299360335714,-0.740635795990823,
-1.26506145151714));
#58625=CARTESIAN_POINT('Ctrl Pts',(-8.41950814576283,-1.15951185702082,
-1.01982861756239));
#58626=CARTESIAN_POINT('Ctrl Pts',(-8.44602268816852,-1.44448431483909,
-0.545878393009778));
#58627=CARTESIAN_POINT('Ctrl Pts',(-8.47253723057421,-1.46465395912042,
-0.0609150100590203));
#58628=CARTESIAN_POINT('Ctrl Pts',(-8.47363980510186,-1.46549268888901,
-0.0407484062119078));
#58629=CARTESIAN_POINT('Ctrl Pts',(-8.4747423796295,-1.46587351909118,-0.0205627583056027));
#58630=CARTESIAN_POINT('Ctrl Pts',(-8.47584495415715,-1.46580452990507,
-0.000374448332874922));
#58631=CARTESIAN_POINT('Ctrl Pts',(-8.54715504584287,-1.46590976831451,
-0.000110809370955516));
#58632=CARTESIAN_POINT('Ctrl Pts',(-8.54683345483006,-1.46591615528121,
-0.00599805663929943));
#58633=CARTESIAN_POINT('Ctrl Pts',(-8.54651186381725,-1.46588376891111,
-0.0118852316495221));
#58634=CARTESIAN_POINT('Ctrl Pts',(-8.54619027280445,-1.46581239682725,
-0.0177719339856615));
#58635=CARTESIAN_POINT('Ctrl Pts',(-8.51967573039876,-1.45992790979631,
-0.503118888677552));
#58636=CARTESIAN_POINT('Ctrl Pts',(-8.49316118799308,-1.18903116892879,
-0.98525275805866));
#58637=CARTESIAN_POINT('Ctrl Pts',(-8.46664664558739,-0.777555846624848,
-1.24271023561792));
#58638=CARTESIAN_POINT('Ctrl Pts',(-8.44013210318171,-0.366080524320909,
-1.50016771317719));
#58639=CARTESIAN_POINT('Ctrl Pts',(-8.41361756077602,0.185973379419495,
-1.53294879891458));
#58640=CARTESIAN_POINT('Ctrl Pts',(-8.38710301837033,0.625025498936305,
-1.32599583333036));
#58641=CARTESIAN_POINT('Ctrl Pts',(-8.36058847596464,1.06407761845314,-1.11904286774613));
#58642=CARTESIAN_POINT('Ctrl Pts',(-8.33407393355895,1.39012795374642,-0.672355850840293));
#58643=CARTESIAN_POINT('Ctrl Pts',(-8.30755939115327,1.45340858779386,-0.191115936690511));
#58644=CARTESIAN_POINT('Ctrl Pts',(-8.28104484874758,1.5166892218413,0.290123977459216));
#58645=CARTESIAN_POINT('Ctrl Pts',(-8.2545303063419,1.31720015464296,0.805916788852843));
#58646=CARTESIAN_POINT('Ctrl Pts',(-8.22801576393622,0.946574667410269,
1.11933829709663));
#58647=CARTESIAN_POINT('Ctrl Pts',(-8.20150122153053,0.575949180177555,
1.43275980534043));
#58648=CARTESIAN_POINT('Ctrl Pts',(-8.17498667912484,0.034187272910406,
1.54381001043435));
#58649=CARTESIAN_POINT('Ctrl Pts',(-8.14847213671915,-0.429858213002534,
1.40147912615362));
#58650=CARTESIAN_POINT('Ctrl Pts',(-8.12195759431346,-0.893903698915473,
1.25914824187289));
#58651=CARTESIAN_POINT('Ctrl Pts',(-8.09544305190777,-1.28023276347424,
0.863436268217562));
#58652=CARTESIAN_POINT('Ctrl Pts',(-8.06892850950209,-1.41138906628869,
0.396109489776231));
#58653=CARTESIAN_POINT('Ctrl Pts',(-8.06167068828234,-1.44729045893222,
0.2681882095508));
#58654=CARTESIAN_POINT('Ctrl Pts',(-8.0544128670626,-1.46407226164141,0.134900973761092));
#58655=CARTESIAN_POINT('Ctrl Pts',(-8.04715504584285,-1.46290284295625,
0.00132519226194577));
#58656=CARTESIAN_POINT('Origin',(-17.3,0.,0.));
#58657=CARTESIAN_POINT('',(-7.47584495415714,-1.46111246214465,-0.000242921189035072));
#58658=CARTESIAN_POINT('',(-7.54715504584287,-1.46121757502423,-0.000473021952020669));
#58659=CARTESIAN_POINT('',(-17.3,-1.4635,-1.79227059055215E-16));
#58660=CARTESIAN_POINT('Ctrl Pts',(-7.47584495415714,-1.46111246214465,
-0.000242921189035072));
#58661=CARTESIAN_POINT('Ctrl Pts',(-7.48990120409459,-1.46072923544993,
0.259251732184533));
#58662=CARTESIAN_POINT('Ctrl Pts',(-7.50395745403204,-1.39493658532748,
0.518927885930192));
#58663=CARTESIAN_POINT('Ctrl Pts',(-7.51801370396949,-1.26487433267444,
0.740955316438846));
#58664=CARTESIAN_POINT('Ctrl Pts',(-7.54452824637518,-1.01953570190919,
1.1597694203175));
#58665=CARTESIAN_POINT('Ctrl Pts',(-7.57104278878086,-0.545513510786813,
1.44462215313213));
#58666=CARTESIAN_POINT('Ctrl Pts',(-7.59755733118654,-0.0605450486214669,
1.46466929902454));
#58667=CARTESIAN_POINT('Ctrl Pts',(-7.62407187359223,0.424423413543935,
1.48471644491695));
#58668=CARTESIAN_POINT('Ctrl Pts',(-7.65058641599792,0.920338146752306,
1.23995800388708));
#58669=CARTESIAN_POINT('Ctrl Pts',(-7.67710095840361,1.19940574436146,0.842821285214332));
#58670=CARTESIAN_POINT('Ctrl Pts',(-7.70361550080929,1.4784733419706,0.445684566541602));
#58671=CARTESIAN_POINT('Ctrl Pts',(-7.73013004321498,1.54069380398054,-0.103830429773995));
#58672=CARTESIAN_POINT('Ctrl Pts',(-7.75664458562067,1.35748679176655,-0.553309559466464));
#58673=CARTESIAN_POINT('Ctrl Pts',(-7.78315912802635,1.17427977955254,-1.00278868915896));
#58674=CARTESIAN_POINT('Ctrl Pts',(-7.80967367043204,0.745645293114572,
-1.35223195222832));
#58675=CARTESIAN_POINT('Ctrl Pts',(-7.83618821283773,0.268472239620885,
-1.44112612736379));
#58676=CARTESIAN_POINT('Ctrl Pts',(-7.86270275524341,-0.208700813872774,
-1.53002030249926));
#58677=CARTESIAN_POINT('Ctrl Pts',(-7.8892172976491,-0.734412434422143,
-1.35836538970088));
#58678=CARTESIAN_POINT('Ctrl Pts',(-7.91573184005478,-1.06718231717409,
-1.00500933345345));
#58679=CARTESIAN_POINT('Ctrl Pts',(-7.93576954475557,-1.31866486369047,
-0.737969299309713));
#58680=CARTESIAN_POINT('Ctrl Pts',(-7.95580724945636,-1.45995444818576,
-0.367156035859364));
#58681=CARTESIAN_POINT('Ctrl Pts',(-7.97584495415714,-1.46332934625901,
0.0013523262496782));
#58682=CARTESIAN_POINT('Ctrl Pts',(-8.04715504584285,-1.46290284295625,
0.00132519226194577));
#58683=CARTESIAN_POINT('Ctrl Pts',(-8.02789832465691,-1.45980009780892,
-0.353083039030015));
#58684=CARTESIAN_POINT('Ctrl Pts',(-8.00864160347097,-1.33032672117917,
-0.709522536201345));
#58685=CARTESIAN_POINT('Ctrl Pts',(-7.98938488228503,-1.09630539301137,
-0.973157905781084));
#58686=CARTESIAN_POINT('Ctrl Pts',(-7.96287033987935,-0.774081875849499,
-1.33615693966975));
#58687=CARTESIAN_POINT('Ctrl Pts',(-7.93635579747366,-0.253651300455625,
-1.52321342421982));
#58688=CARTESIAN_POINT('Ctrl Pts',(-7.90984125506798,0.225931822886316,
-1.4484048590561));
#58689=CARTESIAN_POINT('Ctrl Pts',(-7.88332671266229,0.705514946228339,
-1.37359629389236));
#58690=CARTESIAN_POINT('Ctrl Pts',(-7.8568121702566,1.14425061751844,-1.03692267901471));
#58691=CARTESIAN_POINT('Ctrl Pts',(-7.83029762785091,1.34061005270123,-0.593031627256463));
#58692=CARTESIAN_POINT('Ctrl Pts',(-7.80378308544522,1.53696948788399,-0.149140575498266));
#58693=CARTESIAN_POINT('Ctrl Pts',(-7.77726854303954,1.49095268695951,0.401967913140544));
#58694=CARTESIAN_POINT('Ctrl Pts',(-7.75075400063385,1.22369700105575,0.80714773984519));
#58695=CARTESIAN_POINT('Ctrl Pts',(-7.72423945822817,0.956441315151998,
1.21232756654984));
#58696=CARTESIAN_POINT('Ctrl Pts',(-7.69772491582249,0.467946744269036,
1.47157873132032));
#58697=CARTESIAN_POINT('Ctrl Pts',(-7.6712103734168,-0.0174016813124656,
1.4658168391097));
#58698=CARTESIAN_POINT('Ctrl Pts',(-7.64469583101111,-0.502750106893995,
1.46005494689907));
#58699=CARTESIAN_POINT('Ctrl Pts',(-7.61818128860542,-0.984952387174048,
1.18927999770723));
#58700=CARTESIAN_POINT('Ctrl Pts',(-7.59166674619973,-1.24251379178837,
0.777869720162521));
#58701=CARTESIAN_POINT('Ctrl Pts',(-7.57682951274744,-1.38664219612179,
0.547649253250261));
#58702=CARTESIAN_POINT('Ctrl Pts',(-7.56199227929516,-1.46042671212876,
0.273390336954752));
#58703=CARTESIAN_POINT('Ctrl Pts',(-7.54715504584287,-1.46121757502423,
-0.000473021952020669));
#58704=CARTESIAN_POINT('Origin',(-17.3,0.,0.));
#58705=CARTESIAN_POINT('',(-6.97584495415715,-1.46422371240563,-0.00126593926974311));
#58706=CARTESIAN_POINT('',(-7.04715504584287,-1.46464284830267,-0.00115453508994419));
#58707=CARTESIAN_POINT('',(-17.3,-1.4635,-1.79227059055215E-16));
#58708=CARTESIAN_POINT('Ctrl Pts',(-6.97584495415715,-1.46422371240563,
-0.00126593926974311));
#58709=CARTESIAN_POINT('Ctrl Pts',(-6.99748061632714,-1.4605964766255,0.396006961252073));
#58710=CARTESIAN_POINT('Ctrl Pts',(-7.01911627849713,-1.29314413636782,
0.795971321500709));
#58711=CARTESIAN_POINT('Ctrl Pts',(-7.04075194066713,-1.00473973995226,
1.06743614018744));
#58712=CARTESIAN_POINT('Ctrl Pts',(-7.06726648307281,-0.651299640053113,
1.40011675750195));
#58713=CARTESIAN_POINT('Ctrl Pts',(-7.0937810254785,-0.116207137990993,
1.53980974696585));
#58714=CARTESIAN_POINT('Ctrl Pts',(-7.12029556788419,0.354748448532587,
1.42234854964644));
#58715=CARTESIAN_POINT('Ctrl Pts',(-7.14681011028988,0.825704035056194,
1.30488735232702));
#58716=CARTESIAN_POINT('Ctrl Pts',(-7.17332465269557,1.23252270604125,0.930271968224272));
#58717=CARTESIAN_POINT('Ctrl Pts',(-7.19983919510125,1.38833642804622,0.470578177328132));
#58718=CARTESIAN_POINT('Ctrl Pts',(-7.22635373750694,1.54415015005118,0.0108843864320189));
#58719=CARTESIAN_POINT('Ctrl Pts',(-7.25286827991262,1.44895892307608,-0.533887811257471));
#58720=CARTESIAN_POINT('Ctrl Pts',(-7.2793828223183,1.14648787247628,-0.913502827955351));
#58721=CARTESIAN_POINT('Ctrl Pts',(-7.30589736472399,0.844016821876477,
-1.29311784465323));
#58722=CARTESIAN_POINT('Ctrl Pts',(-7.33241190712968,0.334265947651977,
-1.5075756803595));
#58723=CARTESIAN_POINT('Ctrl Pts',(-7.35892644953537,-0.148615852407503,
-1.45836730175591));
#58724=CARTESIAN_POINT('Ctrl Pts',(-7.38544099194106,-0.631497652466983,
-1.40915892315231));
#58725=CARTESIAN_POINT('Ctrl Pts',(-7.41195553434673,-1.08751037836144,
-1.09628433023885));
#58726=CARTESIAN_POINT('Ctrl Pts',(-7.43847007675242,-1.30718920610463,
-0.66345929631075));
#58727=CARTESIAN_POINT('Ctrl Pts',(-7.45092836922066,-1.41040890506189,
-0.460089357740911));
#58728=CARTESIAN_POINT('Ctrl Pts',(-7.4633866616889,-1.46145212245702,-0.230237428974453));
#58729=CARTESIAN_POINT('Ctrl Pts',(-7.47584495415714,-1.46111246214465,
-0.000242921189035072));
#58730=CARTESIAN_POINT('Ctrl Pts',(-7.54715504584287,-1.46121757502423,
-0.000473021952020669));
#58731=CARTESIAN_POINT('Ctrl Pts',(-7.53547773688947,-1.46184000577589,
-0.216010983476512));
#58732=CARTESIAN_POINT('Ctrl Pts',(-7.52380042793608,-1.41724928492728,
-0.431303931970136));
#58733=CARTESIAN_POINT('Ctrl Pts',(-7.51212311898268,-1.32615366730869,
-0.624690543400295));
#58734=CARTESIAN_POINT('Ctrl Pts',(-7.48560857657699,-1.11931160926606,
-1.06379492352077));
#58735=CARTESIAN_POINT('Ctrl Pts',(-7.4590940341713,-0.672706964232189,
-1.38995807786417));
#58736=CARTESIAN_POINT('Ctrl Pts',(-7.43257949176561,-0.191483049600187,
-1.45336026712094));
#58737=CARTESIAN_POINT('Ctrl Pts',(-7.40606494935992,0.289740865031816,
-1.51676245637771));
#58738=CARTESIAN_POINT('Ctrl Pts',(-7.37955040695424,0.80558404926195,-1.31740368054786));
#58739=CARTESIAN_POINT('Ctrl Pts',(-7.35303586454856,1.1190991644445,-0.946857372823209));
#58740=CARTESIAN_POINT('Ctrl Pts',(-7.32652132214287,1.43261427962704,-0.576311065098553));
#58741=CARTESIAN_POINT('Ctrl Pts',(-7.30000677973718,1.543801325762,-0.0345772254790913));
#58742=CARTESIAN_POINT('Ctrl Pts',(-7.27349223733149,1.40158766007931,0.429504197236137));
#58743=CARTESIAN_POINT('Ctrl Pts',(-7.24697769492581,1.2593739943966,0.893585619951392));
#58744=CARTESIAN_POINT('Ctrl Pts',(-7.22046315252012,0.863759616896217,
1.2800146257624));
#58745=CARTESIAN_POINT('Ctrl Pts',(-7.19394861011444,0.396465982362147,
1.41128896727767));
#58746=CARTESIAN_POINT('Ctrl Pts',(-7.16743406770875,-0.0708276521718959,
1.54256330879292));
#58747=CARTESIAN_POINT('Ctrl Pts',(-7.14091952530306,-0.609800543739616,
1.41868298601245));
#58748=CARTESIAN_POINT('Ctrl Pts',(-7.11440498289737,-0.972880957047548,
1.09655116968807));
#58749=CARTESIAN_POINT('Ctrl Pts',(-7.09198833721254,-1.27984627652,0.824205726954458));
#58750=CARTESIAN_POINT('Ctrl Pts',(-7.0695716915277,-1.46108699957425,0.410153889145206));
#58751=CARTESIAN_POINT('Ctrl Pts',(-7.04715504584287,-1.46464284830267,
-0.00115453508994419));
#58752=CARTESIAN_POINT('Origin',(-17.3,0.,0.));
#58753=CARTESIAN_POINT('',(-6.47584495415715,-1.46530145832529,0.000851233357479376));
#58754=CARTESIAN_POINT('',(-6.54715504584287,-1.4649516336717,0.00103626765265278));
#58755=CARTESIAN_POINT('',(-17.3,-1.4635,-1.79227059055215E-16));
#58756=CARTESIAN_POINT('Ctrl Pts',(-6.47584495415715,-1.46530145832529,
0.000851233357479376));
#58757=CARTESIAN_POINT('Ctrl Pts',(-6.478545486154,-1.46564330146594,0.0503433694787354));
#58758=CARTESIAN_POINT('Ctrl Pts',(-6.48124601815086,-1.46335406023885,
0.0998035045751598));
#58759=CARTESIAN_POINT('Ctrl Pts',(-6.48394655014771,-1.45832971609511,
0.1489842192031));
#58760=CARTESIAN_POINT('Ctrl Pts',(-6.5104610925534,-1.40899936710646,0.631853574228028));
#58761=CARTESIAN_POINT('Ctrl Pts',(-6.53697563495909,-1.09600959912541,
1.08778725603681));
#58762=CARTESIAN_POINT('Ctrl Pts',(-6.56349017736478,-0.663129089947229,
1.30735674874281));
#58763=CARTESIAN_POINT('Ctrl Pts',(-6.59000471977046,-0.230248580769118,
1.52692624144877));
#58764=CARTESIAN_POINT('Ctrl Pts',(-6.61651926217615,0.322522669606081,
1.51013154505203));
#58765=CARTESIAN_POINT('Ctrl Pts',(-6.64303380458183,0.741274789612,1.26468713312949));
#58766=CARTESIAN_POINT('Ctrl Pts',(-6.66954834698752,1.16002690961794,1.01924272120694));
#58767=CARTESIAN_POINT('Ctrl Pts',(-6.6960628893932,1.44475989925459,0.545148593758567));
#58768=CARTESIAN_POINT('Ctrl Pts',(-6.72257743179889,1.46468454547897,0.0601750833208196));
#58769=CARTESIAN_POINT('Ctrl Pts',(-6.74909197420457,1.48460919170335,-0.424798427116929));
#58770=CARTESIAN_POINT('Ctrl Pts',(-6.77560651661026,1.23972549451545,-0.920651320544051));
#58771=CARTESIAN_POINT('Ctrl Pts',(-6.80212105901595,0.842518298341396,
-1.19961859579515));
#58772=CARTESIAN_POINT('Ctrl Pts',(-6.82863560142163,0.445311102167339,
-1.47858587104625));
#58773=CARTESIAN_POINT('Ctrl Pts',(-6.85515014382732,-0.10421959299288,
-1.54066752812133));
#58774=CARTESIAN_POINT('Ctrl Pts',(-6.88166468623301,-0.553652431768097,
-1.3573469870357));
#58775=CARTESIAN_POINT('Ctrl Pts',(-6.90817922863869,-1.00308527054334,
-1.17402644595006));
#58776=CARTESIAN_POINT('Ctrl Pts',(-6.93469377104438,-1.35242025293356,
-0.745303706703668));
#58777=CARTESIAN_POINT('Ctrl Pts',(-6.96120831345007,-1.44119389526058,
-0.268108214497904));
#58778=CARTESIAN_POINT('Ctrl Pts',(-6.96608719368576,-1.45752892991337,
-0.18030056464817));
#58779=CARTESIAN_POINT('Ctrl Pts',(-6.97096607392146,-1.46504166051458,
-0.0908516837366048));
#58780=CARTESIAN_POINT('Ctrl Pts',(-6.97584495415715,-1.46422371240563,
-0.00126593926974311));
#58781=CARTESIAN_POINT('Ctrl Pts',(-7.04715504584287,-1.46464284830267,
-0.00115453508994419));
#58782=CARTESIAN_POINT('Ctrl Pts',(-7.04305714912202,-1.46529287868852,
-0.0763441716942909));
#58783=CARTESIAN_POINT('Ctrl Pts',(-7.03895925240117,-1.46000503173595,
-0.151442128838845));
#58784=CARTESIAN_POINT('Ctrl Pts',(-7.03486135568032,-1.44846188136273,
-0.225565960572915));
#58785=CARTESIAN_POINT('Ctrl Pts',(-7.00834681327463,-1.37377445732185,
-0.705167964641356));
#58786=CARTESIAN_POINT('Ctrl Pts',(-6.98183227086895,-1.03721167419188,
-1.14398866290993));
#58787=CARTESIAN_POINT('Ctrl Pts',(-6.95531772846326,-0.593370235366074,
-1.34046021504245));
#58788=CARTESIAN_POINT('Ctrl Pts',(-6.92880318605757,-0.149528796540265,
-1.53693176717497));
#58789=CARTESIAN_POINT('Ctrl Pts',(-6.90228864365188,0.401591297981385,
-1.49105417317145));
#58790=CARTESIAN_POINT('Ctrl Pts',(-6.8757741012462,0.806838618339453,-1.22390084087157));
#58791=CARTESIAN_POINT('Ctrl Pts',(-6.84925955884051,1.2120859386975,-0.956747508571697));
#58792=CARTESIAN_POINT('Ctrl Pts',(-6.82274501643483,1.47146048489198,-0.468318437975495));
#58793=CARTESIAN_POINT('Ctrl Pts',(-6.79623047402914,1.46582118786923,0.0170314275291633));
#58794=CARTESIAN_POINT('Ctrl Pts',(-6.76971593162346,1.46018189084648,0.502381293033822));
#58795=CARTESIAN_POINT('Ctrl Pts',(-6.74320138921777,1.18952875060651,0.984651953446936));
#58796=CARTESIAN_POINT('Ctrl Pts',(-6.71668684681208,0.778183544070094,
1.24231726868323));
#58797=CARTESIAN_POINT('Ctrl Pts',(-6.69017230440639,0.366838337533681,
1.49998258391951));
#58798=CARTESIAN_POINT('Ctrl Pts',(-6.6636577620007,-0.185198935299168,
1.53304255397898));
#58799=CARTESIAN_POINT('Ctrl Pts',(-6.63714321959502,-0.624355548007335,
1.32631141667502));
#58800=CARTESIAN_POINT('Ctrl Pts',(-6.61062867718933,-1.06351216071555,
1.11958027937104));
#58801=CARTESIAN_POINT('Ctrl Pts',(-6.58411413478364,-1.38978811329906,
0.673058034703574));
#58802=CARTESIAN_POINT('Ctrl Pts',(-6.55759959237795,-1.45331185371989,
0.191850150292584));
#58803=CARTESIAN_POINT('Ctrl Pts',(-6.55411807686626,-1.46165289480791,
0.128664722149329));
#58804=CARTESIAN_POINT('Ctrl Pts',(-6.55063656135457,-1.46546376299974,
0.0648812707058691));
#58805=CARTESIAN_POINT('Ctrl Pts',(-6.54715504584287,-1.4649516336717,0.00103626765265278));
#58806=CARTESIAN_POINT('Origin',(-17.3,0.,0.));
#58807=CARTESIAN_POINT('',(-5.97584495415714,-1.46156852434996,0.000844616552042321));
#58808=CARTESIAN_POINT('',(-6.04715504584287,-1.46134752925932,0.000644857312986237));
#58809=CARTESIAN_POINT('',(-17.3,-1.4635,-1.79227059055215E-16));
#58810=CARTESIAN_POINT('Ctrl Pts',(-5.97584495415714,-1.46156852434996,
0.000844616552042321));
#58811=CARTESIAN_POINT('Ctrl Pts',(-5.98612489838655,-1.46256065115051,
0.190476374356358));
#58812=CARTESIAN_POINT('Ctrl Pts',(-5.99640484261595,-1.42832625212033,
0.37976377404471));
#58813=CARTESIAN_POINT('Ctrl Pts',(-6.00668478684535,-1.35720709570256,
0.553995268745348));
#58814=CARTESIAN_POINT('Ctrl Pts',(-6.03319932925104,-1.17377303744159,
1.00338178792832));
#58815=CARTESIAN_POINT('Ctrl Pts',(-6.05971387165673,-0.744962072740432,
1.35260846735091));
#58816=CARTESIAN_POINT('Ctrl Pts',(-6.08622841406242,-0.267744172268927,
1.44126157120546));
#58817=CARTESIAN_POINT('Ctrl Pts',(-6.1127429564681,0.20947372820258,1.52991467506002));
#58818=CARTESIAN_POINT('Ctrl Pts',(-6.13925749887378,0.735098564444436,
1.35799420334655));
#58819=CARTESIAN_POINT('Ctrl Pts',(-6.16577204127946,1.06768989509561,1.00447008234607));
#58820=CARTESIAN_POINT('Ctrl Pts',(-6.19228658368516,1.40028122574683,0.650945961345559));
#58821=CARTESIAN_POINT('Ctrl Pts',(-6.21880112609086,1.53983905080732,0.115818191058003));
#58822=CARTESIAN_POINT('Ctrl Pts',(-6.24531566849655,1.4222588977432,-0.355107710713123));
#58823=CARTESIAN_POINT('Ctrl Pts',(-6.27183021090223,1.3046787446791,-0.826033612484143));
#58824=CARTESIAN_POINT('Ctrl Pts',(-6.2983447533079,0.929960613490508,-1.23275764573877));
#58825=CARTESIAN_POINT('Ctrl Pts',(-6.32485929571358,0.470227479999877,
-1.38845524791783));
#58826=CARTESIAN_POINT('Ctrl Pts',(-6.35137383811927,0.0104943465091679,
-1.54415285009693));
#58827=CARTESIAN_POINT('Ctrl Pts',(-6.37788838052497,-0.534253789283616,
-1.44882402120037));
#58828=CARTESIAN_POINT('Ctrl Pts',(-6.40440292293066,-0.913792392181853,
-1.14625709263157));
#58829=CARTESIAN_POINT('Ctrl Pts',(-6.42821693333949,-1.25467461830821,
-0.874506900753448));
#58830=CARTESIAN_POINT('Ctrl Pts',(-6.45203094374832,-1.46228699446443,
-0.435583604711616));
#58831=CARTESIAN_POINT('Ctrl Pts',(-6.47584495415715,-1.46530145832529,
0.000851233357479376));
#58832=CARTESIAN_POINT('Ctrl Pts',(-6.54715504584287,-1.4649516336717,0.00103626765265278));
#58833=CARTESIAN_POINT('Ctrl Pts',(-6.52412201894888,-1.4615634860256,-0.42134980744384));
#58834=CARTESIAN_POINT('Ctrl Pts',(-6.50108899205489,-1.26896261059051,
-0.846429927107413));
#58835=CARTESIAN_POINT('Ctrl Pts',(-6.4780559651609,-0.947140017824197,
-1.11885996039094));
#58836=CARTESIAN_POINT('Ctrl Pts',(-6.45154142275521,-0.576672913249429,
-1.43246866250914));
#58837=CARTESIAN_POINT('Ctrl Pts',(-6.42502688034953,-0.0349671758416458,
-1.54379254259112));
#58838=CARTESIAN_POINT('Ctrl Pts',(-6.39851233794385,0.429150154066261,
-1.40169610458007));
#58839=CARTESIAN_POINT('Ctrl Pts',(-6.37199779553816,0.893267483974247,
-1.25959966656899));
#58840=CARTESIAN_POINT('Ctrl Pts',(-6.34548325313247,1.27979640638233,-0.864082910464783));
#58841=CARTESIAN_POINT('Ctrl Pts',(-6.31896871072678,1.41118877822275,-0.396822449652507));
#58842=CARTESIAN_POINT('Ctrl Pts',(-6.29245416832109,1.54258115006316,0.0704380111597157));
#58843=CARTESIAN_POINT('Ctrl Pts',(-6.2659396259154,1.418836971336,0.609442176679984));
#58844=CARTESIAN_POINT('Ctrl Pts',(-6.23942508350972,1.09679687640198,0.972603946241689));
#58845=CARTESIAN_POINT('Ctrl Pts',(-6.21291054110403,0.774756781467961,
1.33576571580339));
#58846=CARTESIAN_POINT('Ctrl Pts',(-6.18639599869835,0.254420770327094,
1.52308508940653));
#58847=CARTESIAN_POINT('Ctrl Pts',(-6.15988145629266,-0.225200083867905,
1.44851881125373));
#58848=CARTESIAN_POINT('Ctrl Pts',(-6.13336691388698,-0.704820938062904,
1.37395253310093));
#58849=CARTESIAN_POINT('Ctrl Pts',(-6.10685237148129,-1.14372663531203,
1.03750060319219));
#58850=CARTESIAN_POINT('Ctrl Pts',(-6.0803378290756,-1.34031029185887,0.593708805617051));
#58851=CARTESIAN_POINT('Ctrl Pts',(-6.06927690133136,-1.42231802887709,
0.408574590160477));
#58852=CARTESIAN_POINT('Ctrl Pts',(-6.05821597358711,-1.46215536248318,
0.204760416790964));
#58853=CARTESIAN_POINT('Ctrl Pts',(-6.04715504584287,-1.46134752925932,
0.000644857312986237));
#58854=CARTESIAN_POINT('Origin',(-17.3,0.,0.));
#58855=CARTESIAN_POINT('',(-5.47584495415715,-1.46220625068146,-0.00117056217213363));
#58856=CARTESIAN_POINT('',(-5.54715504584287,-1.46258246545509,-0.00127304540250365));
#58857=CARTESIAN_POINT('',(-17.3,-1.4635,-1.79227059055215E-16));
#58858=CARTESIAN_POINT('Ctrl Pts',(-5.47584495415715,-1.46220625068146,
-0.00117056217213363));
#58859=CARTESIAN_POINT('Ctrl Pts',(-5.4937043106191,-1.45975057338693,0.327916119857958));
#58860=CARTESIAN_POINT('Ctrl Pts',(-5.51156366708105,-1.34989031251731,
0.65848819549645));
#58861=CARTESIAN_POINT('Ctrl Pts',(-5.529423023543,-1.14602623965269,0.914081898106037));
#58862=CARTESIAN_POINT('Ctrl Pts',(-5.55593756594869,-0.843363452419451,
1.29354406298907));
#58863=CARTESIAN_POINT('Ctrl Pts',(-5.58245210835437,-0.333504302688776,
1.50774435361542));
#58864=CARTESIAN_POINT('Ctrl Pts',(-5.60896665076006,0.1493525764932,1.4582920373891));
#58865=CARTESIAN_POINT('Ctrl Pts',(-5.63548119316574,0.632209455675149,
1.40883972116278));
#58866=CARTESIAN_POINT('Ctrl Pts',(-5.66199573557143,1.0880640643084,1.09573479808381));
#58867=CARTESIAN_POINT('Ctrl Pts',(-5.68851027797711,1.30752420796813,0.662798841274575));
#58868=CARTESIAN_POINT('Ctrl Pts',(-5.7150248203828,1.52698435162785,0.229862884465363));
#58869=CARTESIAN_POINT('Ctrl Pts',(-5.74153936278849,1.51005003031407,-0.322904106074104));
#58870=CARTESIAN_POINT('Ctrl Pts',(-5.76805390519417,1.26449985289427,-0.741594215489832));
#58871=CARTESIAN_POINT('Ctrl Pts',(-5.79456844759986,1.01894967547444,-1.16028432490561));
#58872=CARTESIAN_POINT('Ctrl Pts',(-5.82108299000554,0.54478364194851,-1.44489755319761));
#58873=CARTESIAN_POINT('Ctrl Pts',(-5.84759753241123,0.0598051141809271,
-1.46469969848274));
#58874=CARTESIAN_POINT('Ctrl Pts',(-5.87411207481692,-0.425173413586656,
-1.48450184376786));
#58875=CARTESIAN_POINT('Ctrl Pts',(-5.90062661722261,-0.920964435595895,
-1.23949290604612));
#58876=CARTESIAN_POINT('Ctrl Pts',(-5.9271411596283,-1.19983137069012,-0.842215257713543));
#58877=CARTESIAN_POINT('Ctrl Pts',(-5.94337575780458,-1.37057890110706,
-0.598965991465038));
#58878=CARTESIAN_POINT('Ctrl Pts',(-5.95961035598086,-1.46000170846191,
-0.298631267821943));
#58879=CARTESIAN_POINT('Ctrl Pts',(-5.97584495415714,-1.46156852434996,
0.000844616552042321));
#58880=CARTESIAN_POINT('Ctrl Pts',(-6.04715504584287,-1.46134752925932,
0.000644857312986237));
#58881=CARTESIAN_POINT('Ctrl Pts',(-6.03170143118143,-1.46021887679535,
-0.284532234113107));
#58882=CARTESIAN_POINT('Ctrl Pts',(-6.01624781651998,-1.37975136403226,
-0.570297627475704));
#58883=CARTESIAN_POINT('Ctrl Pts',(-6.00079420185854,-1.22410460259934,
-0.806529445355322));
#58884=CARTESIAN_POINT('Ctrl Pts',(-5.97427965945285,-0.95705364094843,
-1.21184423351093));
#58885=CARTESIAN_POINT('Ctrl Pts',(-5.94776511704716,-0.468690101802097,
-1.47134214458061));
#58886=CARTESIAN_POINT('Ctrl Pts',(-5.92125057464148,0.0166611726591288,
-1.46582544310558));
#58887=CARTESIAN_POINT('Ctrl Pts',(-5.89473603223579,0.502012447120327,
-1.46030874163054));
#58888=CARTESIAN_POINT('Ctrl Pts',(-5.86822148983011,0.984351456896417,
-1.18977742761082));
#58889=CARTESIAN_POINT('Ctrl Pts',(-5.84170694742443,1.24212066631498,-0.778497318327611));
#58890=CARTESIAN_POINT('Ctrl Pts',(-5.81519240501874,1.49988987573356,-0.36721720904436));
#58891=CARTESIAN_POINT('Ctrl Pts',(-5.78867786261305,1.53308928479456,0.184811695502411));
#58892=CARTESIAN_POINT('Ctrl Pts',(-5.76216332020736,1.32646908141922,0.624020512778951));
#58893=CARTESIAN_POINT('Ctrl Pts',(-5.73564877780167,1.11984887804388,1.06322933005547));
#58894=CARTESIAN_POINT('Ctrl Pts',(-5.70913423539599,0.673409062232237,
1.38961806006177));
#58895=CARTESIAN_POINT('Ctrl Pts',(-5.68261969299031,0.19221723874469,1.45326334759375));
#58896=CARTESIAN_POINT('Ctrl Pts',(-5.65610515058462,-0.288974584742884,
1.51690863512575));
#58897=CARTESIAN_POINT('Ctrl Pts',(-5.62959060817893,-0.804918415906365,
1.31781048018338));
#58898=CARTESIAN_POINT('Ctrl Pts',(-5.60307606577324,-1.11862068495122,
0.9474226023952));
#58899=CARTESIAN_POINT('Ctrl Pts',(-5.58443572579645,-1.33916067606315,
0.687031309963428));
#58900=CARTESIAN_POINT('Ctrl Pts',(-5.56579538581966,-1.45974445354556,
0.341981493586538));
#58901=CARTESIAN_POINT('Ctrl Pts',(-5.54715504584287,-1.46258246545509,
-0.00127304540250365));
#58902=CARTESIAN_POINT('Origin',(-17.3,0.,0.));
#58903=CARTESIAN_POINT('',(-4.97584495415715,-1.46580988090682,-0.00036561919089767));
#58904=CARTESIAN_POINT('',(-5.04715504584287,-1.46591140803628,-0.000101597247445848));
#58905=CARTESIAN_POINT('',(-17.3,-1.4635,-1.79227059055215E-16));
#58906=CARTESIAN_POINT('Ctrl Pts',(-4.97584495415715,-1.46580988090682,
-0.00036561919089767));
#58907=CARTESIAN_POINT('Ctrl Pts',(-5.00128372285165,-1.46425219013824,
0.465417621113056));
#58908=CARTESIAN_POINT('Ctrl Pts',(-5.02672249154614,-1.22313864729725,
0.932587879623785));
#58909=CARTESIAN_POINT('Ctrl Pts',(-5.05216126024064,-0.841912163350243,
1.20004406903268));
#58910=CARTESIAN_POINT('Ctrl Pts',(-5.07867580264632,-0.444564088206552,
1.47881064617758));
#58911=CARTESIAN_POINT('Ctrl Pts',(-5.10519034505201,0.10499789945747,1.54061468150885));
#58912=CARTESIAN_POINT('Ctrl Pts',(-5.1317048874577,0.554338070376188,1.35706711777613));
#58913=CARTESIAN_POINT('Ctrl Pts',(-5.15821942986338,1.00367824129491,1.17351955404341));
#58914=CARTESIAN_POINT('Ctrl Pts',(-5.18473397226907,1.35279659546832,0.744620391246714));
#58915=CARTESIAN_POINT('Ctrl Pts',(-5.21124851467476,1.44132915519413,0.267380112957177));
#58916=CARTESIAN_POINT('Ctrl Pts',(-5.23776305708044,1.52986171491994,-0.209860165332388));
#58917=CARTESIAN_POINT('Ctrl Pts',(-5.26427759948613,1.35780848019811,-0.735441559114797));
#58918=CARTESIAN_POINT('Ctrl Pts',(-5.29079214189182,1.00420036065203,-1.06794358188246));
#58919=CARTESIAN_POINT('Ctrl Pts',(-5.3173066842975,0.650592241105968,-1.40044560465011));
#58920=CARTESIAN_POINT('Ctrl Pts',(-5.34382122670319,0.115429236735669,
-1.53986825640303));
#58921=CARTESIAN_POINT('Ctrl Pts',(-5.37033576910888,-0.355466950236626,
-1.42216915509621));
#58922=CARTESIAN_POINT('Ctrl Pts',(-5.39685031151456,-0.826363137208922,
-1.3044700537894));
#58923=CARTESIAN_POINT('Ctrl Pts',(-5.42336485392025,-1.23299250678321,
-0.929649199422844));
#58924=CARTESIAN_POINT('Ctrl Pts',(-5.44987939632593,-1.38857397920246,
-0.469876752669737));
#58925=CARTESIAN_POINT('Ctrl Pts',(-5.45853458226967,-1.43936069664173,
-0.319792472218341));
#58926=CARTESIAN_POINT('Ctrl Pts',(-5.46718976821341,-1.46339634639668,
-0.160655951841513));
#58927=CARTESIAN_POINT('Ctrl Pts',(-5.47584495415715,-1.46220625068146,
-0.00117056217213363));
#58928=CARTESIAN_POINT('Ctrl Pts',(-5.54715504584287,-1.46258246545509,
-0.00127304540250365));
#58929=CARTESIAN_POINT('Ctrl Pts',(-5.53928084341397,-1.463781321286,-0.146273390246097));
#58930=CARTESIAN_POINT('Ctrl Pts',(-5.53140664098508,-1.44396898032646,
-0.290953375998168));
#58931=CARTESIAN_POINT('Ctrl Pts',(-5.52353243855618,-1.40180445964895,
-0.428796083515654));
#58932=CARTESIAN_POINT('Ctrl Pts',(-5.4970178961505,-1.25982525837558,-0.892949291004386));
#58933=CARTESIAN_POINT('Ctrl Pts',(-5.47050335374481,-0.864406148902612,
-1.27957810534789));
#58934=CARTESIAN_POINT('Ctrl Pts',(-5.44398881133913,-0.397178891624646,
-1.41108849913032));
#58935=CARTESIAN_POINT('Ctrl Pts',(-5.41747426893344,0.0700483656533723,
-1.54259889291276));
#58936=CARTESIAN_POINT('Ctrl Pts',(-5.39095972652775,0.609083770736402,
-1.41899086613407));
#58937=CARTESIAN_POINT('Ctrl Pts',(-5.36444518412206,0.972326873381239,
-1.09704251313735));
#58938=CARTESIAN_POINT('Ctrl Pts',(-5.33793064171637,1.33556997602601,-0.775094160140676));
#58939=CARTESIAN_POINT('Ctrl Pts',(-5.31141609931069,1.52302077623267,-0.254805480926044));
#58940=CARTESIAN_POINT('Ctrl Pts',(-5.284901556905,1.4485756487255,0.224834192794464));
#58941=CARTESIAN_POINT('Ctrl Pts',(-5.25838701449932,1.37413052121833,0.704473866514999));
#58942=CARTESIAN_POINT('Ctrl Pts',(-5.23187247209363,1.0377894659973,1.14346453474141));
#58943=CARTESIAN_POINT('Ctrl Pts',(-5.20535792968795,0.594047337987869,
1.34016028316003));
#58944=CARTESIAN_POINT('Ctrl Pts',(-5.17884338728226,0.150305209978438,
1.53685603157865));
#58945=CARTESIAN_POINT('Ctrl Pts',(-5.15232884487657,-0.4008379908194,1.49125686018949));
#58946=CARTESIAN_POINT('Ctrl Pts',(-5.12581430247089,-0.806220220912455,
1.22430828622611));
#58947=CARTESIAN_POINT('Ctrl Pts',(-5.09959455026155,-1.20709538822551,
0.960327661749831));
#58948=CARTESIAN_POINT('Ctrl Pts',(-5.07337479805221,-1.46543272473564,
0.479892224027581));
#58949=CARTESIAN_POINT('Ctrl Pts',(-5.04715504584287,-1.46591140803628,
-0.000101597247445848));
#58950=CARTESIAN_POINT('Origin',(-17.3,0.,0.));
#58951=CARTESIAN_POINT('',(-4.47584495415716,-1.46331444493144,0.00135213804196392));
#58952=CARTESIAN_POINT('',(-4.54715504584288,-1.46288856329395,0.00132347729660035));
#58953=CARTESIAN_POINT('',(-17.3,-1.4635,-1.79227059055215E-16));
#58954=CARTESIAN_POINT('Ctrl Pts',(-4.47584495415716,-1.46331444493144,
0.00135213804196392));
#58955=CARTESIAN_POINT('Ctrl Pts',(-4.48234859267851,-1.46440871301316,
0.120962016398508));
#58956=CARTESIAN_POINT('Ctrl Pts',(-4.48885223119987,-1.45097840452381,
0.24032935462986));
#58957=CARTESIAN_POINT('Ctrl Pts',(-4.49535586972122,-1.42207932171114,
0.355826167080497));
#58958=CARTESIAN_POINT('Ctrl Pts',(-4.52187041212691,-1.3042612796711,0.826692609209612));
#58959=CARTESIAN_POINT('Ctrl Pts',(-4.54838495453259,-0.929337726041169,
1.23322728915951));
#58960=CARTESIAN_POINT('Ctrl Pts',(-4.57489949693828,-0.469525995360321,
1.38869262189244));
#58961=CARTESIAN_POINT('Ctrl Pts',(-4.60141403934397,-0.00971426467944604,
1.54415795462538));
#58962=CARTESIAN_POINT('Ctrl Pts',(-4.62792858174965,0.534985643052358,
1.44855394014133));
#58963=CARTESIAN_POINT('Ctrl Pts',(-4.65444312415534,0.914371345709493,
1.14579531355431));
#58964=CARTESIAN_POINT('Ctrl Pts',(-4.68095766656103,1.29375704836661,0.84303668696731));
#58965=CARTESIAN_POINT('Ctrl Pts',(-4.70747220896671,1.50782854594907,0.33312344827737));
#58966=CARTESIAN_POINT('Ctrl Pts',(-4.7339867513724,1.45825426564029,-0.149720924254138));
#58967=CARTESIAN_POINT('Ctrl Pts',(-4.76050129377809,1.40867998533151,-0.632565296785646));
#58968=CARTESIAN_POINT('Ctrl Pts',(-4.78701583618377,1.09545992713148,-1.08834080315872));
#58969=CARTESIAN_POINT('Ctrl Pts',(-4.81353037858946,0.662468550313567,
-1.30769158377006));
#58970=CARTESIAN_POINT('Ctrl Pts',(-4.84004492099515,0.22947717349565,-1.5270423643814));
#58971=CARTESIAN_POINT('Ctrl Pts',(-4.86655946340083,-0.32328552194016,
-1.509968419231));
#58972=CARTESIAN_POINT('Ctrl Pts',(-4.89307400580652,-0.741913594052176,
-1.2643124919806));
#58973=CARTESIAN_POINT('Ctrl Pts',(-4.9195885482122,-1.16054166616422,-1.01865656473018));
#58974=CARTESIAN_POINT('Ctrl Pts',(-4.94610309061789,-1.44503511495245,
-0.544418655379736));
#58975=CARTESIAN_POINT('Ctrl Pts',(-4.97261763302358,-1.46471475803487,
-0.0594351412252308));
#58976=CARTESIAN_POINT('Ctrl Pts',(-4.97369340673477,-1.46551321958664,
-0.0397579200646598));
#58977=CARTESIAN_POINT('Ctrl Pts',(-4.97476918044596,-1.46587575370118,
-0.0200630098566805));
#58978=CARTESIAN_POINT('Ctrl Pts',(-4.97584495415715,-1.46580988090682,
-0.00036561919089767));
#58979=CARTESIAN_POINT('Ctrl Pts',(-5.04715504584287,-1.46591140803628,
-0.000101597247445848));
#58980=CARTESIAN_POINT('Ctrl Pts',(-5.04686025564653,-1.46591678990042,
-0.00549819564738455));
#58981=CARTESIAN_POINT('Ctrl Pts',(-5.04656546545018,-1.46588957679224,
-0.0108947382241984));
#58982=CARTESIAN_POINT('Ctrl Pts',(-5.04627067525383,-1.46582960481847,
-0.016290916725986));
#58983=CARTESIAN_POINT('Ctrl Pts',(-5.01975613284814,-1.46043549924315,
-0.501643569177134));
#58984=CARTESIAN_POINT('Ctrl Pts',(-4.99324159044245,-1.1900260287042,-0.984050897541824));
#58985=CARTESIAN_POINT('Ctrl Pts',(-4.96672704803676,-0.778811042914844,
-1.2419239846963));
#58986=CARTESIAN_POINT('Ctrl Pts',(-4.94021250563108,-0.367596057125508,
-1.49979707185076));
#58987=CARTESIAN_POINT('Ctrl Pts',(-4.91369796322539,0.184424443914241,
-1.53313591779505));
#58988=CARTESIAN_POINT('Ctrl Pts',(-4.88718342081971,0.623685437736442,
-1.32662666153125));
#58989=CARTESIAN_POINT('Ctrl Pts',(-4.86066887841402,1.06294643155864,-1.12011740526745));
#58990=CARTESIAN_POINT('Ctrl Pts',(-4.83415433600833,1.38944791816332,-0.673760046795552));
#58991=CARTESIAN_POINT('Ctrl Pts',(-4.80763979360265,1.45321474874567,-0.192584314932677));
#58992=CARTESIAN_POINT('Ctrl Pts',(-4.78112525119696,1.51698157932803,0.288591416930226));
#58993=CARTESIAN_POINT('Ctrl Pts',(-4.75461070879128,1.31801375388804,0.804585522184146));
#58994=CARTESIAN_POINT('Ctrl Pts',(-4.72809616638559,0.947705126518188,
1.11838133814061));
#58995=CARTESIAN_POINT('Ctrl Pts',(-4.7015816239799,0.57739649914834,1.43217715409708));
#58996=CARTESIAN_POINT('Ctrl Pts',(-4.67506708157421,0.0357470698487191,
1.5437746807561));
#58997=CARTESIAN_POINT('Ctrl Pts',(-4.64855253916852,-0.428441985606666,
1.40191272527909));
#58998=CARTESIAN_POINT('Ctrl Pts',(-4.62203799676284,-0.892631041062025,
1.2600507698021));
#58999=CARTESIAN_POINT('Ctrl Pts',(-4.59552345435715,-1.2793597226731,0.864729332189069));
#59000=CARTESIAN_POINT('Ctrl Pts',(-4.56900891195147,-1.41098813000681,
0.397535308255665));
#59001=CARTESIAN_POINT('Ctrl Pts',(-4.56172428991527,-1.44715180132278,
0.269178128642617));
#59002=CARTESIAN_POINT('Ctrl Pts',(-4.55443966787907,-1.46405988843861,
0.135395832802253));
#59003=CARTESIAN_POINT('Ctrl Pts',(-4.54715504584288,-1.46288856329395,
0.00132347729660035));
#59004=CARTESIAN_POINT('Origin',(-17.3,0.,0.));
#59005=CARTESIAN_POINT('',(-3.97584495415716,-1.46111494020071,-0.00025097937605606));
#59006=CARTESIAN_POINT('',(-4.04715504584288,-1.46122237770127,-0.000480703445675848));
#59007=CARTESIAN_POINT('',(-17.3,-1.4635,-1.79227059055215E-16));
#59008=CARTESIAN_POINT('Ctrl Pts',(-3.97584495415716,-1.46111494020071,
-0.00025097937605606));
#59009=CARTESIAN_POINT('Ctrl Pts',(-3.98992800491106,-1.46071820887633,
0.259737348729522));
#59010=CARTESIAN_POINT('Ctrl Pts',(-4.00401105566496,-1.39465998093067,
0.519913933469384));
#59011=CARTESIAN_POINT('Ctrl Pts',(-4.01809410641886,-1.26412505040052,
0.742232925278513));
#59012=CARTESIAN_POINT('Ctrl Pts',(-4.04460864882455,-1.01836338899302,
1.16079893337724));
#59013=CARTESIAN_POINT('Ctrl Pts',(-4.07112319123024,-0.544053634075698,
1.44517258451028));
#59014=CARTESIAN_POINT('Ctrl Pts',(-4.09763773363593,-0.0590651644775016,
1.46472972413441));
#59015=CARTESIAN_POINT('Ctrl Pts',(-4.12415227604161,0.425923305120695,
1.48428686375854));
#59016=CARTESIAN_POINT('Ctrl Pts',(-4.1506668184473,0.921590489399769,1.23902749187376));
#59017=CARTESIAN_POINT('Ctrl Pts',(-4.17718136085298,1.20025669080933,0.841609015270768));
#59018=CARTESIAN_POINT('Ctrl Pts',(-4.20369590325867,1.4789228922189,0.444190538667776));
#59019=CARTESIAN_POINT('Ctrl Pts',(-4.23021044566436,1.54058811075896,-0.10538704265343));
#59020=CARTESIAN_POINT('Ctrl Pts',(-4.25672498807004,1.3569270532653,-0.554680836638826));
#59021=CARTESIAN_POINT('Ctrl Pts',(-4.28323953047573,1.17326599577164,-1.00397463062425));
#59022=CARTESIAN_POINT('Ctrl Pts',(-4.30975407288142,0.744278662244238,
-1.35298463727385));
#59023=CARTESIAN_POINT('Ctrl Pts',(-4.3362686152871,0.267016036585803,-1.44139664722228));
#59024=CARTESIAN_POINT('Ctrl Pts',(-4.36278315769279,-0.210246589072633,
-1.52980865717071));
#59025=CARTESIAN_POINT('Ctrl Pts',(-4.38929770009848,-0.735784506862102,
-1.35762267041797));
#59026=CARTESIAN_POINT('Ctrl Pts',(-4.41581224250417,-1.06819720053174,
-1.00393057488741));
#59027=CARTESIAN_POINT('Ctrl Pts',(-4.4358231463885,-1.31907380858995,-0.736994098292163));
#59028=CARTESIAN_POINT('Ctrl Pts',(-4.45583405027283,-1.45994751527582,
-0.366672894645548));
#59029=CARTESIAN_POINT('Ctrl Pts',(-4.47584495415716,-1.46331444493144,
0.00135213804196392));
#59030=CARTESIAN_POINT('Ctrl Pts',(-4.54715504584288,-1.46288856329395,
0.00132347729660035));
#59031=CARTESIAN_POINT('Ctrl Pts',(-4.52792512547339,-1.45979650317788,
-0.352600268824065));
#59032=CARTESIAN_POINT('Ctrl Pts',(-4.5086952051039,-1.33071758853706,-0.708545303265838));
#59033=CARTESIAN_POINT('Ctrl Pts',(-4.48946528473441,-1.09728807987873,
-0.972049738483633));
#59034=CARTESIAN_POINT('Ctrl Pts',(-4.46295074232872,-0.775431489360546,
-1.33537415103575));
#59035=CARTESIAN_POINT('Ctrl Pts',(-4.43643619992304,-0.255190175267832,
-1.52295636588615));
#59036=CARTESIAN_POINT('Ctrl Pts',(-4.40992165751735,0.22446828737602,-1.44863239377439));
#59037=CARTESIAN_POINT('Ctrl Pts',(-4.38340711511166,0.704126750019844,
-1.37430842166264));
#59038=CARTESIAN_POINT('Ctrl Pts',(-4.35689257270597,1.14320236121478,-1.03807826258876));
#59039=CARTESIAN_POINT('Ctrl Pts',(-4.33037803030029,1.34001018895549,-0.594385832456929));
#59040=CARTESIAN_POINT('Ctrl Pts',(-4.3038634878946,1.53681801669619,-0.150693402325121));
#59041=CARTESIAN_POINT('Ctrl Pts',(-4.27734894548891,1.49135806098265,0.400461298864684));
#59042=CARTESIAN_POINT('Ctrl Pts',(-4.25083440308323,1.2245118917388,0.805910945030719));
#59043=CARTESIAN_POINT('Ctrl Pts',(-4.22431986067754,0.957665722494918,
1.2113605911968));
#59044=CARTESIAN_POINT('Ctrl Pts',(-4.19780531827186,0.469433339720774,
1.47110518233911));
#59045=CARTESIAN_POINT('Ctrl Pts',(-4.17129077586617,-0.0159206597535222,
1.46583367300764));
#59046=CARTESIAN_POINT('Ctrl Pts',(-4.14477623346049,-0.501274659227791,
1.46056216367617));
#59047=CARTESIAN_POINT('Ctrl Pts',(-4.1182616910548,-0.983750275402204,
1.19027455387084));
#59048=CARTESIAN_POINT('Ctrl Pts',(-4.09174714864911,-1.24172722383962,
0.779124717811985));
#59049=CARTESIAN_POINT('Ctrl Pts',(-4.07688311438036,-1.38634892401639,
0.548634401997345));
#59050=CARTESIAN_POINT('Ctrl Pts',(-4.06201908011162,-1.46041707087967,
0.273875090335108));
#59051=CARTESIAN_POINT('Ctrl Pts',(-4.04715504584288,-1.46122237770127,
-0.000480703445675848));
#59052=CARTESIAN_POINT('Origin',(-17.3,0.,0.));
#59053=CARTESIAN_POINT('',(-3.47584495415716,-1.46423846103291,-0.0012628549216627));
#59054=CARTESIAN_POINT('',(-3.54715504584288,-1.46465674957962,-0.0011499352553702));
#59055=CARTESIAN_POINT('',(-17.3,-1.4635,-1.79227059055215E-16));
#59056=CARTESIAN_POINT('Ctrl Pts',(-3.47584495415716,-1.46423846103291,
-0.0012628549216627));
#59057=CARTESIAN_POINT('Ctrl Pts',(-3.49750741714361,-1.46061129198041,
0.396491821226815));
#59058=CARTESIAN_POINT('Ctrl Pts',(-3.51916988013006,-1.29269684904186,
0.796941553735221));
#59059=CARTESIAN_POINT('Ctrl Pts',(-3.54083234311651,-1.00366072506953,
1.06845075102716));
#59060=CARTESIAN_POINT('Ctrl Pts',(-3.56734688552219,-0.649884676121027,
1.40077409439001));
#59061=CARTESIAN_POINT('Ctrl Pts',(-3.59386142792788,-0.114651306021696,
1.53992637284989));
#59062=CARTESIAN_POINT('Ctrl Pts',(-3.62037597033356,0.356185361221739,
1.42198939759372));
#59063=CARTESIAN_POINT('Ctrl Pts',(-3.64689051273925,0.827022028465174,
1.30405242233755));
#59064=CARTESIAN_POINT('Ctrl Pts',(-3.67340505514494,1.23346199285271,0.929026193365342));
#59065=CARTESIAN_POINT('Ctrl Pts',(-3.69991959755062,1.38881117598024,0.46917520809393));
#59066=CARTESIAN_POINT('Ctrl Pts',(-3.72643413995631,1.54416035910777,0.00932422282251724));
#59067=CARTESIAN_POINT('Ctrl Pts',(-3.752948682362,1.44841876097529,-0.535351518748095));
#59068=CARTESIAN_POINT('Ctrl Pts',(-3.77946322476768,1.14556431435133,-0.914660734973559));
#59069=CARTESIAN_POINT('Ctrl Pts',(-3.80597776717337,0.84270986772736,-1.29396995119905));
#59070=CARTESIAN_POINT('Ctrl Pts',(-3.83249230957905,0.332742572611882,
-1.50791264207935));
#59071=CARTESIAN_POINT('Ctrl Pts',(-3.85900685198474,-0.150089262462492,
-1.45821640085108));
#59072=CARTESIAN_POINT('Ctrl Pts',(-3.88552139439043,-0.632921097536866,
-1.4085201596228));
#59073=CARTESIAN_POINT('Ctrl Pts',(-3.91203593679612,-1.08861747257013,
-1.09518498628594));
#59074=CARTESIAN_POINT('Ctrl Pts',(-3.93855047920181,-1.30785887613792,
-0.662138217085276));
#59075=CARTESIAN_POINT('Ctrl Pts',(-3.95098197085359,-1.41065143565023,
-0.459101814880751));
#59076=CARTESIAN_POINT('Ctrl Pts',(-3.96341346250538,-1.46146514572316,
-0.229749742597532));
#59077=CARTESIAN_POINT('Ctrl Pts',(-3.97584495415716,-1.46111494020071,
-0.00025097937605606));
#59078=CARTESIAN_POINT('Ctrl Pts',(-4.04715504584288,-1.46122237770127,
-0.000480703445675848));
#59079=CARTESIAN_POINT('Ctrl Pts',(-4.03550453770593,-1.46185358141812,
-0.215522215734277));
#59080=CARTESIAN_POINT('Ctrl Pts',(-4.02385402956899,-1.41747570995839,
-0.430315826540335));
#59081=CARTESIAN_POINT('Ctrl Pts',(-4.01220352143205,-1.32678415700106,
-0.623350322901187));
#59082=CARTESIAN_POINT('Ctrl Pts',(-3.98568897902636,-1.12038586102462,
-1.06266346524309));
#59083=CARTESIAN_POINT('Ctrl Pts',(-3.95917443662068,-0.674110988371246,
-1.3892776876145));
#59084=CARTESIAN_POINT('Ctrl Pts',(-3.93265989421499,-0.192951378833284,
-1.45316605717873));
#59085=CARTESIAN_POINT('Ctrl Pts',(-3.9061453518093,0.288208230704705,-1.51705442674297));
#59086=CARTESIAN_POINT('Ctrl Pts',(-3.87963080940361,0.804252577127286,
-1.3182169435));
#59087=CARTESIAN_POINT('Ctrl Pts',(-3.85311626699793,1.11814191997438,-0.947987590175135));
#59088=CARTESIAN_POINT('Ctrl Pts',(-3.82660172459224,1.43203126282145,-0.57775823685029));
#59089=CARTESIAN_POINT('Ctrl Pts',(-3.80008718218656,1.54376560209305,-0.0361370134435621));
#59090=CARTESIAN_POINT('Ctrl Pts',(-3.77357263978087,1.40202090146358,0.42808786036197));
#59091=CARTESIAN_POINT('Ctrl Pts',(-3.74705809737518,1.26027620083411,0.892312734167503));
#59092=CARTESIAN_POINT('Ctrl Pts',(-3.7205435549695,0.865052460303565,1.27914125837184));
#59093=CARTESIAN_POINT('Ctrl Pts',(-3.69402901256381,0.397891699522902,
1.4108876708586));
#59094=CARTESIAN_POINT('Ctrl Pts',(-3.66751447015812,-0.069269061257761,
1.54263408334537));
#59095=CARTESIAN_POINT('Ctrl Pts',(-3.64099992775244,-0.608366842288541,
1.41929838411456));
#59096=CARTESIAN_POINT('Ctrl Pts',(-3.61448538534675,-0.971772541566861,
1.09753357661018));
#59097=CARTESIAN_POINT('Ctrl Pts',(-3.59204193884546,-1.27938020249592,
0.825173181596368));
#59098=CARTESIAN_POINT('Ctrl Pts',(-3.56959849234417,-1.46110604285371,
0.41064008787777));
#59099=CARTESIAN_POINT('Ctrl Pts',(-3.54715504584288,-1.46465674957962,
-0.0011499352553702));
#59100=CARTESIAN_POINT('Origin',(-17.3,0.,0.));
#59101=CARTESIAN_POINT('',(-2.97584495415716,-1.46529038421007,0.000858184953542052));
#59102=CARTESIAN_POINT('',(-3.04715504584288,-1.46493873305747,0.00104194039951338));
#59103=CARTESIAN_POINT('',(-17.3,-1.4635,-1.79227059055215E-16));
#59104=CARTESIAN_POINT('Ctrl Pts',(-2.97584495415716,-1.46529038421007,
0.000858184953542052));
#59105=CARTESIAN_POINT('Ctrl Pts',(-2.97857228697047,-1.46563784872126,
0.0508424879856784));
#59106=CARTESIAN_POINT('Ctrl Pts',(-2.98129961978378,-1.46330283124409,
0.10079394579702));
#59107=CARTESIAN_POINT('Ctrl Pts',(-2.98402695259709,-1.45817844302379,
0.150457591094951));
#59108=CARTESIAN_POINT('Ctrl Pts',(-3.01054149500277,-1.40836024404669,
0.633276857906377));
#59109=CARTESIAN_POINT('Ctrl Pts',(-3.03705603740846,-1.09490997556484,
1.08889407252482));
#59110=CARTESIAN_POINT('Ctrl Pts',(-3.06357057981415,-0.66180784161105,
1.30802608506082));
#59111=CARTESIAN_POINT('Ctrl Pts',(-3.09008512221983,-0.228705707657263,
1.52715809759682));
#59112=CARTESIAN_POINT('Ctrl Pts',(-3.11659966462552,0.324048291768454,
1.50980490805039));
#59113=CARTESIAN_POINT('Ctrl Pts',(-3.1431142070312,0.74255220914835,1.26393752816612));
#59114=CARTESIAN_POINT('Ctrl Pts',(-3.16962874943689,1.16105612652827,1.01807014828184));
#59115=CARTESIAN_POINT('Ctrl Pts',(-3.19614329184258,1.44530996186235,0.543688578059681));
#59116=CARTESIAN_POINT('Ctrl Pts',(-3.22265783424827,1.46474459678038,0.0586951839612338));
#59117=CARTESIAN_POINT('Ctrl Pts',(-3.24917237665395,1.48417923169841,-0.426298210137186));
#59118=CARTESIAN_POINT('Ctrl Pts',(-3.27568691905964,1.23879466620043,-0.921903428111893));
#59119=CARTESIAN_POINT('Ctrl Pts',(-3.30220146146532,0.841305813494467,
-1.20046923600649));
#59120=CARTESIAN_POINT('Ctrl Pts',(-3.32871600387101,0.443816960788507,
-1.47903504390108));
#59121=CARTESIAN_POINT('Ctrl Pts',(-3.3552305462767,-0.105776179125424,
-1.54056144171556));
#59122=CARTESIAN_POINT('Ctrl Pts',(-3.38174508868239,-0.555023567511395,
-1.35678690217903));
#59123=CARTESIAN_POINT('Ctrl Pts',(-3.40825963108808,-1.00427095589739,
-1.17301236264248));
#59124=CARTESIAN_POINT('Ctrl Pts',(-3.43477417349376,-1.35317259275541,
-0.743936885754905));
#59125=CARTESIAN_POINT('Ctrl Pts',(-3.46128871589945,-1.44146404728557,
-0.266651943178191));
#59126=CARTESIAN_POINT('Ctrl Pts',(-3.46614079531868,-1.45762111094013,
-0.179310271896277));
#59127=CARTESIAN_POINT('Ctrl Pts',(-3.47099287473792,-1.46505089461079,
-0.0903541682802729));
#59128=CARTESIAN_POINT('Ctrl Pts',(-3.47584495415716,-1.46423846103291,
-0.0012628549216627));
#59129=CARTESIAN_POINT('Ctrl Pts',(-3.54715504584288,-1.46465674957962,
-0.0011499352553702));
#59130=CARTESIAN_POINT('Ctrl Pts',(-3.54308394993848,-1.46530082479368,
-0.075845979668695));
#59131=CARTESIAN_POINT('Ctrl Pts',(-3.53901285403409,-1.46008229464905,
-0.150451767153425));
#59132=CARTESIAN_POINT('Ctrl Pts',(-3.53494175812969,-1.44868904639678,
-0.224102367635917));
#59133=CARTESIAN_POINT('Ctrl Pts',(-3.508427215724,-1.3744862344225,-0.703779588599594));
#59134=CARTESIAN_POINT('Ctrl Pts',(-3.48191267331832,-1.03836699294809,
-1.14294011474894));
#59135=CARTESIAN_POINT('Ctrl Pts',(-3.45539813091263,-0.594724289002558,
-1.33986000925486));
#59136=CARTESIAN_POINT('Ctrl Pts',(-3.42888358850694,-0.151081585057076,
-1.53677990376077));
#59137=CARTESIAN_POINT('Ctrl Pts',(-3.40236904610126,0.400084581359495,
-1.49145916662331));
#59138=CARTESIAN_POINT('Ctrl Pts',(-3.37585450369557,0.805601617729781,
-1.22471541912446));
#59139=CARTESIAN_POINT('Ctrl Pts',(-3.34933996128989,1.21111865410007,-0.957971671625605));
#59140=CARTESIAN_POINT('Ctrl Pts',(-3.32282541888421,1.47098656042407,-0.469804913765352));
#59141=CARTESIAN_POINT('Ctrl Pts',(-3.29631087647852,1.46583764767282,0.0155504017651938));
#59142=CARTESIAN_POINT('Ctrl Pts',(-3.26979633407283,1.46068873492156,0.500905717295823));
#59143=CARTESIAN_POINT('Ctrl Pts',(-3.24328179166714,1.19052300309495,0.983449590496744));
#59144=CARTESIAN_POINT('Ctrl Pts',(-3.21676724926145,0.779438342998958,
1.24153038375752));
#59145=CARTESIAN_POINT('Ctrl Pts',(-3.19025270685576,0.368353682903008,
1.49961117701827));
#59146=CARTESIAN_POINT('Ctrl Pts',(-3.16373816445008,-0.183649905462294,
1.53322889033894));
#59147=CARTESIAN_POINT('Ctrl Pts',(-3.13722362204439,-0.623015168294578,
1.32694156781861));
#59148=CARTESIAN_POINT('Ctrl Pts',(-3.11070907963871,-1.06238043112686,
1.12065424529827));
#59149=CARTESIAN_POINT('Ctrl Pts',(-3.08419453723302,-1.38910736842613,
0.674461886936952));
#59150=CARTESIAN_POINT('Ctrl Pts',(-3.05767999482733,-1.45311727289601,
0.193318430423119));
#59151=CARTESIAN_POINT('Ctrl Pts',(-3.05417167849918,-1.46158685119682,
0.129655123742453));
#59152=CARTESIAN_POINT('Ctrl Pts',(-3.05066336217103,-1.46545685722587,
0.0653799035508948));
#59153=CARTESIAN_POINT('Ctrl Pts',(-3.04715504584288,-1.46493873305747,
0.00104194039951338));
#59154=CARTESIAN_POINT('Origin',(-17.3,0.,0.));
#59155=CARTESIAN_POINT('',(-2.47584495415716,-1.46155994553451,0.000838156444187416));
#59156=CARTESIAN_POINT('',(-2.54715504584288,-1.46134104288809,0.000637616632206692));
#59157=CARTESIAN_POINT('',(-17.3,-1.4635,-1.79227059055215E-16));
#59158=CARTESIAN_POINT('Ctrl Pts',(-2.47584495415716,-1.46155994553451,
0.000838156444187416));
#59159=CARTESIAN_POINT('Ctrl Pts',(-2.48615169920302,-1.46254670497474,
0.190967096739963));
#59160=CARTESIAN_POINT('Ctrl Pts',(-2.49645844424887,-1.42812769578372,
0.38075266272535));
#59161=CARTESIAN_POINT('Ctrl Pts',(-2.50676518929473,-1.35664666452184,
0.555366262980827));
#59162=CARTESIAN_POINT('Ctrl Pts',(-2.53327973170041,-1.1727586546639,1.00456721711192));
#59163=CARTESIAN_POINT('Ctrl Pts',(-2.5597942741061,-0.743595061800773,
1.35336046190046));
#59164=CARTESIAN_POINT('Ctrl Pts',(-2.58630881651179,-0.266287832759806,
1.44153135537509));
#59165=CARTESIAN_POINT('Ctrl Pts',(-2.61282335891747,0.211019396281106,
1.5297022488497));
#59166=CARTESIAN_POINT('Ctrl Pts',(-2.63933790132316,0.736470261499846,
1.35725079101045));
#59167=CARTESIAN_POINT('Ctrl Pts',(-2.66585244372885,1.06870423335387,1.00339081121795));
#59168=CARTESIAN_POINT('Ctrl Pts',(-2.69236698613453,1.40093820520792,0.649530831425438));
#59169=CARTESIAN_POINT('Ctrl Pts',(-2.71888152854022,1.53995528369721,0.114262329679646));
#59170=CARTESIAN_POINT('Ctrl Pts',(-2.7453960709459,1.42189938274908,-0.35654453263864));
#59171=CARTESIAN_POINT('Ctrl Pts',(-2.77191061335159,1.30384348180092,-0.82735139495698));
#59172=CARTESIAN_POINT('Ctrl Pts',(-2.79842515575728,0.928714601415265,
-1.2336966178478));
#59173=CARTESIAN_POINT('Ctrl Pts',(-2.82493969816297,0.468824390893206,
-1.38892964145764));
#59174=CARTESIAN_POINT('Ctrl Pts',(-2.85145424056866,0.00893418037119946,
-1.54416266506747));
#59175=CARTESIAN_POINT('Ctrl Pts',(-2.87796878297434,-0.535717360287188,
-1.44828348939639));
#59176=CARTESIAN_POINT('Ctrl Pts',(-2.90448332538003,-0.914950065880211,
-1.14533324205864));
#59177=CARTESIAN_POINT('Ctrl Pts',(-2.92827053497241,-1.2551742234086,-0.873544993963514));
#59178=CARTESIAN_POINT('Ctrl Pts',(-2.95205774456478,-1.46225987355395,
-0.435094144278848));
#59179=CARTESIAN_POINT('Ctrl Pts',(-2.97584495415716,-1.46529038421007,
0.000858184953542052));
#59180=CARTESIAN_POINT('Ctrl Pts',(-3.04715504584288,-1.46493873305747,
0.00104194039951338));
#59181=CARTESIAN_POINT('Ctrl Pts',(-3.02414881976534,-1.46154106858268,
-0.420862354190906));
#59182=CARTESIAN_POINT('Ctrl Pts',(-3.00114259368781,-1.2694430210697,-0.845464750254815));
#59183=CARTESIAN_POINT('Ctrl Pts',(-2.97813636761028,-0.948269993348118,
-1.11790243046778));
#59184=CARTESIAN_POINT('Ctrl Pts',(-2.95162182520459,-0.578119937689832,
-1.4318852801785));
#59185=CARTESIAN_POINT('Ctrl Pts',(-2.9251072827989,-0.036526954732755,
-1.5437564249336));
#59186=CARTESIAN_POINT('Ctrl Pts',(-2.89859274039322,0.427733707804147,
-1.40212898819544));
#59187=CARTESIAN_POINT('Ctrl Pts',(-2.87207819798753,0.89199437034105,-1.26050155145728));
#59188=CARTESIAN_POINT('Ctrl Pts',(-2.84556365558184,1.27892271245777,-0.865375533225857));
#59189=CARTESIAN_POINT('Ctrl Pts',(-2.81904911317616,1.41078712169197,-0.398248065403867));
#59190=CARTESIAN_POINT('Ctrl Pts',(-2.79253457077047,1.54265153092617,0.068879402418151));
#59191=CARTESIAN_POINT('Ctrl Pts',(-2.76602002836478,1.41945200727779,0.608008319830747));
#59192=CARTESIAN_POINT('Ctrl Pts',(-2.7395054859591,1.09777900331638,0.971495282648806));
#59193=CARTESIAN_POINT('Ctrl Pts',(-2.71299094355341,0.776105999355004,
1.33498224546682));
#59194=CARTESIAN_POINT('Ctrl Pts',(-2.68647640114773,0.255959515080636,
1.52282725369035));
#59195=CARTESIAN_POINT('Ctrl Pts',(-2.65996185874204,-0.223736433597789,
1.44874560658848));
#59196=CARTESIAN_POINT('Ctrl Pts',(-2.63344731633635,-0.703432382276295,
1.37466395948659));
#59197=CARTESIAN_POINT('Ctrl Pts',(-2.60693277393067,-1.14267779535884,
1.03865565705922));
#59198=CARTESIAN_POINT('Ctrl Pts',(-2.58041823152498,-1.33970974406678,
0.59506270760455));
#59199=CARTESIAN_POINT('Ctrl Pts',(-2.56933050296428,-1.42210365196957,
0.409563062174604));
#59200=CARTESIAN_POINT('Ctrl Pts',(-2.55824277440358,-1.46214153647667,
0.205250020725279));
#59201=CARTESIAN_POINT('Ctrl Pts',(-2.54715504584288,-1.46134104288809,
0.000637616632206692));
#59202=CARTESIAN_POINT('Origin',(-17.3,0.,0.));
#59203=CARTESIAN_POINT('',(-1.97584495415716,-1.46221851409551,-0.00117471765568408));
#59204=CARTESIAN_POINT('',(-2.04715504584289,-1.46259601224811,-0.00127585584471357));
#59205=CARTESIAN_POINT('',(-17.3,-1.4635,-1.79227059055215E-16));
#59206=CARTESIAN_POINT('Ctrl Pts',(-1.97584495415716,-1.46221851409551,
-0.00117471765568408));
#59207=CARTESIAN_POINT('Ctrl Pts',(-1.99373111143557,-1.45974902951182,
0.328398847612615));
#59208=CARTESIAN_POINT('Ctrl Pts',(-2.01161726871397,-1.3495306267837,0.659468494052664));
#59209=CARTESIAN_POINT('Ctrl Pts',(-2.02950342599237,-1.14510209648561,
0.91523933882229));
#59210=CARTESIAN_POINT('Ctrl Pts',(-2.05601796839806,-0.842056067584495,
1.29439550994524));
#59211=CARTESIAN_POINT('Ctrl Pts',(-2.08253251080374,-0.331980757629562,
1.50808054568027));
#59212=CARTESIAN_POINT('Ctrl Pts',(-2.10904705320943,0.150825910019734,
1.45814039194405));
#59213=CARTESIAN_POINT('Ctrl Pts',(-2.13556159561512,0.633632577669058,
1.40820023820784));
#59214=CARTESIAN_POINT('Ctrl Pts',(-2.16207613802081,1.08917060301271,1.09463489500037));
#59215=CARTESIAN_POINT('Ctrl Pts',(-2.1885906804265,1.3081932105853,0.661477424025895));
#59216=CARTESIAN_POINT('Ctrl Pts',(-2.21510522283218,1.52721581815786,0.228319953051469));
#59217=CARTESIAN_POINT('Ctrl Pts',(-2.24161976523787,1.50972300795938,-0.324429645689988));
#59218=CARTESIAN_POINT('Ctrl Pts',(-2.26813430764355,1.26374992525915,-0.742871445701784));
#59219=CARTESIAN_POINT('Ctrl Pts',(-2.29464885004924,1.01777684255889,-1.16131324571363));
#59220=CARTESIAN_POINT('Ctrl Pts',(-2.32116339245492,0.543323487356945,
-1.4454472469958));
#59221=CARTESIAN_POINT('Ctrl Pts',(-2.34767793486061,0.0583251997158712,
-1.46475937594014));
#59222=CARTESIAN_POINT('Ctrl Pts',(-2.3741924772663,-0.426673087925147,
-1.48407150488447));
#59223=CARTESIAN_POINT('Ctrl Pts',(-2.40070701967198,-0.922216308005284,
-1.23856176149093));
#59224=CARTESIAN_POINT('Ctrl Pts',(-2.42722156207767,-1.20068170461892,
-0.841002558057389));
#59225=CARTESIAN_POINT('Ctrl Pts',(-2.4434293594375,-1.37090190495213,-0.597982749938599));
#59226=CARTESIAN_POINT('Ctrl Pts',(-2.45963715679733,-1.46000822411528,
-0.298147733169239));
#59227=CARTESIAN_POINT('Ctrl Pts',(-2.47584495415716,-1.46155994553451,
0.000838156444187416));
#59228=CARTESIAN_POINT('Ctrl Pts',(-2.54715504584288,-1.46134104288809,
0.000637616632206692));
#59229=CARTESIAN_POINT('Ctrl Pts',(-2.53172823199789,-1.46022728315745,
-0.284048056455808));
#59230=CARTESIAN_POINT('Ctrl Pts',(-2.5163014181529,-1.38005734937291,-0.569313244852052));
#59231=CARTESIAN_POINT('Ctrl Pts',(-2.50087460430791,-1.22491886837172,
-0.805292239031575));
#59232=CARTESIAN_POINT('Ctrl Pts',(-2.47436006190223,-0.958277559635383,
-1.21087663973118));
#59233=CARTESIAN_POINT('Ctrl Pts',(-2.44784551949654,-0.47017645782932,
-1.47086784464852));
#59234=CARTESIAN_POINT('Ctrl Pts',(-2.42133097709086,0.0151801427879505,
-1.46584152880958));
#59235=CARTESIAN_POINT('Ctrl Pts',(-2.39481643468517,0.500536743405221,
-1.46081521297064));
#59236=CARTESIAN_POINT('Ctrl Pts',(-2.36830189227948,0.983148842833728,
-1.19077137637541));
#59237=CARTESIAN_POINT('Ctrl Pts',(-2.3417873498738,1.2413334644567,-0.779751918463746));
#59238=CARTESIAN_POINT('Ctrl Pts',(-2.31527280746811,1.49951808607968,-0.368732460552062));
#59239=CARTESIAN_POINT('Ctrl Pts',(-2.28875826506243,1.53327522989713,0.183262618676012));
#59240=CARTESIAN_POINT('Ctrl Pts',(-2.26224372265674,1.32709889398495,0.622679973952962));
#59241=CARTESIAN_POINT('Ctrl Pts',(-2.23572918025105,1.12092255807279,1.06209732922989));
#59242=CARTESIAN_POINT('Ctrl Pts',(-2.20921463784537,0.674812742430977,
1.38893696055564));
#59243=CARTESIAN_POINT('Ctrl Pts',(-2.18270009543968,0.193685469657787,
1.45306839587207));
#59244=CARTESIAN_POINT('Ctrl Pts',(-2.156185553034,-0.28744180311543,1.51719983118851));
#59245=CARTESIAN_POINT('Ctrl Pts',(-2.12967101062831,-0.803586533020062,
1.31862307049558));
#59246=CARTESIAN_POINT('Ctrl Pts',(-2.10315646822262,-1.11766286959625,
0.948552336073166));
#59247=CARTESIAN_POINT('Ctrl Pts',(-2.08448932742938,-1.33878330626034,
0.688009936463793));
#59248=CARTESIAN_POINT('Ctrl Pts',(-2.06582218663613,-1.45974572493651,
0.342464156450928));
#59249=CARTESIAN_POINT('Ctrl Pts',(-2.04715504584289,-1.46259601224811,
-0.00127585584471357));
#59250=CARTESIAN_POINT('Origin',(-17.3,0.,0.));
#59251=CARTESIAN_POINT('',(-1.47584495415717,-1.46581513481851,-0.000356810360598175));
#59252=CARTESIAN_POINT('',(-1.54715504584288,-1.46591291273786,-9.23842247488784E-5));
#59253=CARTESIAN_POINT('',(-17.3,-1.4635,-1.79227059055215E-16));
#59254=CARTESIAN_POINT('Ctrl Pts',(-1.47584495415717,-1.46581513481851,
-0.000356810360598175));
#59255=CARTESIAN_POINT('Ctrl Pts',(-1.50131052366812,-1.46429011704063,
0.465912677307333));
#59256=CARTESIAN_POINT('Ctrl Pts',(-1.52677609317907,-1.22259768826152,
0.933541855018993));
#59257=CARTESIAN_POINT('Ctrl Pts',(-1.55224166269002,-0.840699239369595,
1.20089411587294));
#59258=CARTESIAN_POINT('Ctrl Pts',(-1.5787562050957,-0.443069702223083,
1.47925910019502));
#59259=CARTESIAN_POINT('Ctrl Pts',(-1.60527074750139,0.106554431146246,
1.54050780744101));
#59260=CARTESIAN_POINT('Ctrl Pts',(-1.63178528990707,0.555708917962632,
1.35650633016601));
#59261=CARTESIAN_POINT('Ctrl Pts',(-1.65829983231276,1.00486340477899,1.17250485289101));
#59262=CARTESIAN_POINT('Ctrl Pts',(-1.68481437471845,1.35354824504234,0.743253191095036));
#59263=CARTESIAN_POINT('Ctrl Pts',(-1.71132891712413,1.44159857415386,0.265923710694476));
#59264=CARTESIAN_POINT('Ctrl Pts',(-1.73784345952982,1.52964890326539,-0.211405769706084));
#59265=CARTESIAN_POINT('Ctrl Pts',(-1.7643580019355,1.35706472122508,-0.736813068711231));
#59266=CARTESIAN_POINT('Ctrl Pts',(-1.79087254434119,1.00312083194446,-1.06895765030956));
#59267=CARTESIAN_POINT('Ctrl Pts',(-1.81738708674688,0.649176942663795,
-1.40110223190793));
#59268=CARTESIAN_POINT('Ctrl Pts',(-1.84390162915257,0.11387334614275,-1.53998409609945));
#59269=CARTESIAN_POINT('Ctrl Pts',(-1.87041617155826,-0.356903680568287,
-1.4218092757004));
#59270=CARTESIAN_POINT('Ctrl Pts',(-1.89693071396394,-0.827680707279217,
-1.30363445530139));
#59271=CARTESIAN_POINT('Ctrl Pts',(-1.92344525636963,-1.2339311641802,-0.92840295031193));
#59272=CARTESIAN_POINT('Ctrl Pts',(-1.94995979877531,-1.38904801870709,
-0.468473544561806));
#59273=CARTESIAN_POINT('Ctrl Pts',(-1.95858818390259,-1.43952627852816,
-0.318802922928734));
#59274=CARTESIAN_POINT('Ctrl Pts',(-1.96721656902988,-1.46340980765971,
-0.160162900787707));
#59275=CARTESIAN_POINT('Ctrl Pts',(-1.97584495415716,-1.46221851409551,
-0.00117471765568408));
#59276=CARTESIAN_POINT('Ctrl Pts',(-2.04715504584289,-1.46259601224811,
-0.00127585584471357));
#59277=CARTESIAN_POINT('Ctrl Pts',(-2.03930764423044,-1.46379423266615,
-0.145779288728592));
#59278=CARTESIAN_POINT('Ctrl Pts',(-2.031460242618,-1.44411917499234,-0.289963598662981));
#59279=CARTESIAN_POINT('Ctrl Pts',(-2.02361284100556,-1.40223698554355,
-0.427379528058853));
#59280=CARTESIAN_POINT('Ctrl Pts',(-1.99709829859987,-1.26072682166689,
-0.891675949616525));
#59281=CARTESIAN_POINT('Ctrl Pts',(-1.97058375619419,-0.865698550665846,
-1.27870408457996));
#59282=CARTESIAN_POINT('Ctrl Pts',(-1.9440692137885,-0.398604405731616,
-1.41068648231822));
#59283=CARTESIAN_POINT('Ctrl Pts',(-1.91755467138282,0.0684897392025882,
-1.54266888005647));
#59284=CARTESIAN_POINT('Ctrl Pts',(-1.89104012897713,0.607649758069999,
-1.41960554056952));
#59285=CARTESIAN_POINT('Ctrl Pts',(-1.86452558657144,0.971217961473909,
-1.09802436035208));
#59286=CARTESIAN_POINT('Ctrl Pts',(-1.83801104416575,1.33478616487784,-0.776443180134614));
#59287=CARTESIAN_POINT('Ctrl Pts',(-1.81149650176006,1.52276255281831,-0.256344159186644));
#59288=CARTESIAN_POINT('Ctrl Pts',(-1.78498195935438,1.44880207486443,0.22337048598841));
#59289=CARTESIAN_POINT('Ctrl Pts',(-1.75846741694869,1.37484159691055,0.703085131163465));
#59290=CARTESIAN_POINT('Ctrl Pts',(-1.73195287454301,1.03894425306233,1.14241540056557));
#59291=CARTESIAN_POINT('Ctrl Pts',(-1.70543833213732,0.595401087256812,
1.33955939206657));
#59292=CARTESIAN_POINT('Ctrl Pts',(-1.67892378973163,0.151857921451289,
1.53670338356758));
#59293=CARTESIAN_POINT('Ctrl Pts',(-1.65240924732594,-0.399331066311595,
1.49166109716746));
#59294=CARTESIAN_POINT('Ctrl Pts',(-1.62589470492026,-0.804982807087559,
1.22512224200014));
#59295=CARTESIAN_POINT('Ctrl Pts',(-1.59964815189446,-1.20653452015798,
0.961277364402592));
#59296=CARTESIAN_POINT('Ctrl Pts',(-1.57340159886867,-1.46547608429131,
0.480390737597124));
#59297=CARTESIAN_POINT('Ctrl Pts',(-1.54715504584288,-1.46591291273786,
-9.23842247488784E-5));
#59298=CARTESIAN_POINT('Origin',(-17.3,0.,0.));
#59299=CARTESIAN_POINT('',(-0.975844954157165,-1.4632995300711,0.00135195255092181));
#59300=CARTESIAN_POINT('',(-1.04715504584289,-1.46287428079508,0.00132175412439906));
#59301=CARTESIAN_POINT('',(-17.3,-1.4635,-1.79227059055215E-16));
#59302=CARTESIAN_POINT('Ctrl Pts',(-0.975844954157165,-1.4632995300711,
0.00135195255092181));
#59303=CARTESIAN_POINT('Ctrl Pts',(-0.982375393494976,-1.4643975106379,
0.121457105082137));
#59304=CARTESIAN_POINT('Ctrl Pts',(-0.988905832832787,-1.4508550804661,
0.241318079550921));
#59305=CARTESIAN_POINT('Ctrl Pts',(-0.995436272170598,-1.42171992921314,
0.357261097571569));
#59306=CARTESIAN_POINT('Ctrl Pts',(-1.02195081457628,-1.30342693797136,
0.828006771626319));
#59307=CARTESIAN_POINT('Ctrl Pts',(-1.04846535698197,-0.928091181909397,
1.23416574829629));
#59308=CARTESIAN_POINT('Ctrl Pts',(-1.07497989938765,-0.468122219837597,
1.38916720728875));
#59309=CARTESIAN_POINT('Ctrl Pts',(-1.10149444179334,-0.00815325776574491,
1.54416866628123));
#59310=CARTESIAN_POINT('Ctrl Pts',(-1.12800898419903,0.536448910315971,
1.44801260759614));
#59311=CARTESIAN_POINT('Ctrl Pts',(-1.15452352660471,0.915528317071882,
1.14487040370153));
#59312=CARTESIAN_POINT('Ctrl Pts',(-1.1810380690104,1.29460772382779,0.841728199806911));
#59313=CARTESIAN_POINT('Ctrl Pts',(-1.20755261141609,1.5081643692579,0.331599850702771));
#59314=CARTESIAN_POINT('Ctrl Pts',(-1.23406715382178,1.45810237232685,-0.15119396951098));
#59315=CARTESIAN_POINT('Ctrl Pts',(-1.26058169622746,1.4080403753958,-0.633987789724676));
#59316=CARTESIAN_POINT('Ctrl Pts',(-1.28709623863315,1.09435973610365,-1.08944708104799));
#59317=CARTESIAN_POINT('Ctrl Pts',(-1.31361078103884,0.661146898645242,
-1.30836038425853));
#59318=CARTESIAN_POINT('Ctrl Pts',(-1.34012532344452,0.227934061186759,
-1.52727368746911));
#59319=CARTESIAN_POINT('Ctrl Pts',(-1.36663986585021,-0.324810974438033,
-1.50964100256683));
#59320=CARTESIAN_POINT('Ctrl Pts',(-1.3931544082559,-0.743190600300525,
-1.26356217237913));
#59321=CARTESIAN_POINT('Ctrl Pts',(-1.41966895066158,-1.16157022616292,
-1.01748334219149));
#59322=CARTESIAN_POINT('Ctrl Pts',(-1.44618349306727,-1.44558444226309,
-0.542958366718559));
#59323=CARTESIAN_POINT('Ctrl Pts',(-1.47269803547295,-1.46477407985142,
-0.0579552482830333));
#59324=CARTESIAN_POINT('Ctrl Pts',(-1.47374700836769,-1.4655332635998,-0.0387674713522122));
#59325=CARTESIAN_POINT('Ctrl Pts',(-1.47479598126243,-1.46587795306069,
-0.0195632943937738));
#59326=CARTESIAN_POINT('Ctrl Pts',(-1.47584495415717,-1.46581513481851,
-0.000356810360598175));
#59327=CARTESIAN_POINT('Ctrl Pts',(-1.54715504584288,-1.46591291273786,
-9.23842247488784E-5));
#59328=CARTESIAN_POINT('Ctrl Pts',(-1.54688705646299,-1.46591737295725,
-0.0049983379223528));
#59329=CARTESIAN_POINT('Ctrl Pts',(-1.54661906708309,-1.46589488315485,
-0.00990424955315265));
#59330=CARTESIAN_POINT('Ctrl Pts',(-1.5463510777032,-1.46584531996366,-0.0148098876518666));
#59331=CARTESIAN_POINT('Ctrl Pts',(-1.51983653529752,-1.46094159827471,
-0.500167738202059));
#59332=CARTESIAN_POINT('Ctrl Pts',(-1.49332199289183,-1.19101966110771,
-0.982848015367965));
#59333=CARTESIAN_POINT('Ctrl Pts',(-1.46680745048614,-0.780065437455982,
-1.24113645682674));
#59334=CARTESIAN_POINT('Ctrl Pts',(-1.44029290808046,-0.369111213804236,
-1.49942489828552));
#59335=CARTESIAN_POINT('Ctrl Pts',(-1.41377836567477,0.182875296332269,
-1.53332150403716));
#59336=CARTESIAN_POINT('Ctrl Pts',(-1.38726382326908,0.622344727124077,
-1.32725615280541));
#59337=CARTESIAN_POINT('Ctrl Pts',(-1.36074928086339,1.06181415791586,-1.12119080157368));
#59338=CARTESIAN_POINT('Ctrl Pts',(-1.33423473845771,1.38876650936299,-0.675163493358575));
#59339=CARTESIAN_POINT('Ctrl Pts',(-1.30772019605202,1.45301945035473,-0.194052463649122));
#59340=CARTESIAN_POINT('Ctrl Pts',(-1.28120565364634,1.51727239134647,0.287058566060359));
#59341=CARTESIAN_POINT('Ctrl Pts',(-1.25469111124065,1.31882592188284,0.803253317264156));
#59342=CARTESIAN_POINT('Ctrl Pts',(-1.22817656883496,0.948834572316278,
1.1174231749986));
#59343=CARTESIAN_POINT('Ctrl Pts',(-1.20166202642928,0.578843222749738,
1.43159303273303));
#59344=CARTESIAN_POINT('Ctrl Pts',(-1.17514748402359,0.0373069930802804,
1.54373799699806));
#59345=CARTESIAN_POINT('Ctrl Pts',(-1.1486329416179,-0.427025233810471,
1.40234501189082));
#59346=CARTESIAN_POINT('Ctrl Pts',(-1.12211839921221,-0.89135746070125,
1.26095202678357));
#59347=CARTESIAN_POINT('Ctrl Pts',(-1.09560385680653,-1.27848568481334,
0.866021092304002));
#59348=CARTESIAN_POINT('Ctrl Pts',(-1.06908931440084,-1.41058591850998,
0.398960495781479));
#59349=CARTESIAN_POINT('Ctrl Pts',(-1.06177789154819,-1.44701274619994,
0.270167870710371));
#59350=CARTESIAN_POINT('Ctrl Pts',(-1.05446646869554,-1.46404753918599,
0.135890589201196));
#59351=CARTESIAN_POINT('Ctrl Pts',(-1.04715504584289,-1.46287428079508,
0.00132175412439906));
#59352=CARTESIAN_POINT('Origin',(-17.3,0.,0.));
#59353=CARTESIAN_POINT('',(-0.47584495415717,-1.4610556053668,-0.000134560743048767));
#59354=CARTESIAN_POINT('',(-0.547155045842891,-1.46121426462895,-0.000470658046818673));
#59355=CARTESIAN_POINT('',(-17.3,-1.4635,-1.79227059055215E-16));
#59356=CARTESIAN_POINT('Ctrl Pts',(-0.47584495415717,-1.4610556053668,-0.000134560743048767));
#59357=CARTESIAN_POINT('Ctrl Pts',(-0.489954805727525,-1.46067797988535,
0.260281498090399));
#59358=CARTESIAN_POINT('Ctrl Pts',(-0.504064657297881,-1.39440376469311,
0.520857511314463));
#59359=CARTESIAN_POINT('Ctrl Pts',(-0.518174508868237,-1.26341397229026,
0.743430076950993));
#59360=CARTESIAN_POINT('Ctrl Pts',(-0.544689051273926,-1.01726436624661,
1.16167754755594));
#59361=CARTESIAN_POINT('Ctrl Pts',(-0.571203593679616,-0.542590552750608,
1.44572691447813));
#59362=CARTESIAN_POINT('Ctrl Pts',(-0.597718136085304,-0.0575643430575941,
1.46483074051128));
#59363=CARTESIAN_POINT('Ctrl Pts',(-0.624232678490992,0.42746186663542,
1.48393456654444));
#59364=CARTESIAN_POINT('Ctrl Pts',(-0.650747220896674,0.922840472525375,
1.23809285168862));
#59365=CARTESIAN_POINT('Ctrl Pts',(-0.677261763302362,1.20109540462185,
0.840373701153215));
#59366=CARTESIAN_POINT('Ctrl Pts',(-0.703776305708048,1.47935033671831,
0.442654550617832));
#59367=CARTESIAN_POINT('Ctrl Pts',(-0.730290848113738,1.54048159502121,
-0.106942035597157));
#59368=CARTESIAN_POINT('Ctrl Pts',(-0.756805390519424,1.35637172984761,
-0.556039857846719));
#59369=CARTESIAN_POINT('Ctrl Pts',(-0.783319932925108,1.17226186467403,
-1.00513768009626));
#59370=CARTESIAN_POINT('Ctrl Pts',(-0.809834475330794,0.742910876024013,
-1.35373673838046));
#59371=CARTESIAN_POINT('Ctrl Pts',(-0.836349017736478,0.265556504920355,
-1.44167185463886));
#59372=CARTESIAN_POINT('Ctrl Pts',(-0.862863560142165,-0.211797866183358,
-1.52960697089727));
#59373=CARTESIAN_POINT('Ctrl Pts',(-0.889378102547852,-0.737155619740722,
-1.35687814512982));
#59374=CARTESIAN_POINT('Ctrl Pts',(-0.91589264495354,-1.06920938330862,
-1.00284754652629));
#59375=CARTESIAN_POINT('Ctrl Pts',(-0.935876748021415,-1.31947946278746,
-0.736013449847445));
#59376=CARTESIAN_POINT('Ctrl Pts',(-0.95586085108929,-1.45993954834883,
-0.366187446103257));
#59377=CARTESIAN_POINT('Ctrl Pts',(-0.975844954157165,-1.4632995300711,
0.00135195255092181));
#59378=CARTESIAN_POINT('Ctrl Pts',(-1.04715504584289,-1.46287428079508,
0.00132175412439906));
#59379=CARTESIAN_POINT('Ctrl Pts',(-1.02795192628985,-1.45979277099851,
-0.352117170168635));
#59380=CARTESIAN_POINT('Ctrl Pts',(-1.00874880673681,-1.33110732839389,
-0.707567307740881));
#59381=CARTESIAN_POINT('Ctrl Pts',(-0.989545687183776,-1.09826933307926,
-0.970940151577963));
#59382=CARTESIAN_POINT('Ctrl Pts',(-0.963031144778092,-0.776780270670734,
-1.33458994384934));
#59383=CARTESIAN_POINT('Ctrl Pts',(-0.936516602372409,-0.256729902572511,
-1.52269926982669));
#59384=CARTESIAN_POINT('Ctrl Pts',(-0.910002059966724,0.223003927681576,
-1.44885926067856));
#59385=CARTESIAN_POINT('Ctrl Pts',(-0.883487517561038,0.70273775793569,
-1.37501925153043));
#59386=CARTESIAN_POINT('Ctrl Pts',(-0.856972975155351,1.14215505034566,
-1.0392299072568));
#59387=CARTESIAN_POINT('Ctrl Pts',(-0.830458432749665,1.33941008664533,
-0.59573789159776));
#59388=CARTESIAN_POINT('Ctrl Pts',(-0.803943890343978,1.53666512294502,
-0.152245875938697));
#59389=CARTESIAN_POINT('Ctrl Pts',(-0.777429347938291,1.49175790313437,
0.398948811105779));
#59390=CARTESIAN_POINT('Ctrl Pts',(-0.750914805532604,1.22532338885631,
0.8046704059668));
#59391=CARTESIAN_POINT('Ctrl Pts',(-0.724400263126918,0.958888874578265,
1.2103920008278));
#59392=CARTESIAN_POINT('Ctrl Pts',(-0.697885720721231,0.470927065832829,
1.47064050350535));
#59393=CARTESIAN_POINT('Ctrl Pts',(-0.671371178315545,-0.0144355535737682,
1.4658545555427));
#59394=CARTESIAN_POINT('Ctrl Pts',(-0.64485663590986,-0.499798172980338,
1.46106860758005));
#59395=CARTESIAN_POINT('Ctrl Pts',(-0.618342093504176,-0.98256160304807,
1.19124820897721));
#59396=CARTESIAN_POINT('Ctrl Pts',(-0.591827551098492,-1.24094710973327,
0.780368395977307));
#59397=CARTESIAN_POINT('Ctrl Pts',(-0.576936716013292,-1.38605902264452,
0.549614138875445));
#59398=CARTESIAN_POINT('Ctrl Pts',(-0.562045880928091,-1.46040081110129,
0.274368907965358));
#59399=CARTESIAN_POINT('Ctrl Pts',(-0.547155045842891,-1.46121426462895,
-0.000470658046818673));
#59400=CARTESIAN_POINT('Origin',(-35.5608671147362,0.,0.));
#59401=CARTESIAN_POINT('',(-0.310867114736255,-1.17578287613307,-0.000108287608020487));
#59402=CARTESIAN_POINT('',(-0.212132885263923,-1.17696636327651,-4.59991182728825E-5));
#59403=CARTESIAN_POINT('',(-35.5608671147362,-1.17775,1.38253677383905E-12));
#59404=CARTESIAN_POINT('',(-0.2,-0.20806946958181,-1.15922480922725));
#59405=CARTESIAN_POINT('Ctrl Pts',(-0.310867114736255,-1.17578287613307,
-0.000108287608020629));
#59406=CARTESIAN_POINT('Ctrl Pts',(-0.298462423900919,-1.17605004458734,
-0.184351563818547));
#59407=CARTESIAN_POINT('Ctrl Pts',(-0.261506718988835,-1.05473749252561,
-0.732947532879346));
#59408=CARTESIAN_POINT('Ctrl Pts',(-0.224551014076752,-0.563910892482186,
-1.09543997095558));
#59409=CARTESIAN_POINT('Ctrl Pts',(-0.200000000000004,-0.207979487136961,
-1.16121778488277));
#59410=CARTESIAN_POINT('',(-0.2,-1.1640875192389,-0.178872328917063));
#59411=CARTESIAN_POINT('Origin',(-0.2,0.,0.));
#59412=CARTESIAN_POINT('Ctrl Pts',(-0.212132885263923,-1.17696636327651,
-4.59991182729606E-5));
#59413=CARTESIAN_POINT('Ctrl Pts',(-0.208088590175949,-1.17739142535704,
-0.059880676848224));
#59414=CARTESIAN_POINT('Ctrl Pts',(-0.204044295087974,-1.17317818858489,
-0.119710943859588));
#59415=CARTESIAN_POINT('Ctrl Pts',(-0.2,-1.1640875192389,-0.178872328917063));
#59416=CARTESIAN_POINT('Origin',(-35.5608671147362,0.,0.));
#59417=CARTESIAN_POINT('',(-0.81086711473626,-1.17758867204732,0.00108798231488299));
#59418=CARTESIAN_POINT('',(-0.712132885263918,-1.17591055699811,-0.000378761538900874));
#59419=CARTESIAN_POINT('',(-35.5608671147362,-1.17775,1.38253677383905E-12));
#59420=CARTESIAN_POINT('Ctrl Pts',(-0.81086711473626,-1.17758867204732,
0.00108798231488304));
#59421=CARTESIAN_POINT('Ctrl Pts',(-0.790883011668376,-1.17488473048725,
-0.294688940654132));
#59422=CARTESIAN_POINT('Ctrl Pts',(-0.744384366194804,-0.911876732317324,
-0.987178885589815));
#59423=CARTESIAN_POINT('Ctrl Pts',(-0.671371178315547,0.252336971202078,
-1.36995284217421));
#59424=CARTESIAN_POINT('Ctrl Pts',(-0.591827551098487,1.28889616535859,
-0.528348726914579));
#59425=CARTESIAN_POINT('Ctrl Pts',(-0.512283923881428,1.14131022863273,
0.798513000617958));
#59426=CARTESIAN_POINT('Ctrl Pts',(-0.432740296664372,-0.0546559205033708,
1.39203554179653));
#59427=CARTESIAN_POINT('Ctrl Pts',(-0.365601360282643,-1.02192204925182,
0.813214204481599));
#59428=CARTESIAN_POINT('Ctrl Pts',(-0.324976966306605,-1.17547898244608,
0.209461246584642));
#59429=CARTESIAN_POINT('Ctrl Pts',(-0.310867114736255,-1.17578287613307,
-0.000108287608020629));
#59430=CARTESIAN_POINT('Ctrl Pts',(-0.712132885263918,-1.17591055699811,
-0.000378761538900839));
#59431=CARTESIAN_POINT('Ctrl Pts',(-0.700509177943399,-1.17642155446286,
-0.173028232716761));
#59432=CARTESIAN_POINT('Ctrl Pts',(-0.662370928217192,-1.05979880462431,
-0.738851338425022));
#59433=CARTESIAN_POINT('Ctrl Pts',(-0.597718136085294,-0.184831240778329,
-1.38079239774389));
#59434=CARTESIAN_POINT('Ctrl Pts',(-0.518174508868238,1.06175884240671,
-0.901671642965467));
#59435=CARTESIAN_POINT('Ctrl Pts',(-0.438630881651178,1.33236304935347,
0.405021101276792));
#59436=CARTESIAN_POINT('Ctrl Pts',(-0.35908725443412,0.380047119706207,
1.34111457344272));
#59437=CARTESIAN_POINT('Ctrl Pts',(-0.283587922305033,-0.857321546120441,
1.05741628964119));
#59438=CARTESIAN_POINT('Ctrl Pts',(-0.234603132581635,-1.17460470324253,
0.332397597978653));
#59439=CARTESIAN_POINT('Ctrl Pts',(-0.212132885263923,-1.17696636327651,
-4.59991182729606E-5));
#59440=CARTESIAN_POINT('Origin',(-35.5608671147362,0.,0.));
#59441=CARTESIAN_POINT('',(-1.31086711473626,-1.17961310217458,-0.000287142740902327));
#59442=CARTESIAN_POINT('',(-1.21213288526391,-1.17724645316462,0.00106368016567451));
#59443=CARTESIAN_POINT('',(-35.5608671147362,-1.17775,1.38253677383905E-12));
#59444=CARTESIAN_POINT('Ctrl Pts',(-1.31086711473626,-1.17961310217458,
-0.000287142740902635));
#59445=CARTESIAN_POINT('Ctrl Pts',(-1.30981814184151,-1.17966365508524,
-0.0157435394407337));
#59446=CARTESIAN_POINT('Ctrl Pts',(-1.28225462654108,-1.17237480984895,
-0.421837399635015));
#59447=CARTESIAN_POINT('Ctrl Pts',(-1.22817656883496,-0.70621222470226,
-1.20069203698611));
#59448=CARTESIAN_POINT('Ctrl Pts',(-1.14863294161791,0.628250636330202,
-1.24326168777629));
#59449=CARTESIAN_POINT('Ctrl Pts',(-1.06908931440084,1.38555307485394,-0.143670610859339));
#59450=CARTESIAN_POINT('Ctrl Pts',(-0.989545687183782,0.869974654993682,
1.08790505669946));
#59451=CARTESIAN_POINT('Ctrl Pts',(-0.910002059966723,-0.444829315197323,
1.32004950107908));
#59452=CARTESIAN_POINT('Ctrl Pts',(-0.85044253581755,-1.12332549722415,
0.585834040613157));
#59453=CARTESIAN_POINT('Ctrl Pts',(-0.817397554074062,-1.17847227068925,
0.0977424704552608));
#59454=CARTESIAN_POINT('Ctrl Pts',(-0.81086711473626,-1.17758867204732,
0.00108798231488304));
#59455=CARTESIAN_POINT('Ctrl Pts',(-1.21213288526391,-1.17724645316462,
0.00106368016567453));
#59456=CARTESIAN_POINT('Ctrl Pts',(-1.19292976571085,-1.17476661157779,
-0.283365901718006));
#59457=CARTESIAN_POINT('Ctrl Pts',(-1.14721210375209,-0.928218299771867,
-0.964372467620693));
#59458=CARTESIAN_POINT('Ctrl Pts',(-1.07497989938766,0.211906852253127,
-1.3767713178738));
#59459=CARTESIAN_POINT('Ctrl Pts',(-0.995436272170595,1.27276858673064,
-0.566093011994411));
#59460=CARTESIAN_POINT('Ctrl Pts',(-0.915892644953538,1.16435148089155,
0.76462692514249));
#59461=CARTESIAN_POINT('Ctrl Pts',(-0.836349017736476,-0.0137086904440423,
1.39293100582981));
#59462=CARTESIAN_POINT('Ctrl Pts',(-0.768429097839939,-1.00890275949954,
0.836708964814963));
#59463=CARTESIAN_POINT('Ctrl Pts',(-0.727023720349086,-1.17525593117465,
0.220798074040274));
#59464=CARTESIAN_POINT('Ctrl Pts',(-0.712132885263918,-1.17591055699811,
-0.000378761538900839));
#59465=CARTESIAN_POINT('Origin',(-35.5608671147362,0.,0.));
#59466=CARTESIAN_POINT('',(-1.81086711473626,-1.17671872564126,-0.000945352728389693));
#59467=CARTESIAN_POINT('',(-1.71213288526391,-1.17969178884661,-7.43461005511814E-5));
#59468=CARTESIAN_POINT('',(-35.5608671147362,-1.17775,1.38253677383905E-12));
#59469=CARTESIAN_POINT('Ctrl Pts',(-1.81086711473626,-1.17671872564126,
-0.000945352728389855));
#59470=CARTESIAN_POINT('Ctrl Pts',(-1.80223872960897,-1.17767741781437,
-0.128890916571168));
#59471=CARTESIAN_POINT('Ctrl Pts',(-1.76709580207599,-1.09939444640547,
-0.648864838733412));
#59472=CARTESIAN_POINT('Ctrl Pts',(-1.70543833213732,-0.339145526056245,
-1.35106551741206));
#59473=CARTESIAN_POINT('Ctrl Pts',(-1.62589470492026,0.9532093987185,-1.01577043941121));
#59474=CARTESIAN_POINT('Ctrl Pts',(-1.5463510777032,1.36987018532208,0.25269238205091));
#59475=CARTESIAN_POINT('Ctrl Pts',(-1.46680745048614,0.528058971205146,
1.28901177668085));
#59476=CARTESIAN_POINT('Ctrl Pts',(-1.38831279616383,-0.78137054082941,
1.14309230194811));
#59477=CARTESIAN_POINT('Ctrl Pts',(-1.3363326842472,-1.17838584581094,0.374942709736548));
#59478=CARTESIAN_POINT('Ctrl Pts',(-1.31086711473626,-1.17961310217458,
-0.000287142740902635));
#59479=CARTESIAN_POINT('Ctrl Pts',(-1.71213288526391,-1.17969178884661,
-7.43461005513196E-5));
#59480=CARTESIAN_POINT('Ctrl Pts',(-1.71186489588399,-1.17969537820321,
-0.00402240689185183));
#59481=CARTESIAN_POINT('Ctrl Pts',(-1.68508236409837,-1.17788662184485,
-0.398583404005852));
#59482=CARTESIAN_POINT('Ctrl Pts',(-1.63178528990707,-0.74125237059894,
-1.17938226616436));
#59483=CARTESIAN_POINT('Ctrl Pts',(-1.55224166269001,0.591379222800219,
-1.26121703368907));
#59484=CARTESIAN_POINT('Ctrl Pts',(-1.47269803547295,1.3807228481852,-0.18439709057274));
#59485=CARTESIAN_POINT('Ctrl Pts',(-1.3931544082559,0.901624120319131,1.06182436804775));
#59486=CARTESIAN_POINT('Ctrl Pts',(-1.31361078103883,-0.405777918272958,
1.33256997446379));
#59487=CARTESIAN_POINT('Ctrl Pts',(-1.25327027337484,-1.11476781233784,
0.609290130836548));
#59488=CARTESIAN_POINT('Ctrl Pts',(-1.21944430811653,-1.17819063155183,
0.109357800774495));
#59489=CARTESIAN_POINT('Ctrl Pts',(-1.21213288526391,-1.17724645316462,
0.00106368016567453));
#59490=CARTESIAN_POINT('Origin',(-35.5608671147362,0.,0.));
#59491=CARTESIAN_POINT('',(-2.31086711473625,-1.17618874332304,0.000674505468416633));
#59492=CARTESIAN_POINT('',(-2.21213288526391,-1.1770225168604,-0.00102674357284102));
#59493=CARTESIAN_POINT('',(-35.5608671147362,-1.17775,1.38253677383905E-12));
#59494=CARTESIAN_POINT('Ctrl Pts',(-2.31086711473625,-1.17618874332304,
0.000674505468416693));
#59495=CARTESIAN_POINT('Ctrl Pts',(-2.29465931737641,-1.17493999723399,
-0.239934057218548));
#59496=CARTESIAN_POINT('Ctrl Pts',(-2.25193697761089,-0.985923408261569,
-0.875958445349159));
#59497=CARTESIAN_POINT('Ctrl Pts',(-2.18270009543968,0.0554231623812737,
-1.39187858910792));
#59498=CARTESIAN_POINT('Ctrl Pts',(-2.10315646822262,1.2008705947473,-0.7059090229788));
#59499=CARTESIAN_POINT('Ctrl Pts',(-2.02361284100557,1.24310255349976,0.628564854542996));
#59500=CARTESIAN_POINT('Ctrl Pts',(-1.9440692137885,0.143321393236571,1.38558893987825));
#59501=CARTESIAN_POINT('Ctrl Pts',(-1.87315397169873,-0.954546644775816,
0.925660834446937));
#59502=CARTESIAN_POINT('Ctrl Pts',(-1.82875327201465,-1.17473141066438,
0.264278607978505));
#59503=CARTESIAN_POINT('Ctrl Pts',(-1.81086711473626,-1.17671872564126,
-0.000945352728389855));
#59504=CARTESIAN_POINT('Ctrl Pts',(-2.21213288526391,-1.1770225168604,-0.00102674357284116));
#59505=CARTESIAN_POINT('Ctrl Pts',(-2.20428548365143,-1.17798678341153,
-0.117315720736906));
#59506=CARTESIAN_POINT('Ctrl Pts',(-2.16992353963328,-1.1086556584985,-0.625393540296511));
#59507=CARTESIAN_POINT('Ctrl Pts',(-2.10904705320943,-0.378771384950898,
-1.34049615412855));
#59508=CARTESIAN_POINT('Ctrl Pts',(-2.02950342599237,0.922893894627693,
-1.04339089670334));
#59509=CARTESIAN_POINT('Ctrl Pts',(-1.94995979877531,1.37671526305346,0.21225643214144));
#59510=CARTESIAN_POINT('Ctrl Pts',(-1.87041617155825,0.56577621956083,1.2729080716121));
#59511=CARTESIAN_POINT('Ctrl Pts',(-1.79114053372112,-0.76044669356272,
1.1645312469487));
#59512=CARTESIAN_POINT('Ctrl Pts',(-1.73837943828967,-1.17934025163867,
0.386593912679761));
#59513=CARTESIAN_POINT('Ctrl Pts',(-1.71213288526391,-1.17969178884661,
-7.43461005513196E-5));
#59514=CARTESIAN_POINT('Origin',(-35.5608671147362,0.,0.));
#59515=CARTESIAN_POINT('',(-2.81086711473625,-1.1791908097051,0.000690623389146067));
#59516=CARTESIAN_POINT('',(-2.71213288526391,-1.1760125816614,0.000513121278469739));
#59517=CARTESIAN_POINT('',(-35.5608671147362,-1.17775,1.38253677383905E-12));
#59518=CARTESIAN_POINT('Ctrl Pts',(-2.81086711473625,-1.1791908097051,0.000690623389146068));
#59519=CARTESIAN_POINT('Ctrl Pts',(-2.78707990514387,-1.17675200961973,
-0.350141529500257));
#59520=CARTESIAN_POINT('Ctrl Pts',(-2.7367781531458,-0.824340564457964,
-1.09628254632819));
#59521=CARTESIAN_POINT('Ctrl Pts',(-2.65996185874204,0.445497494323327,
-1.31982185031089));
#59522=CARTESIAN_POINT('Ctrl Pts',(-2.58041823152498,1.35115114421937,-0.338804249505638));
#59523=CARTESIAN_POINT('Ctrl Pts',(-2.50087460430792,1.01552962555056,0.953465947825067));
#59524=CARTESIAN_POINT('Ctrl Pts',(-2.42133097709085,-0.253038375497675,
1.36980630546842));
#59525=CARTESIAN_POINT('Ctrl Pts',(-2.35799514723364,-1.07802819152289,
0.699314027852116));
#59526=CARTESIAN_POINT('Ctrl Pts',(-2.3211738597821,-1.17698283688684,0.153680559061323));
#59527=CARTESIAN_POINT('Ctrl Pts',(-2.31086711473625,-1.17618874332304,
0.000674505468416693));
#59528=CARTESIAN_POINT('Ctrl Pts',(-2.71213288526391,-1.1760125816614,0.000513121278469617));
#59529=CARTESIAN_POINT('Ctrl Pts',(-2.69670607141889,-1.17511628475514,
-0.228587358038304));
#59530=CARTESIAN_POINT('Ctrl Pts',(-2.65476471516818,-0.999712830335691,
-0.852717840732116));
#59531=CARTESIAN_POINT('Ctrl Pts',(-2.58630881651179,0.0144248373372911,
-1.3929068982755));
#59532=CARTESIAN_POINT('Ctrl Pts',(-2.50676518929473,1.17956949077493,-0.740954465306795));
#59533=CARTESIAN_POINT('Ctrl Pts',(-2.42722156207767,1.26106756278956,0.591697815993344));
#59534=CARTESIAN_POINT('Ctrl Pts',(-2.34767793486061,0.184048426393107,
1.38076930720073));
#59535=CARTESIAN_POINT('Ctrl Pts',(-2.27598170925602,-0.939117811692954,
0.948652692700248));
#59536=CARTESIAN_POINT('Ctrl Pts',(-2.23080002605712,-1.17472875131086,
0.275597649649284));
#59537=CARTESIAN_POINT('Ctrl Pts',(-2.21213288526391,-1.1770225168604,-0.00102674357284116));
#59538=CARTESIAN_POINT('Origin',(-35.5608671147362,0.,0.));
#59539=CARTESIAN_POINT('',(-3.31086711473625,-1.17834427569628,-0.00101628109532418));
#59540=CARTESIAN_POINT('',(-3.21213288526392,-1.17890781883051,0.000838500381393336));
#59541=CARTESIAN_POINT('',(-35.5608671147362,-1.17775,1.38253677383905E-12));
#59542=CARTESIAN_POINT('Ctrl Pts',(-3.31086711473625,-1.17834427569628,
-0.00101628109532408));
#59543=CARTESIAN_POINT('Ctrl Pts',(-3.30601503531701,-1.17899808071603,
-0.072712416598091));
#59544=CARTESIAN_POINT('Ctrl Pts',(-3.27464841349208,-1.14034568634848,
-0.535493912102965));
#59545=CARTESIAN_POINT('Ctrl Pts',(-3.21676724926146,-0.527407731806677,
-1.28927840998041));
#59546=CARTESIAN_POINT('Ctrl Pts',(-3.13722362204439,0.799445675505238,
-1.14073850900496));
#59547=CARTESIAN_POINT('Ctrl Pts',(-3.05767999482733,1.39186454536937,0.0557747376017607));
#59548=CARTESIAN_POINT('Ctrl Pts',(-2.97813636761027,0.705605670279753,
1.20104886331929));
#59549=CARTESIAN_POINT('Ctrl Pts',(-2.89859274039321,-0.62887883157946,
1.24294374337767));
#59550=CARTESIAN_POINT('Ctrl Pts',(-2.84283632276854,-1.15932309657661,
0.47191381349839));
#59551=CARTESIAN_POINT('Ctrl Pts',(-2.81359444754955,-1.17947043138465,
0.0409154357539586));
#59552=CARTESIAN_POINT('Ctrl Pts',(-2.81086711473625,-1.1791908097051,0.000690623389146068));
#59553=CARTESIAN_POINT('Ctrl Pts',(-3.21213288526392,-1.17890781883051,
0.000838500381393362));
#59554=CARTESIAN_POINT('Ctrl Pts',(-3.18912665918635,-1.17617355211756,
-0.338688512228519));
#59555=CARTESIAN_POINT('Ctrl Pts',(-3.13960589070309,-0.843417985641057,
-1.07419213998031));
#59556=CARTESIAN_POINT('Ctrl Pts',(-3.06357057981415,0.406451325412254,
-1.33236444837786));
#59557=CARTESIAN_POINT('Ctrl Pts',(-2.98402695259708,1.34059178648789,-0.378432775049564));
#59558=CARTESIAN_POINT('Ctrl Pts',(-2.90448332538003,1.04315774690456,0.923157417945318));
#59559=CARTESIAN_POINT('Ctrl Pts',(-2.82493969816297,-0.212604170117943,
1.37666160332707));
#59560=CARTESIAN_POINT('Ctrl Pts',(-2.76082288479093,-1.06738626099137,
0.722781401633066));
#59561=CARTESIAN_POINT('Ctrl Pts',(-2.72322061382458,-1.17665677798775,
0.165174726280128));
#59562=CARTESIAN_POINT('Ctrl Pts',(-2.71213288526391,-1.1760125816614,0.000513121278469617));
#59563=CARTESIAN_POINT('Origin',(-35.5608671147362,0.,0.));
#59564=CARTESIAN_POINT('',(-3.81086711473625,-1.17583062577477,-0.000201975373600133));
#59565=CARTESIAN_POINT('',(-3.71213288526391,-1.17868089293979,-0.000925409118186643));
#59566=CARTESIAN_POINT('',(-35.5608671147362,-1.17775,1.38253677383905E-12));
#59567=CARTESIAN_POINT('Ctrl Pts',(-3.81086711473625,-1.17583062577477,
-0.000201975373600293));
#59568=CARTESIAN_POINT('Ctrl Pts',(-3.79843562308445,-1.17611245328021,
-0.184890850251831));
#59569=CARTESIAN_POINT('Ctrl Pts',(-3.75948958902697,-1.04800296746839,
-0.763124087068342));
#59570=CARTESIAN_POINT('Ctrl Pts',(-3.69402901256381,-0.142621398653279,
-1.3856611673339));
#59571=CARTESIAN_POINT('Ctrl Pts',(-3.61448538534675,1.08856544484988,-0.869150738531468));
#59572=CARTESIAN_POINT('Ctrl Pts',(-3.53494175812969,1.31970927922097,0.445830856210143));
#59573=CARTESIAN_POINT('Ctrl Pts',(-3.45539813091263,0.338462949072693,
1.35123668027329));
#59574=CARTESIAN_POINT('Ctrl Pts',(-3.38070658311482,-0.874900453070544,
1.03578123328469));
#59575=CARTESIAN_POINT('Ctrl Pts',(-3.33252957772269,-1.17542531542853,
0.319076352887373));
#59576=CARTESIAN_POINT('Ctrl Pts',(-3.31086711473625,-1.17834427569628,
-0.00101628109532408));
#59577=CARTESIAN_POINT('Ctrl Pts',(-3.71213288526391,-1.17868089293979,
-0.000925409118186669));
#59578=CARTESIAN_POINT('Ctrl Pts',(-3.70806178935948,-1.17919921175325,
-0.0610369679214061));
#59579=CARTESIAN_POINT('Ctrl Pts',(-3.67747615104936,-1.14764809049271,
-0.512101957958643));
#59580=CARTESIAN_POINT('Ctrl Pts',(-3.62037597033357,-0.565133098256669,
-1.27319373407426));
#59581=CARTESIAN_POINT('Ctrl Pts',(-3.5408323431165,0.765517983049464,-1.16377829540639));
#59582=CARTESIAN_POINT('Ctrl Pts',(-3.46128871589945,1.39290321025801,0.0147766736470439));
#59583=CARTESIAN_POINT('Ctrl Pts',(-3.38174508868238,0.740656492133029,
1.17975661214186));
#59584=CARTESIAN_POINT('Ctrl Pts',(-3.30220146146532,-0.592016332323219,
1.2609180645441));
#59585=CARTESIAN_POINT('Ctrl Pts',(-3.24566406032584,-1.15267305353486,
0.495261131766334));
#59586=CARTESIAN_POINT('Ctrl Pts',(-3.21564120159203,-1.17932477867964,
0.0526144047891755));
#59587=CARTESIAN_POINT('Ctrl Pts',(-3.21213288526392,-1.17890781883051,
0.000838500381393362));
#59588=CARTESIAN_POINT('Origin',(-35.5608671147362,0.,0.));
#59589=CARTESIAN_POINT('',(-4.31086711473625,-1.17760067476461,0.00108813158859299));
#59590=CARTESIAN_POINT('',(-4.21213288526391,-1.17591708598406,-0.000386845562409671));
#59591=CARTESIAN_POINT('',(-35.5608671147362,-1.17775,1.38253677383905E-12));
#59592=CARTESIAN_POINT('Ctrl Pts',(-4.31086711473625,-1.17760067476461,
0.00108813158859295));
#59593=CARTESIAN_POINT('Ctrl Pts',(-4.29085621085191,-1.1748911418629,-0.295079604829545));
#59594=CARTESIAN_POINT('Ctrl Pts',(-4.24433076456189,-0.911310100265462,
-0.987967233608653));
#59595=CARTESIAN_POINT('Ctrl Pts',(-4.17129077586617,0.253730346700255,
-1.36967829988445));
#59596=CARTESIAN_POINT('Ctrl Pts',(-4.09174714864911,1.28941158768824,-0.527082053902699));
#59597=CARTESIAN_POINT('Ctrl Pts',(-4.01220352143205,1.14053653923849,0.799733791128557));
#59598=CARTESIAN_POINT('Ctrl Pts',(-3.93265989421499,-0.0561263093121601,
1.39185041272904));
#59599=CARTESIAN_POINT('Ctrl Pts',(-3.86554775864972,-1.02226475660902,
0.812599585797225));
#59600=CARTESIAN_POINT('Ctrl Pts',(-3.82495016549014,-1.17551135668189,
0.209023342990697));
#59601=CARTESIAN_POINT('Ctrl Pts',(-3.81086711473625,-1.17583062577477,
-0.000201975373600293));
#59602=CARTESIAN_POINT('Ctrl Pts',(-4.21213288526391,-1.17591708598406,
-0.000386845562409758));
#59603=CARTESIAN_POINT('Ctrl Pts',(-4.20048237712693,-1.17642504647458,
-0.173441263805405));
#59604=CARTESIAN_POINT('Ctrl Pts',(-4.16231732658427,-1.05943529231218,
-0.739684098294869));
#59605=CARTESIAN_POINT('Ctrl Pts',(-4.09763773363592,-0.183350861145989,
-1.38086210931729));
#59606=CARTESIAN_POINT('Ctrl Pts',(-4.01809410641886,1.06250748323233,-0.900819377736997));
#59607=CARTESIAN_POINT('Ctrl Pts',(-3.9385504792018,1.3322617396258,0.406787856702201));
#59608=CARTESIAN_POINT('Ctrl Pts',(-3.85900685198474,0.378094140562434,
1.34068733271538));
#59609=CARTESIAN_POINT('Ctrl Pts',(-3.78353432067212,-0.856808474456836,
1.05816423047969));
#59610=CARTESIAN_POINT('Ctrl Pts',(-3.73457633176517,-1.17582346564415,
0.330462154765891));
#59611=CARTESIAN_POINT('Ctrl Pts',(-3.71213288526391,-1.17868089293979,
-0.000925409118186669));
#59612=CARTESIAN_POINT('Origin',(-35.5608671147362,0.,0.));
#59613=CARTESIAN_POINT('',(-4.81086711473624,-1.17960887409498,-0.000294231637304944));
#59614=CARTESIAN_POINT('',(-4.71213288526391,-1.17725794698973,0.0010650668865906));
#59615=CARTESIAN_POINT('',(-35.5608671147362,-1.17775,1.38253677383905E-12));
#59616=CARTESIAN_POINT('Ctrl Pts',(-4.81086711473624,-1.17960887409498,
-0.000294231637304968));
#59617=CARTESIAN_POINT('Ctrl Pts',(-4.80979134102505,-1.17966188515311,
-0.0161456849046697));
#59618=CARTESIAN_POINT('Ctrl Pts',(-4.78220102490816,-1.17217941461582,
-0.422635941839761));
#59619=CARTESIAN_POINT('Ctrl Pts',(-4.72809616638559,-0.704998830211815,
-1.20140517037799));
#59620=CARTESIAN_POINT('Ctrl Pts',(-4.64855253916853,0.629506665960787,
-1.24262588558339));
#59621=CARTESIAN_POINT('Ctrl Pts',(-4.56900891195147,1.38569714811699,-0.142271387535955));
#59622=CARTESIAN_POINT('Ctrl Pts',(-4.48946528473441,0.868875748162881,
1.08878495042198));
#59623=CARTESIAN_POINT('Ctrl Pts',(-4.40992165751735,-0.446164189652799,
1.31959662392811));
#59624=CARTESIAN_POINT('Ctrl Pts',(-4.35038893418463,-1.12361025449941,
0.585032693523647));
#59625=CARTESIAN_POINT('Ctrl Pts',(-4.3173707532576,-1.1784812857883,0.0973440483868324));
#59626=CARTESIAN_POINT('Ctrl Pts',(-4.31086711473625,-1.17760067476461,
0.00108813158859295));
#59627=CARTESIAN_POINT('Ctrl Pts',(-4.71213288526391,-1.17725794698973,
0.00106506688659067));
#59628=CARTESIAN_POINT('Ctrl Pts',(-4.69290296489438,-1.17476961504499,
-0.283754674824574));
#59629=CARTESIAN_POINT('Ctrl Pts',(-4.64715850211917,-0.927667344013,-0.965158191565359));
#59630=CARTESIAN_POINT('Ctrl Pts',(-4.57489949693828,0.213299609668962,
-1.37655402354802));
#59631=CARTESIAN_POINT('Ctrl Pts',(-4.49535586972123,1.27333644141125,-0.564811482005513));
#59632=CARTESIAN_POINT('Ctrl Pts',(-4.41581224250416,1.1635848947598,0.765811919414912));
#59633=CARTESIAN_POINT('Ctrl Pts',(-4.33626861528711,-0.0151285090234098,
1.39289943335687));
#59634=CARTESIAN_POINT('Ctrl Pts',(-4.26837549620702,-1.0093367994606,0.835934120578));
#59635=CARTESIAN_POINT('Ctrl Pts',(-4.22699691953262,-1.17526901621324,
0.220400674850707));
#59636=CARTESIAN_POINT('Ctrl Pts',(-4.21213288526391,-1.17591708598406,
-0.000386845562409758));
#59637=CARTESIAN_POINT('Origin',(-35.5608671147362,0.,0.));
#59638=CARTESIAN_POINT('',(-5.31086711473625,-1.17670885667242,-0.000942008607549203));
#59639=CARTESIAN_POINT('',(-5.21213288526391,-1.17969057793969,-8.17602703367948E-5));
#59640=CARTESIAN_POINT('',(-35.5608671147362,-1.17775,1.38253677383905E-12));
#59641=CARTESIAN_POINT('Ctrl Pts',(-5.31086711473625,-1.17670885667242,
-0.00094200860754937));
#59642=CARTESIAN_POINT('Ctrl Pts',(-5.3022119287925,-1.1776665848779,-0.129287698859234));
#59643=CARTESIAN_POINT('Ctrl Pts',(-5.26704220044306,-1.09906906098629,
-0.64967040496034));
#59644=CARTESIAN_POINT('Ctrl Pts',(-5.20535792968794,-0.337780283452094,
-1.35140749373458));
#59645=CARTESIAN_POINT('Ctrl Pts',(-5.12581430247089,0.954235217191234,
-1.01480682116499));
#59646=CARTESIAN_POINT('Ctrl Pts',(-5.04627067525382,1.36961416599977,0.254076308033152));
#59647=CARTESIAN_POINT('Ctrl Pts',(-4.96672704803676,0.526756342369506,
1.2895446831283));
#59648=CARTESIAN_POINT('Ctrl Pts',(-4.88825919453091,-0.782078078757634,
1.14235246346663));
#59649=CARTESIAN_POINT('Ctrl Pts',(-4.83630588343073,-1.17835532417835,
0.374544313813887));
#59650=CARTESIAN_POINT('Ctrl Pts',(-4.81086711473624,-1.17960887409498,
-0.000294231637304968));
#59651=CARTESIAN_POINT('Ctrl Pts',(-5.21213288526391,-1.17969057793969,
-8.17602703368457E-5));
#59652=CARTESIAN_POINT('Ctrl Pts',(-5.21183809506752,-1.17969490898888,
-0.0044246668410752));
#59653=CARTESIAN_POINT('Ctrl Pts',(-5.18502876246545,-1.17770326595971,
-0.399380889169589));
#59654=CARTESIAN_POINT('Ctrl Pts',(-5.13170488745769,-0.740060404085762,
-1.1801306290134));
#59655=CARTESIAN_POINT('Ctrl Pts',(-5.05216126024064,0.592653251738383,
-1.26061882678114));
#59656=CARTESIAN_POINT('Ctrl Pts',(-4.97261763302358,1.38090837817934,-0.183002060931766));
#59657=CARTESIAN_POINT('Ctrl Pts',(-4.89307400580652,0.900550968384048,
1.06273498887245));
#59658=CARTESIAN_POINT('Ctrl Pts',(-4.81353037858945,-0.407124362038215,
1.33215894587174));
#59659=CARTESIAN_POINT('Ctrl Pts',(-4.75321667174192,-1.1150679509245,0.608485500857434));
#59660=CARTESIAN_POINT('Ctrl Pts',(-4.71941750730007,-1.17820056959916,
0.108959646111801));
#59661=CARTESIAN_POINT('Ctrl Pts',(-4.71213288526391,-1.17725794698973,
0.00106506688659067));
#59662=CARTESIAN_POINT('Origin',(-35.5608671147362,0.,0.));
#59663=CARTESIAN_POINT('',(-5.81086711473624,-1.17619564711525,0.000679704233106716));
#59664=CARTESIAN_POINT('',(-5.71213288526391,-1.17701161509376,-0.0010244818722574));
#59665=CARTESIAN_POINT('',(-35.5608671147362,-1.17775,1.38253677383905E-12));
#59666=CARTESIAN_POINT('Ctrl Pts',(-5.81086711473624,-1.17619564711525,
0.000679704233106926));
#59667=CARTESIAN_POINT('Ctrl Pts',(-5.79463251655995,-1.17493475376919,
-0.240323181193375));
#59668=CARTESIAN_POINT('Ctrl Pts',(-5.75188337597797,-0.985441160761987,
-0.876754842997505));
#59669=CARTESIAN_POINT('Ctrl Pts',(-5.68261969299031,0.0568294419673366,
-1.39182188103819));
#59670=CARTESIAN_POINT('Ctrl Pts',(-5.60307606577323,1.20158320893396,-0.704695342697066));
#59671=CARTESIAN_POINT('Ctrl Pts',(-5.52353243855619,1.24246683775691,0.629820522915297));
#59672=CARTESIAN_POINT('Ctrl Pts',(-5.44398881133912,0.141921367341324,
1.38573304048903));
#59673=CARTESIAN_POINT('Ctrl Pts',(-5.37310037006582,-0.955066676424592,
0.924870157254964));
#59674=CARTESIAN_POINT('Ctrl Pts',(-5.32872647119819,-1.17473265309615,
0.26389013335399));
#59675=CARTESIAN_POINT('Ctrl Pts',(-5.31086711473625,-1.17670885667242,
-0.00094200860754937));
#59676=CARTESIAN_POINT('Ctrl Pts',(-5.71213288526391,-1.17701161509376,
-0.00102448187225759));
#59677=CARTESIAN_POINT('Ctrl Pts',(-5.70425868283498,-1.17797639299272,
-0.11771334838427));
#59678=CARTESIAN_POINT('Ctrl Pts',(-5.66986993800036,-1.10834486446487,
-0.626198871419997));
#59679=CARTESIAN_POINT('Ctrl Pts',(-5.60896665076006,-0.377416799240644,
-1.34087816854557));
#59680=CARTESIAN_POINT('Ctrl Pts',(-5.52942302354299,0.923947631924043,
-1.0424579016407));
#59681=CARTESIAN_POINT('Ctrl Pts',(-5.44987939632593,1.37650010191426,0.213647309042655));
#59682=CARTESIAN_POINT('Ctrl Pts',(-5.37033576910888,0.564489829717927,
1.27347906750608));
#59683=CARTESIAN_POINT('Ctrl Pts',(-5.2910869320882,-0.761174594165626,
1.16379940679085));
#59684=CARTESIAN_POINT('Ctrl Pts',(-5.23835263747321,-1.17930535808438,
0.386192734438204));
#59685=CARTESIAN_POINT('Ctrl Pts',(-5.21213288526391,-1.17969057793969,
-8.17602703368457E-5));
#59686=CARTESIAN_POINT('Origin',(-35.5608671147362,0.,0.));
#59687=CARTESIAN_POINT('',(-6.31086711473623,-1.17919972158703,0.000685029099866681));
#59688=CARTESIAN_POINT('',(-6.2121328852639,-1.17601780156144,0.000518948208354519));
#59689=CARTESIAN_POINT('',(-35.5608671147362,-1.17775,1.38253677383905E-12));
#59690=CARTESIAN_POINT('Ctrl Pts',(-6.31086711473623,-1.17919972158703,
0.000685029099866626));
#59691=CARTESIAN_POINT('Ctrl Pts',(-6.2870531043274,-1.1767738351423,-0.350535422240098));
#59692=CARTESIAN_POINT('Ctrl Pts',(-6.23672455151288,-0.823675614850911,
-1.09703732904515));
#59693=CARTESIAN_POINT('Ctrl Pts',(-6.15988145629266,0.446830771117568,
-1.31937106076852));
#59694=CARTESIAN_POINT('Ctrl Pts',(-6.08033782907561,1.35149277113303,-0.337438918303999));
#59695=CARTESIAN_POINT('Ctrl Pts',(-6.00079420185854,1.01456575685592,0.954491518572258));
#59696=CARTESIAN_POINT('Ctrl Pts',(-5.92125057464148,-0.254422253155312,
1.36954994473014));
#59697=CARTESIAN_POINT('Ctrl Pts',(-5.85794154560071,-1.07838539397748,
0.698508541121604));
#59698=CARTESIAN_POINT('Ctrl Pts',(-5.82114705896563,-1.1769940600563,0.153285650768014));
#59699=CARTESIAN_POINT('Ctrl Pts',(-5.81086711473624,-1.17619564711525,
0.000679704233106926));
#59700=CARTESIAN_POINT('Ctrl Pts',(-6.2121328852639,-1.17601780156144,0.000518948208354537));
#59701=CARTESIAN_POINT('Ctrl Pts',(-6.19667927060242,-1.17510951974459,
-0.22897699947036));
#59702=CARTESIAN_POINT('Ctrl Pts',(-6.15471111353526,-0.999248015551786,
-0.85351639676874));
#59703=CARTESIAN_POINT('Ctrl Pts',(-6.08622841406241,0.0158321768580185,
-1.39289161294304));
#59704=CARTESIAN_POINT('Ctrl Pts',(-6.00668478684535,1.18031752451205,-0.739762289225985));
#59705=CARTESIAN_POINT('Ctrl Pts',(-5.92714115962829,1.26046908724875,0.592971654736946));
#59706=CARTESIAN_POINT('Ctrl Pts',(-5.84759753241124,0.182653249041503,
1.38095455893587));
#59707=CARTESIAN_POINT('Ctrl Pts',(-5.77592810762311,-0.939656131499914,
0.947865308820643));
#59708=CARTESIAN_POINT('Ctrl Pts',(-5.73077322524066,-1.17472772816033,
0.275209227245314));
#59709=CARTESIAN_POINT('Ctrl Pts',(-5.71213288526391,-1.17701161509376,
-0.00102448187225759));
#59710=CARTESIAN_POINT('Origin',(-35.5608671147362,0.,0.));
#59711=CARTESIAN_POINT('',(-6.81086711473623,-1.17833240675485,-0.00101876322115038));
#59712=CARTESIAN_POINT('',(-6.7121328852639,-1.17891820058549,0.000833935244456217));
#59713=CARTESIAN_POINT('',(-35.5608671147362,-1.17775,1.38253677383905E-12));
#59714=CARTESIAN_POINT('Ctrl Pts',(-6.81086711473623,-1.17833240675485,
-0.00101876322115052));
#59715=CARTESIAN_POINT('Ctrl Pts',(-6.80598823450053,-1.17899064958735,
-0.0731127916092454));
#59716=CARTESIAN_POINT('Ctrl Pts',(-6.77459481185915,-1.14008822124925,
-0.536297066982777));
#59717=CARTESIAN_POINT('Ctrl Pts',(-6.71668684681209,-0.526104818498686,
-1.28981062717108));
#59718=CARTESIAN_POINT('Ctrl Pts',(-6.63714321959501,0.800597831774603,
-1.13993019337537));
#59719=CARTESIAN_POINT('Ctrl Pts',(-6.55759959237797,1.39180748198953,0.0571810028673485));
#59720=CARTESIAN_POINT('Ctrl Pts',(-6.47805596516089,0.704391810220957,
1.2017611708258));
#59721=CARTESIAN_POINT('Ctrl Pts',(-6.39851233794385,-0.630134339685656,
1.24230771065784));
#59722=CARTESIAN_POINT('Ctrl Pts',(-6.34278272113561,-1.15954471322248,
0.471113104676609));
#59723=CARTESIAN_POINT('Ctrl Pts',(-6.31356764673308,-1.17947481947488,
0.0405137706896489));
#59724=CARTESIAN_POINT('Ctrl Pts',(-6.31086711473623,-1.17919972158703,
0.000685029099866626));
#59725=CARTESIAN_POINT('Ctrl Pts',(-6.71213288526389,-1.17891820058549,
0.000833935244456199));
#59726=CARTESIAN_POINT('Ctrl Pts',(-6.68909985836987,-1.1761915925298,-0.339080789692708));
#59727=CARTESIAN_POINT('Ctrl Pts',(-6.63955228907016,-0.842772870908722,
-1.07495319818965));
#59728=CARTESIAN_POINT('Ctrl Pts',(-6.56349017736478,0.407797294762003,
-1.33195310338462));
#59729=CARTESIAN_POINT('Ctrl Pts',(-6.4839465501477,1.34097345813645,-0.377078092448702));
#59730=CARTESIAN_POINT('Ctrl Pts',(-6.40440292293066,1.04222448684345,0.924210918705832));
#59731=CARTESIAN_POINT('Ctrl Pts',(-6.32485929571359,-0.213994994785076,
1.37644609245625));
#59732=CARTESIAN_POINT('Ctrl Pts',(-6.26076928315801,-1.06775896809028,
0.721976263731495));
#59733=CARTESIAN_POINT('Ctrl Pts',(-6.22319381300811,-1.17666790445113,
0.164780718057665));
#59734=CARTESIAN_POINT('Ctrl Pts',(-6.2121328852639,-1.17601780156144,0.000518948208354537));
#59735=CARTESIAN_POINT('Origin',(-35.5608671147362,0.,0.));
#59736=CARTESIAN_POINT('',(-7.31086711473623,-1.17582863156191,-0.000195490556475402));
#59737=CARTESIAN_POINT('',(-7.2121328852639,-1.17866970590259,-0.0009291108299532));
#59738=CARTESIAN_POINT('',(-35.5608671147362,-1.17775,1.38253677383905E-12));
#59739=CARTESIAN_POINT('Ctrl Pts',(-7.31086711473623,-1.17582863156191,
-0.000195490556475393));
#59740=CARTESIAN_POINT('Ctrl Pts',(-7.29840882226798,-1.17610197282125,
-0.185283315322087));
#59741=CARTESIAN_POINT('Ctrl Pts',(-7.25943598739405,-1.04760233522402,
-0.763928060988009));
#59742=CARTESIAN_POINT('Ctrl Pts',(-7.19394861011444,-0.141221299809534,
-1.38580455999072));
#59743=CARTESIAN_POINT('Ctrl Pts',(-7.11440498289737,1.08944305027853,-0.868050444508131));
#59744=CARTESIAN_POINT('Ctrl Pts',(-7.03486135568032,1.3192581529162,0.447164019097165));
#59745=CARTESIAN_POINT('Ctrl Pts',(-6.95531772846325,0.337097531626415,
1.35157796230272));
#59746=CARTESIAN_POINT('Ctrl Pts',(-6.8806529814819,-0.875511261087105,
1.03501036576305));
#59747=CARTESIAN_POINT('Ctrl Pts',(-6.83250277690622,-1.17541339278816,
0.318686162360974));
#59748=CARTESIAN_POINT('Ctrl Pts',(-6.81086711473623,-1.17833240675485,
-0.00101876322115052));
#59749=CARTESIAN_POINT('Ctrl Pts',(-7.2121328852639,-1.17866970590259,-0.000929110829953382));
#59750=CARTESIAN_POINT('Ctrl Pts',(-7.20803498854302,-1.17919281713394,
-0.0614378874008591));
#59751=CARTESIAN_POINT('Ctrl Pts',(-7.17742254941645,-1.14740386673235,
-0.512904288824735));
#59752=CARTESIAN_POINT('Ctrl Pts',(-7.12029556788419,-0.563846417115518,
-1.27376407593289));
#59753=CARTESIAN_POINT('Ctrl Pts',(-7.04075194066713,0.766693435271625,
-1.16300424743101));
#59754=CARTESIAN_POINT('Ctrl Pts',(-6.96120831345008,1.39288756943087,0.0161840092713161));
#59755=CARTESIAN_POINT('Ctrl Pts',(-6.88166468623301,0.73946412716746,1.1805043447034));
#59756=CARTESIAN_POINT('Ctrl Pts',(-6.80212105901595,-0.593290019902356,
1.26031926729517));
#59757=CARTESIAN_POINT('Ctrl Pts',(-6.74561045869291,-1.15290745544743,
0.494459474393185));
#59758=CARTESIAN_POINT('Ctrl Pts',(-6.71561440077556,-1.1793303360935,0.0522131305606883));
#59759=CARTESIAN_POINT('Ctrl Pts',(-6.71213288526389,-1.17891820058549,
0.000833935244456199));
#59760=CARTESIAN_POINT('Origin',(-35.5608671147362,0.,0.));
#59761=CARTESIAN_POINT('',(-7.81086711473624,-1.17761266659143,0.00108828304854199));
#59762=CARTESIAN_POINT('',(-7.7121328852639,-1.17591322103504,-0.000380663888920052));
#59763=CARTESIAN_POINT('',(-35.5608671147362,-1.17775,1.38253677383905E-12));
#59764=CARTESIAN_POINT('Ctrl Pts',(-7.81086711473624,-1.17761266659143,
0.00108828304854196));
#59765=CARTESIAN_POINT('Ctrl Pts',(-7.79082941003544,-1.17489672111447,
-0.295468412184884));
#59766=CARTESIAN_POINT('Ctrl Pts',(-7.74427716292896,-0.91073905944592,
-0.988747856234089));
#59767=CARTESIAN_POINT('Ctrl Pts',(-7.6712103734168,0.255114094679148,-1.36942124005254));
#59768=CARTESIAN_POINT('Ctrl Pts',(-7.59166674619974,1.28994347575683,-0.525779006202587));
#59769=CARTESIAN_POINT('Ctrl Pts',(-7.51212311898267,1.13972793260945,0.800885743187348));
#59770=CARTESIAN_POINT('Ctrl Pts',(-7.43257949176562,-0.0575325601190364,
1.39179299413997));
#59771=CARTESIAN_POINT('Ctrl Pts',(-7.36549415701681,-1.0226996709703,0.811798018593268));
#59772=CARTESIAN_POINT('Ctrl Pts',(-7.32492336467368,-1.17552023030474,
0.208632543615389));
#59773=CARTESIAN_POINT('Ctrl Pts',(-7.31086711473623,-1.17582863156191,
-0.000195490556475393));
#59774=CARTESIAN_POINT('Ctrl Pts',(-7.7121328852639,-1.17591322103504,-0.00038066388892));
#59775=CARTESIAN_POINT('Ctrl Pts',(-7.70045557631047,-1.17641412149157,
-0.173834599103264));
#59776=CARTESIAN_POINT('Ctrl Pts',(-7.66226372495135,-1.05905068433182,
-0.740488825604028));
#59777=CARTESIAN_POINT('Ctrl Pts',(-7.59755733118654,-0.181955590322025,
-1.38104665612053));
#59778=CARTESIAN_POINT('Ctrl Pts',(-7.51801370396949,1.06341709890332,-0.899745395648787));
#59779=CARTESIAN_POINT('Ctrl Pts',(-7.43847007675242,1.3318500546647,0.408133722106875));
#59780=CARTESIAN_POINT('Ctrl Pts',(-7.35892644953538,0.376739361598168,
1.34106866216976));
#59781=CARTESIAN_POINT('Ctrl Pts',(-7.28348071903918,-0.857438750290286,
1.0573987684494));
#59782=CARTESIAN_POINT('Ctrl Pts',(-7.2345495309487,-1.17580814058615,0.330070886875712));
#59783=CARTESIAN_POINT('Ctrl Pts',(-7.2121328852639,-1.17866970590259,-0.000929110829953382));
#59784=CARTESIAN_POINT('Origin',(-35.5608671147362,0.,0.));
#59785=CARTESIAN_POINT('',(-8.31086711473624,-1.17960456788227,-0.000301336879507475));
#59786=CARTESIAN_POINT('',(-8.21213288526389,-1.17726943853211,0.00106644700324871));
#59787=CARTESIAN_POINT('',(-35.5608671147362,-1.17775,1.38253677383905E-12));
#59788=CARTESIAN_POINT('Ctrl Pts',(-8.31086711473624,-1.17960456788227,
-0.000301336879507583));
#59789=CARTESIAN_POINT('Ctrl Pts',(-8.30976454020858,-1.1796600868532,-0.0165478569140431));
#59790=CARTESIAN_POINT('Ctrl Pts',(-8.28214742327524,-1.17198360631363,
-0.423434528327187));
#59791=CARTESIAN_POINT('Ctrl Pts',(-8.2280157639362,-0.703784610462002,
-1.20211686457176));
#59792=CARTESIAN_POINT('Ctrl Pts',(-8.14847213671916,0.630761852593739,
-1.24198921868246));
#59793=CARTESIAN_POINT('Ctrl Pts',(-8.06892850950209,1.38584018711583,-0.140871252517076));
#59794=CARTESIAN_POINT('Ctrl Pts',(-7.98938488228504,0.867775232498749,
1.08966227789749));
#59795=CARTESIAN_POINT('Ctrl Pts',(-7.90984125506796,-0.447497238546542,
1.31914516089179));
#59796=CARTESIAN_POINT('Ctrl Pts',(-7.85033533255171,-1.12389613593606,
0.584228134995474));
#59797=CARTESIAN_POINT('Ctrl Pts',(-7.81734395244113,-1.17849054848121,
0.0969450497794044));
#59798=CARTESIAN_POINT('Ctrl Pts',(-7.81086711473624,-1.17761266659143,
0.00108828304854196));
#59799=CARTESIAN_POINT('Ctrl Pts',(-8.21213288526389,-1.17726943853211,
0.00106644700324865));
#59800=CARTESIAN_POINT('Ctrl Pts',(-8.19287616407791,-1.17477250782038,
-0.284143183611619));
#59801=CARTESIAN_POINT('Ctrl Pts',(-8.14710490048626,-0.927115044542352,
-0.965942824430619));
#59802=CARTESIAN_POINT('Ctrl Pts',(-8.0748190944889,0.214690325287459,-1.37633781008121));
#59803=CARTESIAN_POINT('Ctrl Pts',(-7.99527546727185,1.27390645824667,-0.563524656841738));
#59804=CARTESIAN_POINT('Ctrl Pts',(-7.91573184005478,1.16281054989956,0.766987176081464));
#59805=CARTESIAN_POINT('Ctrl Pts',(-7.83618821283773,-0.016535840652032,
1.39288343704887));
#59806=CARTESIAN_POINT('Ctrl Pts',(-7.7683218945741,-1.00978864286737,0.835134152043033));
#59807=CARTESIAN_POINT('Ctrl Pts',(-7.72697011871615,-1.17527677499773,
0.220010570106118));
#59808=CARTESIAN_POINT('Ctrl Pts',(-7.7121328852639,-1.17591322103504,-0.00038066388892));
#59809=CARTESIAN_POINT('Origin',(-35.5608671147362,0.,0.));
#59810=CARTESIAN_POINT('',(-8.81086711473623,-1.17669902819161,-0.000938630091047622));
#59811=CARTESIAN_POINT('',(-8.71213288526389,-1.17968925837541,-8.9173716636276E-5));
#59812=CARTESIAN_POINT('',(-35.5608671147362,-1.17775,1.38253677383905E-12));
#59813=CARTESIAN_POINT('Ctrl Pts',(-8.81086711473623,-1.17669902819161,
-0.000938630091047495));
#59814=CARTESIAN_POINT('Ctrl Pts',(-8.80218512797603,-1.17765573995214,
-0.129684452328276));
#59815=CARTESIAN_POINT('Ctrl Pts',(-8.76698859881015,-1.09874317011466,
-0.65047597720531));
#59816=CARTESIAN_POINT('Ctrl Pts',(-8.70527752723856,-0.336414693769986,
-1.35174808593414));
#59817=CARTESIAN_POINT('Ctrl Pts',(-8.62573390002151,0.955260057255724,
-1.01384217559874));
#59818=CARTESIAN_POINT('Ctrl Pts',(-8.54619027280444,1.36935675665274,0.255459991036712));
#59819=CARTESIAN_POINT('Ctrl Pts',(-8.46664664558739,0.525453160360428,
1.29007624204083));
#59820=CARTESIAN_POINT('Ctrl Pts',(-8.38820559289798,-0.782784891184577,
1.14161242002925));
#59821=CARTESIAN_POINT('Ctrl Pts',(-8.33627908261427,-1.1783249751922,0.374145954339654));
#59822=CARTESIAN_POINT('Ctrl Pts',(-8.31086711473624,-1.17960456788227,
-0.000301336879507583));
#59823=CARTESIAN_POINT('Ctrl Pts',(-8.71213288526389,-1.17968925837541,
-8.91737166363286E-5));
#59824=CARTESIAN_POINT('Ctrl Pts',(-8.71181129425105,-1.17969439827978,
-0.00482692941936411));
#59825=CARTESIAN_POINT('Ctrl Pts',(-8.68497516083253,-1.17751950125305,
-0.400178411758024));
#59826=CARTESIAN_POINT('Ctrl Pts',(-8.63162448500833,-0.738867661530245,
-1.1808777591165));
#59827=CARTESIAN_POINT('Ctrl Pts',(-8.55208085779126,0.59392663665258,-1.26001938616266));
#59828=CARTESIAN_POINT('Ctrl Pts',(-8.47253723057421,1.38109257254281,-0.181606743537313));
#59829=CARTESIAN_POINT('Ctrl Pts',(-8.39299360335714,0.899476756568682,
1.06364433323544));
#59830=CARTESIAN_POINT('Ctrl Pts',(-8.3134499761401,-0.408470123411764,
1.33174692096928));
#59831=CARTESIAN_POINT('Ctrl Pts',(-8.25316307010899,-1.11536792071274,
0.607680449651806));
#59832=CARTESIAN_POINT('Ctrl Pts',(-8.2193907064836,-1.17821052692035,0.108561408848025));
#59833=CARTESIAN_POINT('Ctrl Pts',(-8.21213288526389,-1.17726943853211,
0.00106644700324865));
#59834=CARTESIAN_POINT('Origin',(-35.5608671147362,0.,0.));
#59835=CARTESIAN_POINT('',(-9.31086711473623,-1.17620260599838,0.000684878377940163));
#59836=CARTESIAN_POINT('',(-9.21213288526389,-1.17700074425756,-0.00102218139484231));
#59837=CARTESIAN_POINT('',(-35.5608671147362,-1.17775,1.38253677383905E-12));
#59838=CARTESIAN_POINT('Ctrl Pts',(-9.31086711473623,-1.17620260599838,
0.000684878377940155));
#59839=CARTESIAN_POINT('Ctrl Pts',(-9.29460571574348,-1.17492956671425,
-0.240712289578281));
#59840=CARTESIAN_POINT('Ctrl Pts',(-9.25182977434505,-0.984958310030366,
-0.877551160602252));
#59841=CARTESIAN_POINT('Ctrl Pts',(-9.18253929054092,0.0582356635878705,
-1.3917637520418));
#59842=CARTESIAN_POINT('Ctrl Pts',(-9.10299566332388,1.20229459640314,-0.703480943217913));
#59843=CARTESIAN_POINT('Ctrl Pts',(-9.02345203610679,1.24182985382652,0.631075548691406));
#59844=CARTESIAN_POINT('Ctrl Pts',(-8.94390840888976,0.140521196236644,
1.38587572582076));
#59845=CARTESIAN_POINT('Ctrl Pts',(-8.87304676843288,-0.955586084668702,
0.92407937504744));
#59846=CARTESIAN_POINT('Ctrl Pts',(-8.82869967038171,-1.17473396925088,
0.263501653288927));
#59847=CARTESIAN_POINT('Ctrl Pts',(-8.81086711473623,-1.17669902819161,
-0.000938630091047495));
#59848=CARTESIAN_POINT('Ctrl Pts',(-9.21213288526389,-1.17700074425756,
-0.0010221813948424));
#59849=CARTESIAN_POINT('Ctrl Pts',(-9.20423188201851,-1.17796598494008,
-0.118110947805483));
#59850=CARTESIAN_POINT('Ctrl Pts',(-9.16981633636744,-1.10803357457856,
-0.627004213361478));
#59851=CARTESIAN_POINT('Ctrl Pts',(-9.10888624831068,-0.37606182780791,
-1.34125881353932));
#59852=CARTESIAN_POINT('Ctrl Pts',(-9.02934262109362,0.925000425181733,
-1.04152384353156));
#59853=CARTESIAN_POINT('Ctrl Pts',(-8.94979899387657,1.37628353717109,0.215037970003031));
#59854=CARTESIAN_POINT('Ctrl Pts',(-8.87025536665949,0.563202860613652,
1.27404875928191));
#59855=CARTESIAN_POINT('Ctrl Pts',(-8.79103333045528,-0.761901787005847,
1.16306729225316));
#59856=CARTESIAN_POINT('Ctrl Pts',(-8.73832583665674,-1.17927062333932,
0.385791649689134));
#59857=CARTESIAN_POINT('Ctrl Pts',(-8.71213288526389,-1.17968925837541,
-8.91737166363286E-5));
#59858=CARTESIAN_POINT('Origin',(-35.5608671147362,0.,0.));
#59859=CARTESIAN_POINT('',(-9.81086711473622,-1.17920857465814,0.00067940234225231));
#59860=CARTESIAN_POINT('',(-9.71213288526389,-1.17602308153073,0.000524756514563435));
#59861=CARTESIAN_POINT('',(-35.5608671147362,-1.17775,1.38253677383905E-12));
#59862=CARTESIAN_POINT('Ctrl Pts',(-9.81086711473622,-1.17920857465814,
0.000679402342252224));
#59863=CARTESIAN_POINT('Ctrl Pts',(-9.78702630351093,-1.17679579427288,
-0.350929376268994));
#59864=CARTESIAN_POINT('Ctrl Pts',(-9.73667094987996,-0.823009981098092,
-1.0977918872868));
#59865=CARTESIAN_POINT('Ctrl Pts',(-9.65980105384327,0.448163591769547,
-1.31891892435554));
#59866=CARTESIAN_POINT('Ctrl Pts',(-9.58025742662623,1.35183301838504,-0.33607324263468));
#59867=CARTESIAN_POINT('Ctrl Pts',(-9.50071379940917,1.0136008524543,0.955516114942553));
#59868=CARTESIAN_POINT('Ctrl Pts',(-9.42117017219209,-0.255805871095256,
1.36929218588443));
#59869=CARTESIAN_POINT('Ctrl Pts',(-9.35788794396779,-1.07874206960061,
0.697703046197374));
#59870=CARTESIAN_POINT('Ctrl Pts',(-9.32112025814917,-1.17700528320692,
0.152890711568344));
#59871=CARTESIAN_POINT('Ctrl Pts',(-9.31086711473623,-1.17620260599838,
0.000684878377940155));
#59872=CARTESIAN_POINT('Ctrl Pts',(-9.71213288526389,-1.17602308153073,
0.000524756514563435));
#59873=CARTESIAN_POINT('Ctrl Pts',(-9.69665246978596,-1.17510280305878,
-0.229366621244868));
#59874=CARTESIAN_POINT('Ctrl Pts',(-9.65465751190234,-0.99878260724446,
-0.854314884247616));
#59875=CARTESIAN_POINT('Ctrl Pts',(-9.58614801161304,0.0172395002259546,
-1.39287490567643));
#59876=CARTESIAN_POINT('Ctrl Pts',(-9.50660438439598,1.18106435331442,-0.738569357989597));
#59877=CARTESIAN_POINT('Ctrl Pts',(-9.42706075717891,1.25986932500286,0.59424488819676));
#59878=CARTESIAN_POINT('Ctrl Pts',(-9.34751712996187,0.181257885165623,
1.3811384008478));
#59879=CARTESIAN_POINT('Ctrl Pts',(-9.27587450599017,-0.940193819229214,
0.947077805540203));
#59880=CARTESIAN_POINT('Ctrl Pts',(-9.23074642442419,-1.17472678680111,
0.274820806024488));
#59881=CARTESIAN_POINT('Ctrl Pts',(-9.21213288526389,-1.17700074425756,
-0.0010221813948424));
#59882=CARTESIAN_POINT('Origin',(-35.5608671147362,0.,0.));
#59883=CARTESIAN_POINT('',(-10.3108671147362,-1.17832052192974,-0.00102120244541717));
#59884=CARTESIAN_POINT('',(-10.2121328852639,-1.17892853960487,0.000829332411371141));
#59885=CARTESIAN_POINT('',(-35.5608671147362,-1.17775,1.38253677383905E-12));
#59886=CARTESIAN_POINT('Ctrl Pts',(-10.3108671147362,-1.17832052192974,
-0.0010212024454173));
#59887=CARTESIAN_POINT('Ctrl Pts',(-10.3059614336841,-1.17898318451254,
-0.073513146495671));
#59888=CARTESIAN_POINT('Ctrl Pts',(-10.2745412102262,-1.13983029700994,
-0.537100248604522));
#59889=CARTESIAN_POINT('Ctrl Pts',(-10.2166064443627,-0.524801368121128,
-1.29034152766978));
#59890=CARTESIAN_POINT('Ctrl Pts',(-10.1370628171456,0.801749170760637,
-1.13912071405783));
#59891=CARTESIAN_POINT('Ctrl Pts',(-10.0575191899286,1.39174899779504,0.0585872097601163));
#59892=CARTESIAN_POINT('Ctrl Pts',(-9.97797556271153,0.703177231089948,
1.20247225152501));
#59893=CARTESIAN_POINT('Ctrl Pts',(-9.89843193549446,-0.63138920452485,
1.24167040973862));
#59894=CARTESIAN_POINT('Ctrl Pts',(-9.84272911950269,-1.15976589559383,
0.470312429397423));
#59895=CARTESIAN_POINT('Ctrl Pts',(-9.81354084591662,-1.17947916637948,
0.0401120938638806));
#59896=CARTESIAN_POINT('Ctrl Pts',(-9.81086711473622,-1.17920857465814,
0.000679402342252224));
#59897=CARTESIAN_POINT('Ctrl Pts',(-10.2121328852639,-1.17892853960487,
0.000829332411371106));
#59898=CARTESIAN_POINT('Ctrl Pts',(-10.1890730575534,-1.17620975931657,
-0.339473117241695));
#59899=CARTESIAN_POINT('Ctrl Pts',(-10.1394986874372,-0.842127078826765,
-1.07571404946627));
#59900=CARTESIAN_POINT('Ctrl Pts',(-10.0634097749154,0.40914284781568,-1.33154039867832));
#59901=CARTESIAN_POINT('Ctrl Pts',(-9.98386614769835,1.34135376086346,-0.375723024911412));
#59902=CARTESIAN_POINT('Ctrl Pts',(-9.90432252048127,1.04129016283722,0.9252634759946));
#59903=CARTESIAN_POINT('Ctrl Pts',(-9.82477889326422,-0.215385600998657,
1.3762291764505));
#59904=CARTESIAN_POINT('Ctrl Pts',(-9.76071568152509,-1.06813113821466,
0.721171110256381));
#59905=CARTESIAN_POINT('Ctrl Pts',(-9.72316701219165,-1.17667903740497,
0.164386679045683));
#59906=CARTESIAN_POINT('Ctrl Pts',(-9.71213288526389,-1.17602308153073,
0.000524756514563435));
#59907=CARTESIAN_POINT('Origin',(-35.5608671147362,0.,0.));
#59908=CARTESIAN_POINT('',(-10.8108671147362,-1.17582670261709,-0.000188998789078225));
#59909=CARTESIAN_POINT('',(-10.7121328852639,-1.17865848830409,-0.000932771918738112));
#59910=CARTESIAN_POINT('',(-35.5608671147362,-1.17775,1.38253677383905E-12));
#59911=CARTESIAN_POINT('Ctrl Pts',(-10.8108671147362,-1.17582670261709,
-0.000188998789078139));
#59912=CARTESIAN_POINT('Ctrl Pts',(-10.7983820214515,-1.176091511301,-0.185675751126754));
#59913=CARTESIAN_POINT('Ctrl Pts',(-10.7593823857611,-1.04720114782861,
-0.764732004625058));
#59914=CARTESIAN_POINT('Ctrl Pts',(-10.6938682076651,-0.139821056801252,
-1.38594653796095));
#59915=CARTESIAN_POINT('Ctrl Pts',(-10.614324580448,1.09031954355872,-0.866949264343001));
#59916=CARTESIAN_POINT('Ctrl Pts',(-10.534780953231,1.31880567985816,0.4484967255007));
#59917=CARTESIAN_POINT('Ctrl Pts',(-10.4552373260139,0.335731770057017,
1.35191786458549));
#59918=CARTESIAN_POINT('Ctrl Pts',(-10.380599379849,-0.876121404964598,
1.03423932121344));
#59919=CARTESIAN_POINT('Ctrl Pts',(-10.3324759760898,-1.175401582903,0.318296003784583));
#59920=CARTESIAN_POINT('Ctrl Pts',(-10.3108671147362,-1.17832052192974,
-0.0010212024454173));
#59921=CARTESIAN_POINT('Ctrl Pts',(-10.7121328852639,-1.17865848830409,
-0.00093277191873813));
#59922=CARTESIAN_POINT('Ctrl Pts',(-10.7080081877265,-1.17918638551096,
-0.0618387895771099));
#59923=CARTESIAN_POINT('Ctrl Pts',(-10.6773689477835,-1.14715919296215,
-0.513706649318993));
#59924=CARTESIAN_POINT('Ctrl Pts',(-10.6202151654348,-0.562559160376593,
-1.27433311748048));
#59925=CARTESIAN_POINT('Ctrl Pts',(-10.5406715382178,0.767868104821389,
-1.1622290122128));
#59926=CARTESIAN_POINT('Ctrl Pts',(-10.4611279110007,1.39287050668653,0.0175913283742381));
#59927=CARTESIAN_POINT('Ctrl Pts',(-10.3815842837836,0.73827100732634,1.18125087215736));
#59928=CARTESIAN_POINT('Ctrl Pts',(-10.3020406565666,-0.594563101826563,
1.25971918346015));
#59929=CARTESIAN_POINT('Ctrl Pts',(-10.24555685706,-1.15314141439117,0.493657848568567));
#59930=CARTESIAN_POINT('Ctrl Pts',(-10.2155875999591,-1.17933585445271,
0.0518118414046211));
#59931=CARTESIAN_POINT('Ctrl Pts',(-10.2121328852639,-1.17892853960487,
0.000829332411371106));
#59932=CARTESIAN_POINT('Origin',(-35.5608671147362,0.,0.));
#59933=CARTESIAN_POINT('',(-11.3108671147362,-1.17762466953345,0.00108839146631162));
#59934=CARTESIAN_POINT('',(-11.2121328852639,-1.17590941904104,-0.000374468625826685));
#59935=CARTESIAN_POINT('',(-35.5608671147362,-1.17775,1.38253677383905E-12));
#59936=CARTESIAN_POINT('Ctrl Pts',(-11.3108671147362,-1.17762466953345,
0.00108839146631154));
#59937=CARTESIAN_POINT('Ctrl Pts',(-11.290802609219,-1.17490239677762,-0.295857233741433));
#59938=CARTESIAN_POINT('Ctrl Pts',(-11.244223561296,-0.910167371062506,
-0.989528333638478));
#59939=CARTESIAN_POINT('Ctrl Pts',(-11.1711299709674,0.256497582227027,
-1.36916278225881));
#59940=CARTESIAN_POINT('Ctrl Pts',(-11.0915863437504,1.2904740469978,-0.52447542176553));
#59941=CARTESIAN_POINT('Ctrl Pts',(-11.0120427165333,1.13891816249902,0.802036877668863));
#59942=CARTESIAN_POINT('Ctrl Pts',(-10.9324990893162,-0.0589387521943207,
1.39173415475109));
#59943=CARTESIAN_POINT('Ctrl Pts',(-10.8654405553839,-1.02313400954157,
0.810996401841933));
#59944=CARTESIAN_POINT('Ctrl Pts',(-10.8248965638572,-1.17552913816377,
0.208241718963453));
#59945=CARTESIAN_POINT('Ctrl Pts',(-10.8108671147362,-1.17582670261709,
-0.000188998789078139));
#59946=CARTESIAN_POINT('Ctrl Pts',(-11.2121328852639,-1.17590941904104,
-0.000374468625826806));
#59947=CARTESIAN_POINT('Ctrl Pts',(-11.200428775494,-1.17640320837023,-0.174227904069011));
#59948=CARTESIAN_POINT('Ctrl Pts',(-11.1622101233184,-1.05866553135645,
-0.74129353109382));
#59949=CARTESIAN_POINT('Ctrl Pts',(-11.0974769287372,-0.18056013375031,
-1.38122979309427));
#59950=CARTESIAN_POINT('Ctrl Pts',(-11.0179333015201,1.06432562899421,-0.898670495063273));
#59951=CARTESIAN_POINT('Ctrl Pts',(-10.938389674303,1.33143701009596,0.409479170871799));
#59952=CARTESIAN_POINT('Ctrl Pts',(-10.858846047086,0.375384198042811,1.34144862260576));
#59953=CARTESIAN_POINT('Ctrl Pts',(-10.7834271174063,-0.858068354441969,
1.0566331129145));
#59954=CARTESIAN_POINT('Ctrl Pts',(-10.7345227301322,-1.17579293599113,
0.329679660768861));
#59955=CARTESIAN_POINT('Ctrl Pts',(-10.7121328852639,-1.17865848830409,
-0.00093277191873813));
#59956=CARTESIAN_POINT('Origin',(-35.5608671147362,0.,0.));
#59957=CARTESIAN_POINT('',(-11.8108671147362,-1.17960016821189,-0.000308426038616608));
#59958=CARTESIAN_POINT('',(-11.7121328852639,-1.17728095270416,0.00106778596620033));
#59959=CARTESIAN_POINT('',(-35.5608671147362,-1.17775,1.38253677383905E-12));
#59960=CARTESIAN_POINT('Ctrl Pts',(-11.8108671147362,-1.17960016821189,
-0.000308426038616535));
#59961=CARTESIAN_POINT('Ctrl Pts',(-11.8097377393921,-1.17965824466903,
-0.0169500240275318));
#59962=CARTESIAN_POINT('Ctrl Pts',(-11.7820938216423,-1.17178738065343,
-0.424233150976045));
#59963=CARTESIAN_POINT('Ctrl Pts',(-11.7279353614868,-0.702569672259767,
-1.20282733159494));
#59964=CARTESIAN_POINT('Ctrl Pts',(-11.6483917342698,0.632016395318918,
-1.2413512839076));
#59965=CARTESIAN_POINT('Ctrl Pts',(-11.5688481070527,1.38598181139171,-0.139470973691));
#59966=CARTESIAN_POINT('Ctrl Pts',(-11.4893044798357,0.866673830973786,
1.09053849300069));
#59967=CARTESIAN_POINT('Ctrl Pts',(-11.4097608526186,-0.448829830616605,
1.31869235121755));
#59968=CARTESIAN_POINT('Ctrl Pts',(-11.3502817309188,-1.12418153891304,
0.583423595664754));
#59969=CARTESIAN_POINT('Ctrl Pts',(-11.3173171516247,-1.17849978502934,
0.0965460260839821));
#59970=CARTESIAN_POINT('Ctrl Pts',(-11.3108671147362,-1.17762466953345,
0.00108839146631154));
#59971=CARTESIAN_POINT('Ctrl Pts',(-11.7121328852639,-1.17728095270416,
0.00106778596620021));
#59972=CARTESIAN_POINT('Ctrl Pts',(-11.6928493632614,-1.17477548883292,
-0.284531699071451));
#59973=CARTESIAN_POINT('Ctrl Pts',(-11.6470512988533,-0.926562106106686,
-0.966727326674524));
#59974=CARTESIAN_POINT('Ctrl Pts',(-11.5747386920395,0.216080821741205,
-1.37612019159185));
#59975=CARTESIAN_POINT('Ctrl Pts',(-11.4951950648225,1.27447517462567,-0.562237256408714));
#59976=CARTESIAN_POINT('Ctrl Pts',(-11.4156514376054,1.16203501799428,0.768161649775757));
#59977=CARTESIAN_POINT('Ctrl Pts',(-11.3361078103884,-0.0179431554001853,
1.39286601882789));
#59978=CARTESIAN_POINT('Ctrl Pts',(-11.2682682929412,-1.010239900524,0.834334123584145));
#59979=CARTESIAN_POINT('Ctrl Pts',(-11.2269433178997,-1.17528457582444,
0.219620442970041));
#59980=CARTESIAN_POINT('Ctrl Pts',(-11.2121328852639,-1.17590941904104,
-0.000374468625826806));
#59981=CARTESIAN_POINT('Origin',(-35.5608671147362,0.,0.));
#59982=CARTESIAN_POINT('',(-12.3108671147362,-1.17668924014875,-0.000935216629109687));
#59983=CARTESIAN_POINT('',(-12.2121328852639,-1.17968782784267,-9.65820520404392E-5));
#59984=CARTESIAN_POINT('',(-35.5608671147362,-1.17775,1.38253677383905E-12));
#59985=CARTESIAN_POINT('Ctrl Pts',(-12.3108671147362,-1.17668924014875,
-0.000935216629109649));
#59986=CARTESIAN_POINT('Ctrl Pts',(-12.3021583271596,-1.17764488283097,
-0.130081176142648));
#59987=CARTESIAN_POINT('Ctrl Pts',(-12.2669349971772,-1.09841677303328,
-0.651281554432957));
#59988=CARTESIAN_POINT('Ctrl Pts',(-12.2051971247892,-0.335048760661853,
-1.35208729821336));
#59989=CARTESIAN_POINT('Ctrl Pts',(-12.1256534975721,0.956283922151258,
-1.01287649506048));
#59990=CARTESIAN_POINT('Ctrl Pts',(-12.0461098703551,1.36909794940973,0.256843413256152));
#59991=CARTESIAN_POINT('Ctrl Pts',(-11.966566243138,0.524149441947044,1.29060648399021));
#59992=CARTESIAN_POINT('Ctrl Pts',(-11.8881519912651,-0.783491007014861,
1.14087211442108));
#59993=CARTESIAN_POINT('Ctrl Pts',(-11.8362522817978,-1.17829477353105,
0.373747681458496));
#59994=CARTESIAN_POINT('Ctrl Pts',(-11.8108671147362,-1.17960016821189,
-0.000308426038616535));
#59995=CARTESIAN_POINT('Ctrl Pts',(-12.2121328852639,-1.17968782784267,
-9.65820520404728E-5));
#59996=CARTESIAN_POINT('Ctrl Pts',(-12.2117844934346,-1.17969384319053,
-0.00522919056453987));
#59997=CARTESIAN_POINT('Ctrl Pts',(-12.1849215591996,-1.17733532698894,
-0.400975971111822));
#59998=CARTESIAN_POINT('Ctrl Pts',(-12.1315440825589,-0.737674164708033,
-1.18162368373076));
#59999=CARTESIAN_POINT('Ctrl Pts',(-12.0520004553419,0.595199415261899,
-1.25941865926429));
#60000=CARTESIAN_POINT('Ctrl Pts',(-11.9724568281248,1.3812753570299,-0.180211240751194));
#60001=CARTESIAN_POINT('Ctrl Pts',(-11.8929132009078,0.898401626530242,
1.06455259178631));
#60002=CARTESIAN_POINT('Ctrl Pts',(-11.8133695736907,-0.409815467802085,
1.33133353656448));
#60003=CARTESIAN_POINT('Ctrl Pts',(-11.7531094684761,-1.11566740233522,
0.606875413125733));
#60004=CARTESIAN_POINT('Ctrl Pts',(-11.7193639056671,-1.17822046263239,
0.108163144542644));
#60005=CARTESIAN_POINT('Ctrl Pts',(-11.7121328852639,-1.17728095270416,
0.00106778596620021));
#60006=CARTESIAN_POINT('Origin',(-35.5608671147362,0.,0.));
#60007=CARTESIAN_POINT('',(-12.8108671147362,-1.17620961977275,0.000690027712506509));
#60008=CARTESIAN_POINT('',(-12.7121328852639,-1.17698990462219,-0.00101984215893941));
#60009=CARTESIAN_POINT('',(-35.5608671147362,-1.17775,1.38253677383905E-12));
#60010=CARTESIAN_POINT('Ctrl Pts',(-12.8108671147362,-1.17620961977275,
0.000690027712506418));
#60011=CARTESIAN_POINT('Ctrl Pts',(-12.794578914927,-1.17492443634169,-0.24110138251064));
#60012=CARTESIAN_POINT('Ctrl Pts',(-12.7517761727121,-0.984474855720211,
-0.878347397724903));
#60013=CARTESIAN_POINT('Ctrl Pts',(-12.6824588880915,0.0596418257590296,
-1.39170420227544));
#60014=CARTESIAN_POINT('Ctrl Pts',(-12.6029152608745,1.2030047565203,-0.702265825596333));
#60015=CARTESIAN_POINT('Ctrl Pts',(-12.5233716336574,1.24119160218488,0.632329930239507));
#60016=CARTESIAN_POINT('Ctrl Pts',(-12.4438280064404,0.139120881682115,
1.38601699639326));
#60017=CARTESIAN_POINT('Ctrl Pts',(-12.3729931668,-0.956104870347375,0.923288487221614));
#60018=CARTESIAN_POINT('Ctrl Pts',(-12.3286728695652,-1.17473535860622,
0.263113168064762));
#60019=CARTESIAN_POINT('Ctrl Pts',(-12.3108671147362,-1.17668924014875,
-0.000935216629109649));
#60020=CARTESIAN_POINT('Ctrl Pts',(-12.7121328852639,-1.17698990462219,
-0.00101984215893938));
#60021=CARTESIAN_POINT('Ctrl Pts',(-12.704205081202,-1.17795555935218,-0.11850851884417));
#60022=CARTESIAN_POINT('Ctrl Pts',(-12.6697627347345,-1.10772178842638,
-0.62780956583934));
#60023=CARTESIAN_POINT('Ctrl Pts',(-12.6088058458613,-0.374706472475756,
-1.34163808932065));
#60024=CARTESIAN_POINT('Ctrl Pts',(-12.5292622186442,0.926052274160795,
-1.04058872219181));
#60025=CARTESIAN_POINT('Ctrl Pts',(-12.4497185914272,1.37606556746074,0.216428411443782));
#60026=CARTESIAN_POINT('Ctrl Pts',(-12.3701749642101,0.561915316568623,
1.27461715045607));
#60027=CARTESIAN_POINT('Ctrl Pts',(-12.2909797288224,-0.762628277933677,
1.1623348962687));
#60028=CARTESIAN_POINT('Ctrl Pts',(-12.2382990358403,-1.17923604199531,
0.385390665053393));
#60029=CARTESIAN_POINT('Ctrl Pts',(-12.2121328852639,-1.17968782784267,
-9.65820520404728E-5));
#60030=CARTESIAN_POINT('Origin',(-35.5608671147362,0.,0.));
#60031=CARTESIAN_POINT('',(-13.3108671147362,-1.1792173683553,0.000673743327001118));
#60032=CARTESIAN_POINT('',(-13.2121328852639,-1.17602842142206,0.000530545984581826));
#60033=CARTESIAN_POINT('',(-35.5608671147362,-1.17775,1.38253677383905E-12));
#60034=CARTESIAN_POINT('Ctrl Pts',(-13.3108671147362,-1.1792173683553,0.000673743327001138));
#60035=CARTESIAN_POINT('Ctrl Pts',(-13.2869995026945,-1.17681788725409,
-0.351323391984844));
#60036=CARTESIAN_POINT('Ctrl Pts',(-13.236617348247,-0.822343662973783,
-1.09854622043971));
#60037=CARTESIAN_POINT('Ctrl Pts',(-13.1597206513939,0.449495954917602,
-1.3184654415356));
#60038=CARTESIAN_POINT('Ctrl Pts',(-13.0801770241768,1.35217188563002,-0.334707223887899));
#60039=CARTESIAN_POINT('Ctrl Pts',(-13.0006333969598,1.01263491332703,0.956539735882493));
#60040=CARTESIAN_POINT('Ctrl Pts',(-12.9210897697427,-0.25718922789799,
1.36903302920864));
#60041=CARTESIAN_POINT('Ctrl Pts',(-12.8578343423349,-1.07909821874922,
0.696897543302798));
#60042=CARTESIAN_POINT('Ctrl Pts',(-12.8210934573327,-1.17701650612111,
0.152495741468027));
#60043=CARTESIAN_POINT('Ctrl Pts',(-12.8108671147362,-1.17620961977275,
0.000690027712506418));
#60044=CARTESIAN_POINT('Ctrl Pts',(-13.2121328852639,-1.17602842142206,
0.000530545984581809));
#60045=CARTESIAN_POINT('Ctrl Pts',(-13.1966256689695,-1.17509613497152,
-0.229756223488072));
#60046=CARTESIAN_POINT('Ctrl Pts',(-13.1546039102694,-0.998316605074535,
-0.855113302780238));
#60047=CARTESIAN_POINT('Ctrl Pts',(-13.0860676091637,0.0186468059951288,
-1.39285677650551));
#60048=CARTESIAN_POINT('Ctrl Pts',(-13.0065239819466,1.18180997643742,-0.737375672791089));
#60049=CARTESIAN_POINT('Ctrl Pts',(-12.9269803547296,1.25926827663031,0.595517515026806));
#60050=CARTESIAN_POINT('Ctrl Pts',(-12.8474367275125,0.179862336254169,
1.38132083283659));
#60051=CARTESIAN_POINT('Ctrl Pts',(-12.7758209043573,-0.940730875292218,
0.946290183190409));
#60052=CARTESIAN_POINT('Ctrl Pts',(-12.7307196236077,-1.17472592689814,
0.274432385832564));
#60053=CARTESIAN_POINT('Ctrl Pts',(-12.7121328852639,-1.17698990462219,
-0.00101984215893938));
#60054=CARTESIAN_POINT('Origin',(-35.5608671147362,0.,0.));
#60055=CARTESIAN_POINT('',(-13.8108671147362,-1.1783086217086,-0.00102359871729984));
#60056=CARTESIAN_POINT('',(-13.7121328852639,-1.17893883534851,0.000824692032647192));
#60057=CARTESIAN_POINT('',(-35.5608671147362,-1.17775,1.38253677383905E-12));
#60058=CARTESIAN_POINT('Ctrl Pts',(-13.8108671147362,-1.1783086217086,-0.0010235987173));
#60059=CARTESIAN_POINT('Ctrl Pts',(-13.8059346328676,-1.17897568560547,
-0.0739134811648439));
#60060=CARTESIAN_POINT('Ctrl Pts',(-13.7744876085933,-1.13957191331326,
-0.537903456860039));
#60061=CARTESIAN_POINT('Ctrl Pts',(-13.7165260419133,-0.523497382004637,
-1.29087111093451));
#60062=CARTESIAN_POINT('Ctrl Pts',(-13.6369824146963,0.802899691287971,
-1.13831007187878));
#60063=CARTESIAN_POINT('Ctrl Pts',(-13.5574387874792,1.39168909284562,0.05999335684464));
#60064=CARTESIAN_POINT('Ctrl Pts',(-13.4778951602621,0.701961934126549,
1.20318210469084));
#60065=CARTESIAN_POINT('Ctrl Pts',(-13.3983515330451,-0.632643424815839,
1.24103184127092));
#60066=CARTESIAN_POINT('Ctrl Pts',(-13.3426755178698,-1.15998664398442,
0.469511787720473));
#60067=CARTESIAN_POINT('Ctrl Pts',(-13.3135140451002,-1.17948347203477,
0.0397104053879535));
#60068=CARTESIAN_POINT('Ctrl Pts',(-13.3108671147362,-1.1792173683553,0.000673743327001138));
#60069=CARTESIAN_POINT('Ctrl Pts',(-13.7121328852639,-1.17893883534851,
0.000824692032647123));
#60070=CARTESIAN_POINT('Ctrl Pts',(-13.6890462567369,-1.17622805273099,
-0.339865495247411));
#60071=CARTESIAN_POINT('Ctrl Pts',(-13.6394450858043,-0.841480609154534,
-1.07647469321775));
#60072=CARTESIAN_POINT('Ctrl Pts',(-13.563329372466,0.410487983199367,-1.33112633468056));
#60073=CARTESIAN_POINT('Ctrl Pts',(-13.483785745249,1.34173269428113,-0.374367573820533));
#60074=CARTESIAN_POINT('Ctrl Pts',(-13.4042421180319,1.04035477583892,0.92631508873616));
#60075=CARTESIAN_POINT('Ctrl Pts',(-13.3246984908148,-0.216775987337669,
1.37601085553309));
#60076=CARTESIAN_POINT('Ctrl Pts',(-13.2606620798922,-1.06850277171503,
0.720365941468082));
#60077=CARTESIAN_POINT('Ctrl Pts',(-13.2231402113752,-1.17669017662013,
0.163992609232004));
#60078=CARTESIAN_POINT('Ctrl Pts',(-13.2121328852639,-1.17602842142206,
0.000530545984581809));
#60079=CARTESIAN_POINT('Origin',(-35.5608671147362,0.,0.));
#60080=CARTESIAN_POINT('',(-14.3108671147362,-1.17582483899281,-0.0001825003029064));
#60081=CARTESIAN_POINT('',(-14.2121328852639,-1.17864724066233,-0.000936392280242448));
#60082=CARTESIAN_POINT('',(-35.5608671147362,-1.17775,1.38253677383905E-12));
#60083=CARTESIAN_POINT('Ctrl Pts',(-14.3108671147362,-1.17582483899281,
-0.00018250030290639));
#60084=CARTESIAN_POINT('Ctrl Pts',(-14.2983552206351,-1.17608106896736,
-0.186068157712449));
#60085=CARTESIAN_POINT('Ctrl Pts',(-14.2593287841282,-1.04679940493409,
-0.765535917678041));
#60086=CARTESIAN_POINT('Ctrl Pts',(-14.1937878052157,-0.138420671057853,
-1.38608710109966));
#60087=CARTESIAN_POINT('Ctrl Pts',(-14.1142441779986,1.09119492379563,-0.865847199160223));
#60088=CARTESIAN_POINT('Ctrl Pts',(-14.0347005507816,1.31835186050876,0.449828974060237));
#60089=CARTESIAN_POINT('Ctrl Pts',(-13.9551569235645,0.334365665758747,
1.3522563867746));
#60090=CARTESIAN_POINT('Ctrl Pts',(-13.880545778216,-0.876730884968787,
1.03346810019051));
#60091=CARTESIAN_POINT('Ctrl Pts',(-13.8324491752733,-1.1753898855048,0.317905876834171));
#60092=CARTESIAN_POINT('Ctrl Pts',(-13.8108671147362,-1.1783086217086,-0.0010235987173));
#60093=CARTESIAN_POINT('Ctrl Pts',(-14.2121328852639,-1.17864724066233,
-0.00093639228024244));
#60094=CARTESIAN_POINT('Ctrl Pts',(-14.2079813869101,-1.1791799169808,-0.062239674349538));
#60095=CARTESIAN_POINT('Ctrl Pts',(-14.1773153461506,-1.14691406887258,
-0.514509039350729));
#60096=CARTESIAN_POINT('Ctrl Pts',(-14.1201347629855,-0.561271329354032,
-1.27490085813617));
#60097=CARTESIAN_POINT('Ctrl Pts',(-14.0405911357683,0.769041990499703,
-1.16145259054315));
#60098=CARTESIAN_POINT('Ctrl Pts',(-13.9610475085513,1.39285202204237,0.0189986295192388));
#60099=CARTESIAN_POINT('Ctrl Pts',(-13.8815038813343,0.737077133827655,
1.18199619374158));
#60100=CARTESIAN_POINT('Ctrl Pts',(-13.8019602541172,-0.595835576796184,
1.25911781365174));
#60101=CARTESIAN_POINT('Ctrl Pts',(-13.7455032554271,-1.15337493066883,
0.492856254368816));
#60102=CARTESIAN_POINT('Ctrl Pts',(-13.7155607991426,-1.17934133367546,
0.0514105374266761));
#60103=CARTESIAN_POINT('Ctrl Pts',(-13.7121328852639,-1.17893883534851,
0.000824692032647123));
#60104=CARTESIAN_POINT('Origin',(-35.5608671147362,0.,0.));
#60105=CARTESIAN_POINT('',(-14.8108671147362,-1.17763668317489,0.00108845679832357));
#60106=CARTESIAN_POINT('',(-14.7121328852639,-1.17590568010642,-0.000368259996795101));
#60107=CARTESIAN_POINT('',(-35.5608671147362,-1.17775,1.38253677383905E-12));
#60108=CARTESIAN_POINT('Ctrl Pts',(-14.8108671147362,-1.17763668317489,
0.00108845679832346));
#60109=CARTESIAN_POINT('Ctrl Pts',(-14.7907758084025,-1.1749081691312,-0.296246069770847));
#60110=CARTESIAN_POINT('Ctrl Pts',(-14.7441699596631,-0.90959503482556,
-0.990308665309722));
#60111=CARTESIAN_POINT('Ctrl Pts',(-14.6710495685181,0.25788080793157,-1.36890292676711));
#60112=CARTESIAN_POINT('Ctrl Pts',(-14.591505941301,1.2910033008695,-0.523171301922277));
#60113=CARTESIAN_POINT('Ctrl Pts',(-14.5119623140839,1.13810722973384,0.803187193397973));
#60114=CARTESIAN_POINT('Ctrl Pts',(-14.4324186868668,-0.0603448841024907,
1.39167389462245));
#60115=CARTESIAN_POINT('Ctrl Pts',(-14.365386953751,-1.02356777266643,0.810194735888077));
#60116=CARTESIAN_POINT('Ctrl Pts',(-14.3248697630407,-1.17553807999456,
0.207850868947047));
#60117=CARTESIAN_POINT('Ctrl Pts',(-14.3108671147362,-1.17582483899281,
-0.00018250030290639));
#60118=CARTESIAN_POINT('Ctrl Pts',(-14.7121328852639,-1.17590568010642,
-0.000368259996795066));
#60119=CARTESIAN_POINT('Ctrl Pts',(-14.7004019746775,-1.17639230734852,
-0.174621178730114));
#60120=CARTESIAN_POINT('Ctrl Pts',(-14.6621565216855,-1.05827983303723,
-0.742098214484146));
#60121=CARTESIAN_POINT('Ctrl Pts',(-14.5973965262878,-0.179164492855332,
-1.38141152005153));
#60122=CARTESIAN_POINT('Ctrl Pts',(-14.5178528990707,1.06523307257745,-0.897594677077771));
#60123=CARTESIAN_POINT('Ctrl Pts',(-14.4383092718537,1.33102260634132,0.410824201623429));
#60124=CARTESIAN_POINT('Ctrl Pts',(-14.3587656446366,0.37402865127972,1.34182721363559));
#60125=CARTESIAN_POINT('Ctrl Pts',(-14.2833735157734,-0.858697287164189,
1.05586726445034));
#60126=CARTESIAN_POINT('Ctrl Pts',(-14.2344959293158,-1.17577785159837,
0.329288476095253));
#60127=CARTESIAN_POINT('Ctrl Pts',(-14.2121328852639,-1.17864724066233,
-0.00093639228024244));
#60128=CARTESIAN_POINT('Origin',(-35.5608671147362,0.,0.));
#60129=CARTESIAN_POINT('',(-15.3108671147362,-1.17959567567971,-0.000315498773397984));
#60130=CARTESIAN_POINT('',(-15.2121328852639,-1.17729248913048,0.00106908369163515));
#60131=CARTESIAN_POINT('',(-35.5608671147362,-1.17775,1.38253677383905E-12));
#60132=CARTESIAN_POINT('Ctrl Pts',(-15.3108671147362,-1.17959567567971,
-0.000315498773397779));
#60133=CARTESIAN_POINT('Ctrl Pts',(-15.3097109385756,-1.17965635862726,
-0.017352186126931));
#60134=CARTESIAN_POINT('Ctrl Pts',(-15.2820402200094,-1.17159073736189,
-0.425031809757892));
#60135=CARTESIAN_POINT('Ctrl Pts',(-15.2278549590375,-0.70135401684535,
-1.20353657072225));
#60136=CARTESIAN_POINT('Ctrl Pts',(-15.1483113318204,0.633270292855629,
-1.24071208191002));
#60137=CARTESIAN_POINT('Ctrl Pts',(-15.0687677046033,1.38612202080006,-0.138070552487189));
#60138=CARTESIAN_POINT('Ctrl Pts',(-14.9892240773863,0.865571544712346,
1.09141359483712));
#60139=CARTESIAN_POINT('Ctrl Pts',(-14.9096804501692,-0.45016196450262,
1.31823819536764));
#60140=CARTESIAN_POINT('Ctrl Pts',(-14.8502281292859,-1.12446646376063,
0.582619075676667));
#60141=CARTESIAN_POINT('Ctrl Pts',(-14.8172903508082,-1.17850899528528,
0.0961469773735007));
#60142=CARTESIAN_POINT('Ctrl Pts',(-14.8108671147362,-1.17763668317489,
0.00108845679832346));
#60143=CARTESIAN_POINT('Ctrl Pts',(-15.2121328852639,-1.17729248913048,
0.00106908369163521));
#60144=CARTESIAN_POINT('Ctrl Pts',(-15.192822562445,-1.17477855836446,-0.284920221449956));
#60145=CARTESIAN_POINT('Ctrl Pts',(-15.1469976972204,-0.92600852840609,
-0.967511697806338));
#60146=CARTESIAN_POINT('Ctrl Pts',(-15.0746582895901,0.217471097610649,
-1.37590116830213));
#60147=CARTESIAN_POINT('Ctrl Pts',(-14.9951146623731,1.27504258996775,-0.560949282020663));
#60148=CARTESIAN_POINT('Ctrl Pts',(-14.915571035156,1.16125829983559,0.76933533929888));
#60149=CARTESIAN_POINT('Ctrl Pts',(-14.836027407939,-0.0193504518311904,
1.39284717871167));
#60150=CARTESIAN_POINT('Ctrl Pts',(-14.7682146913082,-1.0106905727704,0.833534035568003));
#60151=CARTESIAN_POINT('Ctrl Pts',(-14.7269165170832,-1.17529241842247,
0.219230293332935));
#60152=CARTESIAN_POINT('Ctrl Pts',(-14.7121328852639,-1.17590568010642,
-0.000368259996795066));
#60153=CARTESIAN_POINT('Origin',(-35.5608671147362,0.,0.));
#60154=CARTESIAN_POINT('',(-15.8108671147362,-1.1766794928373,-0.000931768368600377));
#60155=CARTESIAN_POINT('',(-15.7121328852639,-1.17968628694626,-0.000103984866668544));
#60156=CARTESIAN_POINT('',(-35.5608671147362,-1.17775,1.38253677383905E-12));
#60157=CARTESIAN_POINT('Ctrl Pts',(-15.8108671147362,-1.1766794928373,-0.000931768368600226));
#60158=CARTESIAN_POINT('Ctrl Pts',(-15.8021315263431,-1.17763401370504,
-0.130477870265945));
#60159=CARTESIAN_POINT('Ctrl Pts',(-15.7668813955443,-1.0980898693991,-0.652087136442379));
#60160=CARTESIAN_POINT('Ctrl Pts',(-15.7051167223398,-0.333682485522065,
-1.352425130226));
#60161=CARTESIAN_POINT('Ctrl Pts',(-15.6255730951227,0.957306810832643,
-1.011909780536));
#60162=CARTESIAN_POINT('Ctrl Pts',(-15.5460294679057,1.36883774453492,0.258226573279226));
#60163=CARTESIAN_POINT('Ctrl Pts',(-15.4664858406886,0.52284518846023,1.29113540843514));
#60164=CARTESIAN_POINT('Ctrl Pts',(-15.3880983896322,-0.78419642644012,
1.14013154729383));
#60165=CARTESIAN_POINT('Ctrl Pts',(-15.3362254809813,-1.17826471897844,
0.373349494719946));
#60166=CARTESIAN_POINT('Ctrl Pts',(-15.3108671147362,-1.17959567567971,
-0.000315498773397779));
#60167=CARTESIAN_POINT('Ctrl Pts',(-15.7121328852639,-1.17968628694626,
-0.000103984866668646));
#60168=CARTESIAN_POINT('Ctrl Pts',(-15.7117576926181,-1.17969324372913,
-0.0056314501573956));
#60169=CARTESIAN_POINT('Ctrl Pts',(-15.6848679575667,-1.17715074290506,
-0.401773567217293));
#60170=CARTESIAN_POINT('Ctrl Pts',(-15.6314636801096,-0.736479914837584,
-1.1823684020947));
#60171=CARTESIAN_POINT('Ctrl Pts',(-15.5519200528925,0.596471586267007,
-1.2588166466993));
#60172=CARTESIAN_POINT('Ctrl Pts',(-15.4723764256754,1.38145673145398,-0.178815553998048));
#60173=CARTESIAN_POINT('Ctrl Pts',(-15.3928327984584,0.897325579366346,
1.06545976359786));
#60174=CARTESIAN_POINT('Ctrl Pts',(-15.3132891712414,-0.41116039383583,
1.3309187930794));
#60175=CARTESIAN_POINT('Ctrl Pts',(-15.2530558668431,-1.11596639612747,
0.606070391443501));
#60176=CARTESIAN_POINT('Ctrl Pts',(-15.2193371048507,-1.17823037657205,
0.107764853257028));
#60177=CARTESIAN_POINT('Ctrl Pts',(-15.2121328852639,-1.17729248913048,
0.00106908369163521));
#60178=CARTESIAN_POINT('Origin',(-35.5608671147362,0.,0.));
#60179=CARTESIAN_POINT('',(-16.3108671147362,-1.17621668823985,0.000695152040889676));
#60180=CARTESIAN_POINT('',(-16.2121328852639,-1.17697909652625,-0.00101746427987839));
#60181=CARTESIAN_POINT('',(-35.5608671147362,-1.17775,1.38253677383905E-12));
#60182=CARTESIAN_POINT('Ctrl Pts',(-16.3108671147362,-1.17621668823985,
0.000695152040889723));
#60183=CARTESIAN_POINT('Ctrl Pts',(-16.2945521141105,-1.17491936293083,
-0.24149046014261));
#60184=CARTESIAN_POINT('Ctrl Pts',(-16.2517225710792,-0.983990797500948,
-0.879143553958332));
#60185=CARTESIAN_POINT('Ctrl Pts',(-16.1823784856422,0.061047927045359,
-1.39164323179989));
#60186=CARTESIAN_POINT('Ctrl Pts',(-16.1028348584251,1.20371368856048,-0.701049991072757));
#60187=CARTESIAN_POINT('Ctrl Pts',(-16.0232912312081,1.24055208348352,0.633583666279101));
#60188=CARTESIAN_POINT('Ctrl Pts',(-15.943747603991,0.13772042510721,1.3861568520623));
#60189=CARTESIAN_POINT('Ctrl Pts',(-15.872939565167,-0.956623033777217,
0.922497494227833));
#60190=CARTESIAN_POINT('Ctrl Pts',(-15.8286460687488,-1.17473682087889,
0.262724677481997));
#60191=CARTESIAN_POINT('Ctrl Pts',(-15.8108671147362,-1.1766794928373,-0.000931768368600226));
#60192=CARTESIAN_POINT('Ctrl Pts',(-16.2121328852639,-1.17697909652625,
-0.00101746427987831));
#60193=CARTESIAN_POINT('Ctrl Pts',(-16.2041782803856,-1.17794511640517,
-0.118906061450257));
#60194=CARTESIAN_POINT('Ctrl Pts',(-16.1697091331016,-1.10740950566883,
-0.628614928672698));
#60195=CARTESIAN_POINT('Ctrl Pts',(-16.1087254434119,-0.373350734627734,
-1.34201599550232));
#60196=CARTESIAN_POINT('Ctrl Pts',(-16.0291818161949,0.927103177787362,
-1.0396525385761));
#60197=CARTESIAN_POINT('Ctrl Pts',(-15.9496381889778,1.37584619300581,0.217818631945427));
#60198=CARTESIAN_POINT('Ctrl Pts',(-15.8700945617608,0.560627198897243,
1.27518424044833));
#60199=CARTESIAN_POINT('Ctrl Pts',(-15.7909261271894,-0.763354067122768,
1.16160221950801));
#60200=CARTESIAN_POINT('Ctrl Pts',(-15.7382722350238,-1.17920161385159,
0.384989780054453));
#60201=CARTESIAN_POINT('Ctrl Pts',(-15.7121328852639,-1.17968628694626,
-0.000103984866668646));
#60202=CARTESIAN_POINT('Origin',(-35.5608671147362,0.,0.));
#60203=CARTESIAN_POINT('',(-16.8108671147362,-1.17922610211458,0.000668052266892519));
#60204=CARTESIAN_POINT('',(-16.7121328852639,-1.17603382108715,0.000536316405655574));
#60205=CARTESIAN_POINT('',(-35.5608671147362,-1.17775,1.38253677383905E-12));
#60206=CARTESIAN_POINT('Ctrl Pts',(-16.8108671147362,-1.17922610211458,
0.000668052266892499));
#60207=CARTESIAN_POINT('Ctrl Pts',(-16.786972701878,-1.17684011432817,-0.351717469786626));
#60208=CARTESIAN_POINT('Ctrl Pts',(-16.7365637466141,-0.821676660253239,
-1.09930032789078));
#60209=CARTESIAN_POINT('Ctrl Pts',(-16.6596402489445,0.450827859201633,
-1.31801061277163));
#60210=CARTESIAN_POINT('Ctrl Pts',(-16.5800966217275,1.35250937252205,-0.333340863458119));
#60211=CARTESIAN_POINT('Ctrl Pts',(-16.5005529945104,1.01166794046017,0.957562380347131));
#60212=CARTESIAN_POINT('Ctrl Pts',(-16.4210093672934,-0.258572322151341,
1.36877247496735));
#60213=CARTESIAN_POINT('Ctrl Pts',(-16.3577807407019,-1.07945384177108,
0.696092032679032));
#60214=CARTESIAN_POINT('Ctrl Pts',(-16.3210666565162,-1.17702772858213,
0.152100740472336));
#60215=CARTESIAN_POINT('Ctrl Pts',(-16.3108671147362,-1.17621668823985,
0.000695152040889723));
#60216=CARTESIAN_POINT('Ctrl Pts',(-16.7121328852639,-1.17603382108715,
0.000536316405655504));
#60217=CARTESIAN_POINT('Ctrl Pts',(-16.696598868153,-1.1750895157582,-0.230145806328667));
#60218=CARTESIAN_POINT('Ctrl Pts',(-16.6545503086365,-0.997850008706123,
-0.855911651981158));
#60219=CARTESIAN_POINT('Ctrl Pts',(-16.5859872067143,0.0200540927288029,
-1.39283722544883));
#60220=CARTESIAN_POINT('Ctrl Pts',(-16.5064435794972,1.18255439311996,-0.736181234849029));
#60221=CARTESIAN_POINT('Ctrl Pts',(-16.4268999522802,1.25866594274463,0.596789533927942));
#60222=CARTESIAN_POINT('Ctrl Pts',(-16.3473563250631,0.17846660373185,1.38150185471594));
#60223=CARTESIAN_POINT('Ctrl Pts',(-16.2757673027243,-0.941267299997083,
0.945502442243397));
#60224=CARTESIAN_POINT('Ctrl Pts',(-16.2306928227913,-1.17472514816837,
0.274043966445028));
#60225=CARTESIAN_POINT('Ctrl Pts',(-16.2121328852639,-1.17697909652625,
-0.00101746427987831));
#60226=CARTESIAN_POINT('Origin',(-35.5608671147362,0.,0.));
#60227=CARTESIAN_POINT('',(-17.3108671147362,-1.17829670657796,-0.00102595198748888));
#60228=CARTESIAN_POINT('',(-17.2121328852639,-1.17894908727537,0.000820014261101384));
#60229=CARTESIAN_POINT('',(-35.5608671147362,-1.17775,1.38253677383905E-12));
#60230=CARTESIAN_POINT('Ctrl Pts',(-17.3108671147362,-1.17829670657796,
-0.00102595198748913));
#60231=CARTESIAN_POINT('Ctrl Pts',(-17.3059078320511,-1.17896815298064,
-0.0743137955243832));
#60232=CARTESIAN_POINT('Ctrl Pts',(-17.2744340069604,-1.13931306984172,
-0.538706691640527));
#60233=CARTESIAN_POINT('Ctrl Pts',(-17.2164456394639,-0.522192861480347,
-1.29139937642464));
#60234=CARTESIAN_POINT('Ctrl Pts',(-17.1369020122469,0.804049392182112,
-1.13749826766574));
#60235=CARTESIAN_POINT('Ctrl Pts',(-17.0573583850298,1.39162776720246,0.0613994426854746));
#60236=CARTESIAN_POINT('Ctrl Pts',(-16.9778147578128,0.700745920571368,
1.20389072959865));
#60237=CARTESIAN_POINT('Ctrl Pts',(-16.8982711305957,-0.63389699927829,
1.24039200590658));
#60238=CARTESIAN_POINT('Ctrl Pts',(-16.8426219162368,-1.16020695868756,
0.468711179705086));
#60239=CARTESIAN_POINT('Ctrl Pts',(-16.8134872442837,-1.17948773637762,
0.0393087053733596));
#60240=CARTESIAN_POINT('Ctrl Pts',(-16.8108671147362,-1.17922610211458,
0.000668052266892499));
#60241=CARTESIAN_POINT('Ctrl Pts',(-17.2121328852639,-1.17894908727537,
0.000820014261101471));
#60242=CARTESIAN_POINT('Ctrl Pts',(-17.1890194559205,-1.17624647302594,
-0.340257924082543));
#60243=CARTESIAN_POINT('Ctrl Pts',(-17.1393914841714,-0.84083346165202,
-1.07723512885116));
#60244=CARTESIAN_POINT('Ctrl Pts',(-17.0632489700166,0.411832699539931,
-1.33071091181399));
#60245=CARTESIAN_POINT('Ctrl Pts',(-16.9837053427996,1.34211025800256,-0.373011740559811));
#60246=CARTESIAN_POINT('Ctrl Pts',(-16.9041617155825,1.03941832680352,0.927365755856943));
#60247=CARTESIAN_POINT('Ctrl Pts',(-16.8246180883655,-0.218166152382787,
1.37579112992694));
#60248=CARTESIAN_POINT('Ctrl Pts',(-16.7606084782593,-1.06887386894006,
0.719560757628652));
#60249=CARTESIAN_POINT('Ctrl Pts',(-16.7231134105587,-1.17670132186795,
0.163598508604886));
#60250=CARTESIAN_POINT('Ctrl Pts',(-16.7121328852639,-1.17603382108715,
0.000536316405655504));
#60251=CARTESIAN_POINT('Origin',(-35.5608671147362,0.,0.));
#60252=CARTESIAN_POINT('',(-17.8108671147362,-1.17582304073982,-0.000175995329426161));
#60253=CARTESIAN_POINT('',(-17.7121328852639,-1.17863596349438,-0.000939971812119189));
#60254=CARTESIAN_POINT('',(-35.5608671147362,-1.17775,1.38253677383905E-12));
#60255=CARTESIAN_POINT('Ctrl Pts',(-17.8108671147362,-1.17582304073982,
-0.000175995329426085));
#60256=CARTESIAN_POINT('Ctrl Pts',(-17.7983284198186,-1.17607064606856,
-0.186460535126324));
#60257=CARTESIAN_POINT('Ctrl Pts',(-17.7592751824953,-1.0463971061925,-0.766339799844726));
#60258=CARTESIAN_POINT('Ctrl Pts',(-17.6937074027663,-0.137020144008901,
-1.38622624926336));
#60259=CARTESIAN_POINT('Ctrl Pts',(-17.6141637755493,1.09206919009568,-0.864744250084811));
#60260=CARTESIAN_POINT('Ctrl Pts',(-17.5346201483322,1.31789669533126,0.451160763415784));
#60261=CARTESIAN_POINT('Ctrl Pts',(-17.4550765211151,0.332999220126171,
1.35259352852449));
#60262=CARTESIAN_POINT('Ctrl Pts',(-17.3804921765831,-0.877339701365798,
1.0326967032482));
#60263=CARTESIAN_POINT('Ctrl Pts',(-17.3324223744568,-1.17537830032499,
0.317515781186765));
#60264=CARTESIAN_POINT('Ctrl Pts',(-17.3108671147362,-1.17829670657796,
-0.00102595198748913));
#60265=CARTESIAN_POINT('Ctrl Pts',(-17.7121328852639,-1.17863596349438,
-0.000939971812119285));
#60266=CARTESIAN_POINT('Ctrl Pts',(-17.7079545860936,-1.17917341164053,
-0.062640541617889));
#60267=CARTESIAN_POINT('Ctrl Pts',(-17.6772617445177,-1.14666849415385,
-0.515311458828749));
#60268=CARTESIAN_POINT('Ctrl Pts',(-17.6200543605361,-0.559982925362541,
-1.27546729732031));
#60269=CARTESIAN_POINT('Ctrl Pts',(-17.540510733319,0.770215091108087,-1.16067498321473));
#60270=CARTESIAN_POINT('Ctrl Pts',(-17.460967106102,1.39283211551731,0.0204059112696104));
#60271=CARTESIAN_POINT('Ctrl Pts',(-17.3814234788849,0.735882507890194,
1.18274030869519));
#60272=CARTESIAN_POINT('Ctrl Pts',(-17.3018798516679,-0.597107443512156,
1.25851515848381));
#60273=CARTESIAN_POINT('Ctrl Pts',(-17.2454496537941,-1.15360800458277,
0.492054691869927));
#60274=CARTESIAN_POINT('Ctrl Pts',(-17.2155339983262,-1.17934677368052,
0.0510092187330667));
#60275=CARTESIAN_POINT('Ctrl Pts',(-17.2121328852639,-1.17894908727537,
0.000820014261101471));
#60276=CARTESIAN_POINT('Origin',(-35.5608671147362,0.,0.));
#60277=CARTESIAN_POINT('',(-18.3108671147362,-1.17764870709862,0.00108847900253356));
#60278=CARTESIAN_POINT('',(-18.2121328852639,-1.17590200433377,-0.000362038225872191));
#60279=CARTESIAN_POINT('',(-35.5608671147362,-1.17775,1.38253677383905E-12));
#60280=CARTESIAN_POINT('Ctrl Pts',(-18.3108671147362,-1.17764870709862,
0.00108847900253358));
#60281=CARTESIAN_POINT('Ctrl Pts',(-18.290749007586,-1.17491403845395,-0.296634920545634));
#60282=CARTESIAN_POINT('Ctrl Pts',(-18.2441163580302,-0.909022050445814,
-0.991088850735009));
#60283=CARTESIAN_POINT('Ctrl Pts',(-18.1709691660687,0.259263770380752,
-1.36864167384269));
#60284=CARTESIAN_POINT('Ctrl Pts',(-18.0914255388516,1.29153123683166,-0.521866648004122));
#60285=CARTESIAN_POINT('Ctrl Pts',(-18.0118819116345,1.13729513514176,0.804336689200407));
#60286=CARTESIAN_POINT('Ctrl Pts',(-17.9323382844175,-0.0617509544081363,
1.39161221381557));
#60287=CARTESIAN_POINT('Ctrl Pts',(-17.865333352118,-1.02400096068858,0.809393021075806));
#60288=CARTESIAN_POINT('Ctrl Pts',(-17.8248429622243,-1.17554705553286,
0.207459993479165));
#60289=CARTESIAN_POINT('Ctrl Pts',(-17.8108671147362,-1.17582304073982,
-0.000175995329426085));
#60290=CARTESIAN_POINT('Ctrl Pts',(-18.2121328852639,-1.17590200433377,
-0.00036203822587207));
#60291=CARTESIAN_POINT('Ctrl Pts',(-18.2003751738611,-1.17638141866479,
-0.175014423114699));
#60292=CARTESIAN_POINT('Ctrl Pts',(-18.1621029200526,-1.05789358902536,
-0.742902875494098));
#60293=CARTESIAN_POINT('Ctrl Pts',(-18.0973161238384,-0.177768669061831,
-1.38159183680678));
#60294=CARTESIAN_POINT('Ctrl Pts',(-18.0177724966214,1.06613942872675,-0.896517942790525));
#60295=CARTESIAN_POINT('Ctrl Pts',(-17.9382288694043,1.33060684382376,0.412168812988731));
#60296=CARTESIAN_POINT('Ctrl Pts',(-17.8586852421873,0.372672722692757,
1.34220443487269));
#60297=CARTESIAN_POINT('Ctrl Pts',(-17.7833199141404,-0.85932554870962,
1.05510122363174));
#60298=CARTESIAN_POINT('Ctrl Pts',(-17.7344691284993,-1.17576288714689,
0.328897332505749));
#60299=CARTESIAN_POINT('Ctrl Pts',(-17.7121328852639,-1.17863596349438,
-0.000939971812119285));
#60300=CARTESIAN_POINT('Origin',(-35.5608671147362,0.,0.));
#60301=CARTESIAN_POINT('',(-18.8108671147362,-1.17959109088123,-0.000322554745341552));
#60302=CARTESIAN_POINT('',(-18.7121328852639,-1.17730404743425,0.00107034009675953));
#60303=CARTESIAN_POINT('',(-35.5608671147362,-1.17775,1.38253677383905E-12));
#60304=CARTESIAN_POINT('Ctrl Pts',(-18.8108671147362,-1.17959109088123,
-0.000322554745341669));
#60305=CARTESIAN_POINT('Ctrl Pts',(-18.8096841377592,-1.17965442875519,
-0.0177543430943377));
#60306=CARTESIAN_POINT('Ctrl Pts',(-18.7819866183765,-1.17139367616527,
-0.425830504643864));
#60307=CARTESIAN_POINT('Ctrl Pts',(-18.7277745565881,-0.700137645459773,
-1.20424458122967));
#60308=CARTESIAN_POINT('Ctrl Pts',(-18.648230929371,0.63452354392386,-1.24007161334226));
#60309=CARTESIAN_POINT('Ctrl Pts',(-18.5686873021539,1.38626081519776,-0.136669990335221));
#60310=CARTESIAN_POINT('Ctrl Pts',(-18.4891436749369,0.864468374839663,
1.09228758251344));
#60311=CARTESIAN_POINT('Ctrl Pts',(-18.4096000477198,-0.451493638844702,
1.31778269380568));
#60312=CARTESIAN_POINT('Ctrl Pts',(-18.3501745276529,-1.12475091080895,
0.581814575175766));
#60313=CARTESIAN_POINT('Ctrl Pts',(-18.3172635499917,-1.17851817910214,
0.0957479037213191));
#60314=CARTESIAN_POINT('Ctrl Pts',(-18.3108671147362,-1.17764870709862,
0.00108847900253358));
#60315=CARTESIAN_POINT('Ctrl Pts',(-18.7121328852639,-1.17730404743425,
0.00107034009675942));
#60316=CARTESIAN_POINT('Ctrl Pts',(-18.6927957616285,-1.1747817166967,-0.285308750994182));
#60317=CARTESIAN_POINT('Ctrl Pts',(-18.6469440955875,-0.925454311140779,
-0.968295937334803));
#60318=CARTESIAN_POINT('Ctrl Pts',(-18.5745778871408,0.21886115147667,-1.37568074043561));
#60319=CARTESIAN_POINT('Ctrl Pts',(-18.4950342599237,1.27560870369364,-0.55966073499237));
#60320=CARTESIAN_POINT('Ctrl Pts',(-18.4154906327066,1.16048039621642,0.770508243452683));
#60321=CARTESIAN_POINT('Ctrl Pts',(-18.3359470054896,-0.0207577285084573,
1.39282691671949));
#60322=CARTESIAN_POINT('Ctrl Pts',(-18.2681610896753,-1.01114065994669,
0.832733888360385));
#60323=CARTESIAN_POINT('Ctrl Pts',(-18.2268897162668,-1.17530030252116,
0.21884012108592));
#60324=CARTESIAN_POINT('Ctrl Pts',(-18.2121328852639,-1.17590200433377,
-0.00036203822587207));
#60325=CARTESIAN_POINT('Origin',(-35.5608671147362,0.,0.));
#60326=CARTESIAN_POINT('',(-19.3108671147362,-1.17666978654916,-0.000928285457528838));
#60327=CARTESIAN_POINT('',(-19.2121328852639,-1.17968463629076,-0.000111381752591205));
#60328=CARTESIAN_POINT('',(-35.5608671147362,-1.17775,1.38253677383905E-12));
#60329=CARTESIAN_POINT('Ctrl Pts',(-19.3108671147362,-1.17666978654916,
-0.000928285457529009));
#60330=CARTESIAN_POINT('Ctrl Pts',(-19.3021047255266,-1.17762313276549,
-0.130874534662354));
#60331=CARTESIAN_POINT('Ctrl Pts',(-19.2668277939114,-1.09776245886893,
-0.652892723031988));
#60332=CARTESIAN_POINT('Ctrl Pts',(-19.2050363198904,-0.332315869745427,
-1.35276158162712));
#60333=CARTESIAN_POINT('Ctrl Pts',(-19.1254926926734,0.958328722255644,
-1.0109420330122));
#60334=CARTESIAN_POINT('Ctrl Pts',(-19.0459490654563,1.36857614229396,0.25960946969393));
#60335=CARTESIAN_POINT('Ctrl Pts',(-18.9664054382392,0.521540401231442,
1.29166301483565));
#60336=CARTESIAN_POINT('Ctrl Pts',(-18.8880447879992,-0.78490114965271,
1.13939071929856));
#60337=CARTESIAN_POINT('Ctrl Pts',(-18.8361986801649,-1.1782348113175,0.372951393674192));
#60338=CARTESIAN_POINT('Ctrl Pts',(-18.8108671147362,-1.17959109088123,
-0.000322554745341669));
#60339=CARTESIAN_POINT('Ctrl Pts',(-19.2121328852639,-1.17968463629076,
-0.000111381752591032));
#60340=CARTESIAN_POINT('Ctrl Pts',(-19.2117308918017,-1.17969259990424,
-0.00603370807851372));
#60341=CARTESIAN_POINT('Ctrl Pts',(-19.1848143559338,-1.17696574873875,
-0.402571200060254));
#60342=CARTESIAN_POINT('Ctrl Pts',(-19.1313832776602,-0.735284913137964,
-1.18311191344811));
#60343=CARTESIAN_POINT('Ctrl Pts',(-19.0518396504431,0.597743148369296,
-1.25821334908223));
#60344=CARTESIAN_POINT('Ctrl Pts',(-18.9722960232261,1.38163669562993,-0.177419684702549));
#60345=CARTESIAN_POINT('Ctrl Pts',(-18.892752396009,0.896248616175358,1.06636584774406));
#60346=CARTESIAN_POINT('Ctrl Pts',(-18.813208768792,-0.412504900140071,
1.33050269093737));
#60347=CARTESIAN_POINT('Ctrl Pts',(-18.7530022652102,-1.1162649024249,0.605265384768711));
#60348=CARTESIAN_POINT('Ctrl Pts',(-18.7193103040342,-1.17824026857666,
0.107366535052814));
#60349=CARTESIAN_POINT('Ctrl Pts',(-18.7121328852639,-1.17730404743425,
0.00107034009675942));
#60350=CARTESIAN_POINT('Origin',(-35.5608671147362,0.,0.));
#60351=CARTESIAN_POINT('',(-19.8108671147362,-1.17622381119946,0.000700251168187343));
#60352=CARTESIAN_POINT('',(-19.7121328852639,-1.17696832030681,-0.00101504787385631));
#60353=CARTESIAN_POINT('',(-35.5608671147362,-1.17775,1.38253677383905E-12));
#60354=CARTESIAN_POINT('Ctrl Pts',(-19.8108671147362,-1.17622381119946,
0.000700251168187383));
#60355=CARTESIAN_POINT('Ctrl Pts',(-19.7945253132941,-1.17491434676118,
-0.2418795226269));
#60356=CARTESIAN_POINT('Ctrl Pts',(-19.7516689694463,-0.983506135042355,
-0.879939628894577));
#60357=CARTESIAN_POINT('Ctrl Pts',(-19.6822980831928,0.0624539660114313,
-1.3915808406774));
#60358=CARTESIAN_POINT('Ctrl Pts',(-19.6027544559757,1.20442139179994,-0.699833440888375));
#60359=CARTESIAN_POINT('Ctrl Pts',(-19.5232108287587,1.23991129837533,0.634836755530266));
#60360=CARTESIAN_POINT('Ctrl Pts',(-19.4436672015416,0.13631982794163,1.38629529268513));
#60361=CARTESIAN_POINT('Ctrl Pts',(-19.3728859635341,-0.95714057527515,
0.921706396515711));
#60362=CARTESIAN_POINT('Ctrl Pts',(-19.3286192679323,-1.17473835578566,
0.262336181341884));
#60363=CARTESIAN_POINT('Ctrl Pts',(-19.3108671147362,-1.17666978654916,
-0.000928285457529009));
#60364=CARTESIAN_POINT('Ctrl Pts',(-19.7121328852639,-1.17696832030681,
-0.00101504787385635));
#60365=CARTESIAN_POINT('Ctrl Pts',(-19.7041514795691,-1.17793465627579,
-0.119303575573876));
#60366=CARTESIAN_POINT('Ctrl Pts',(-19.6696555314687,-1.10709672596639,
-0.629420301679817));
#60367=CARTESIAN_POINT('Ctrl Pts',(-19.6086450409626,-0.371994615647838,
-1.3423925316986));
#60368=CARTESIAN_POINT('Ctrl Pts',(-19.5291014137455,0.928153134988703,
-1.03871529364008));
#60369=CARTESIAN_POINT('Ctrl Pts',(-19.4495577865284,1.37562541403019,0.219208630088832));
#60370=CARTESIAN_POINT('Ctrl Pts',(-19.3700141593114,0.55933850891441,1.27575002867982));
#60371=CARTESIAN_POINT('Ctrl Pts',(-19.2908725255565,-0.764079154747326,
1.16086926264095));
#60372=CARTESIAN_POINT('Ctrl Pts',(-19.2382454342073,-1.17916733870663,
0.384588994216886));
#60373=CARTESIAN_POINT('Ctrl Pts',(-19.2121328852639,-1.17968463629076,
-0.000111381752591032));
#60374=CARTESIAN_POINT('Origin',(-35.5608671147362,0.,0.));
#60375=CARTESIAN_POINT('',(-20.3108671147362,-1.17923477537134,0.000662329376658134));
#60376=CARTESIAN_POINT('',(-20.2121328852639,-1.17603928037595,0.000542067565237406));
#60377=CARTESIAN_POINT('',(-35.5608671147362,-1.17775,1.38253677383905E-12));
#60378=CARTESIAN_POINT('Ctrl Pts',(-20.3108671147362,-1.17923477537134,
0.000662329376658151));
#60379=CARTESIAN_POINT('Ctrl Pts',(-20.2869459010615,-1.17686247573691,
-0.35211161007433));
#60380=CARTESIAN_POINT('Ctrl Pts',(-20.2365101449812,-0.821008972712208,
-1.10005420902622));
#60381=CARTESIAN_POINT('Ctrl Pts',(-20.1595598464952,0.452159303261918,
-1.31755443852794));
#60382=CARTESIAN_POINT('Ctrl Pts',(-20.0800162192781,1.35284547871658,-0.331974162740232));
#60383=CARTESIAN_POINT('Ctrl Pts',(-20.0004725920611,1.01069993484086,0.958584047292498));
#60384=CARTESIAN_POINT('Ctrl Pts',(-19.920928964844,-0.259955152443364,
1.36851052342652));
#60385=CARTESIAN_POINT('Ctrl Pts',(-19.857727139069,-1.07980893901382,0.695286514566635));
#60386=CARTESIAN_POINT('Ctrl Pts',(-19.8210398556998,-1.17703895037361,
0.151705708587368));
#60387=CARTESIAN_POINT('Ctrl Pts',(-19.8108671147362,-1.17622381119946,
0.000700251168187383));
#60388=CARTESIAN_POINT('Ctrl Pts',(-20.2121328852639,-1.17603928037595,
0.000542067565237423));
#60389=CARTESIAN_POINT('Ctrl Pts',(-20.1965720673366,-1.17508294569432,
-0.230535369896458));
#60390=CARTESIAN_POINT('Ctrl Pts',(-20.1544967070036,-0.997382817803285,
-0.856709931464427));
#60391=CARTESIAN_POINT('Ctrl Pts',(-20.0859068042649,0.0214613589905084,
-1.39281625252631));
#60392=CARTESIAN_POINT('Ctrl Pts',(-20.0063631770478,1.1832976026021,-0.734986045382691));
#60393=CARTESIAN_POINT('Ctrl Pts',(-19.9268195498308,1.25806232396071,0.598060943601679));
#60394=CARTESIAN_POINT('Ctrl Pts',(-19.8472759226137,0.177070689023417,
1.38168146630109));
#60395=CARTESIAN_POINT('Ctrl Pts',(-19.7757137010914,-0.941803093652268,
0.94471458317044));
#60396=CARTESIAN_POINT('Ctrl Pts',(-19.7306660219748,-1.17472445032866,
0.27365554763835));
#60397=CARTESIAN_POINT('Ctrl Pts',(-19.7121328852639,-1.17696832030681,
-0.00101504787385635));
#60398=CARTESIAN_POINT('Origin',(-35.5608671147362,0.,0.));
#60399=CARTESIAN_POINT('',(-20.8108671147362,-1.17828477702325,-0.00102826220839124));
#60400=CARTESIAN_POINT('',(-20.7121328852639,-1.17895929484358,0.00081529925158268));
#60401=CARTESIAN_POINT('',(-35.5608671147362,-1.17775,1.38253677383905E-12));
#60402=CARTESIAN_POINT('Ctrl Pts',(-20.8108671147362,-1.17828477702325,
-0.00102826220839125));
#60403=CARTESIAN_POINT('Ctrl Pts',(-20.8058810312347,-1.17896058675312,
-0.0747140894821463));
#60404=CARTESIAN_POINT('Ctrl Pts',(-20.7743804053275,-1.13905376627765,
-0.539509952836493));
#60405=CARTESIAN_POINT('Ctrl Pts',(-20.7163652370146,-0.520887807880025,
-1.29192632360089));
#60406=CARTESIAN_POINT('Ctrl Pts',(-20.6368216097975,0.80519827226939,-1.13668530224745));
#60407=CARTESIAN_POINT('Ctrl Pts',(-20.5572779825804,1.39156502092812,0.06280546584721));
#60408=CARTESIAN_POINT('Ctrl Pts',(-20.4777343553634,0.699529191665802,
1.20459812552501));
#60409=CARTESIAN_POINT('Ctrl Pts',(-20.3981907281463,-0.635149926632454,
1.23975090429883));
#60410=CARTESIAN_POINT('Ctrl Pts',(-20.3425683146039,-1.16042683999627,
0.467910605410006));
#60411=CARTESIAN_POINT('Ctrl Pts',(-20.3134604434672,-1.17949195934555,
0.0389069939316387));
#60412=CARTESIAN_POINT('Ctrl Pts',(-20.3108671147362,-1.17923477537134,
0.000662329376658151));
#60413=CARTESIAN_POINT('Ctrl Pts',(-20.7121328852639,-1.17895929484358,
0.000815299251582628));
#60414=CARTESIAN_POINT('Ctrl Pts',(-20.688992655104,-1.17626502045395,-0.340650404120654));
#60415=CARTESIAN_POINT('Ctrl Pts',(-20.6393378825385,-0.84018563607975,
-1.07799535577281));
#60416=CARTESIAN_POINT('Ctrl Pts',(-20.5631685675673,0.413176995464697,
-1.3302941305027));
#60417=CARTESIAN_POINT('Ctrl Pts',(-20.4836249403502,1.34248645164237,-0.371655526513227));
#60418=CARTESIAN_POINT('Ctrl Pts',(-20.4040813131332,1.03848081668687,0.928415476284475));
#60419=CARTESIAN_POINT('Ctrl Pts',(-20.3245376859161,-0.219556094714919,
1.37556999985631));
#60420=CARTESIAN_POINT('Ctrl Pts',(-20.2605548766263,-1.06924443023848,
0.718755558999398));
#60421=CARTESIAN_POINT('Ctrl Pts',(-20.2230866097423,-1.17671247292024,
0.163204377153041));
#60422=CARTESIAN_POINT('Ctrl Pts',(-20.2121328852639,-1.17603928037595,
0.000542067565237423));
#60423=CARTESIAN_POINT('Origin',(-35.5608671147362,0.,0.));
#60424=CARTESIAN_POINT('',(-21.3108671147362,-1.17582130790704,-0.000169484100476859));
#60425=CARTESIAN_POINT('',(-21.2121328852639,-1.17862465731635,-0.000943510414042614));
#60426=CARTESIAN_POINT('',(-35.5608671147362,-1.17775,1.38253677383905E-12));
#60427=CARTESIAN_POINT('Ctrl Pts',(-21.3108671147362,-1.17582130790704,
-0.000169484100476808));
#60428=CARTESIAN_POINT('Ctrl Pts',(-21.2983016190021,-1.17606024285316,
-0.186852883416342));
#60429=CARTESIAN_POINT('Ctrl Pts',(-21.2592215808624,-1.04599425125585,
-0.767143650822197));
#60430=CARTESIAN_POINT('Ctrl Pts',(-21.1936270003169,-0.135619477084131,
-1.38636398230999));
#60431=CARTESIAN_POINT('Ctrl Pts',(-21.1140833730999,1.09294234156633,-0.863640418242735));
#60432=CARTESIAN_POINT('Ctrl Pts',(-21.0345397458828,1.31744018479035,0.452492092207748));
#60433=CARTESIAN_POINT('Ctrl Pts',(-20.9549961186657,0.331632434554235,
1.352929289491));
#60434=CARTESIAN_POINT('Ctrl Pts',(-20.8804385749502,-0.877947854422183,
1.03192513093976));
#60435=CARTESIAN_POINT('Ctrl Pts',(-20.8323955736404,-1.17536682709477,
0.317125716520315));
#60436=CARTESIAN_POINT('Ctrl Pts',(-20.8108671147362,-1.17828477702325,
-0.00102826220839125));
#60437=CARTESIAN_POINT('Ctrl Pts',(-21.2121328852639,-1.17862465731635,
-0.00094351041404258));
#60438=CARTESIAN_POINT('Ctrl Pts',(-21.2079277852772,-1.17916686958785,
-0.0630413912822054));
#60439=CARTESIAN_POINT('Ctrl Pts',(-21.1772081428848,-1.14642246849581,
-0.516113907661345));
#60440=CARTESIAN_POINT('Ctrl Pts',(-21.1199739580867,-0.558693949717291,
-1.27603243445472));
#60441=CARTESIAN_POINT('Ctrl Pts',(-21.0404303308696,0.771387405449101,
-1.15989619102127));
#60442=CARTESIAN_POINT('Ctrl Pts',(-20.9608867036526,1.39281078713163,0.0218131721888098));
#60443=CARTESIAN_POINT('Ctrl Pts',(-20.8813430764355,0.734687130733419,
1.18348321625862));
#60444=CARTESIAN_POINT('Ctrl Pts',(-20.8017994492184,-0.598378700676205,
1.25791121857157));
#60445=CARTESIAN_POINT('Ctrl Pts',(-20.7453960521612,-1.15384063643505,
0.491253161147155));
#60446=CARTESIAN_POINT('Ctrl Pts',(-20.7155071975097,-1.17935217438729,
0.050607885430154));
#60447=CARTESIAN_POINT('Ctrl Pts',(-20.7121328852639,-1.17895929484358,
0.000815299251582628));
#60448=CARTESIAN_POINT('Origin',(-35.5608671147362,0.,0.));
#60449=CARTESIAN_POINT('',(-21.8108671147362,-1.17766074088617,0.00108845803827099));
#60450=CARTESIAN_POINT('',(-21.7121328852638,-1.17589839182392,-0.00035580353738629));
#60451=CARTESIAN_POINT('',(-35.5608671147362,-1.17775,1.38253677383905E-12));
#60452=CARTESIAN_POINT('Ctrl Pts',(-21.8108671147362,-1.17766074088617,
0.00108845803827095));
#60453=CARTESIAN_POINT('Ctrl Pts',(-21.7907222067696,-1.17492000502449,
-0.297023786339216));
#60454=CARTESIAN_POINT('Ctrl Pts',(-21.7440627563973,-0.908448417634372,
-0.991868889400734));
#60455=CARTESIAN_POINT('Ctrl Pts',(-21.6708887636193,0.260646468162729,
-1.36837902375229));
#60456=CARTESIAN_POINT('Ctrl Pts',(-21.5913451364022,1.29205785434534,-0.520561461342927));
#60457=CARTESIAN_POINT('Ctrl Pts',(-21.5118015091852,1.13648187955178,0.805485363902682));
#60458=CARTESIAN_POINT('Ctrl Pts',(-21.4322578819681,-0.0631569616758272,
1.3915491123934));
#60459=CARTESIAN_POINT('Ctrl Pts',(-21.3652797504851,-1.02443357395186,
0.808591257748514));
#60460=CARTESIAN_POINT('Ctrl Pts',(-21.3248161614078,-1.17555606451471,
0.207069092473432));
#60461=CARTESIAN_POINT('Ctrl Pts',(-21.3108671147362,-1.17582130790704,
-0.000169484100476808));
#60462=CARTESIAN_POINT('Ctrl Pts',(-21.7121328852638,-1.17589839182392,
-0.000355803537386394));
#60463=CARTESIAN_POINT('Ctrl Pts',(-21.7003483730446,-1.17637054255772,
-0.175407637251437));
#60464=CARTESIAN_POINT('Ctrl Pts',(-21.6620493184196,-1.05750679897208,
-0.743707513842047));
#60465=CARTESIAN_POINT('Ctrl Pts',(-21.5972357213891,-0.176372663794721,
-1.38177074317598));
#60466=CARTESIAN_POINT('Ctrl Pts',(-21.517692094172,1.06704469651685,-0.895440293300685));
#60467=CARTESIAN_POINT('Ctrl Pts',(-21.4381484669549,1.33018972296772,0.413513003595081));
#60468=CARTESIAN_POINT('Ctrl Pts',(-21.3586048397379,0.371316413666049,
1.34258028593203));
#60469=CARTESIAN_POINT('Ctrl Pts',(-21.2832663125075,-0.859953139331574,
1.05433499103261));
#60470=CARTESIAN_POINT('Ctrl Pts',(-21.2344423276828,-1.17574804237543,
0.328506229651944));
#60471=CARTESIAN_POINT('Ctrl Pts',(-21.2121328852639,-1.17862465731635,
-0.00094351041404258));
#60472=CARTESIAN_POINT('Origin',(-35.5608671147362,0.,0.));
#60473=CARTESIAN_POINT('',(-22.3108671147362,-1.17958641441151,-0.000329593618060359));
#60474=CARTESIAN_POINT('',(-22.2121328852638,-1.17731562723721,0.00107155510022959));
#60475=CARTESIAN_POINT('',(-35.5608671147362,-1.17775,1.38253677383905E-12));
#60476=CARTESIAN_POINT('Ctrl Pts',(-22.3108671147362,-1.17958641441151,
-0.000329593618060599));
#60477=CARTESIAN_POINT('Ctrl Pts',(-22.3096573369427,-1.17965245508073,
-0.0181564948118189));
#60478=CARTESIAN_POINT('Ctrl Pts',(-22.2819330167435,-1.17119619678948,
-0.426629235604552));
#60479=CARTESIAN_POINT('Ctrl Pts',(-22.2276941541387,-0.69892055934474,
-1.20495136239444));
#60480=CARTESIAN_POINT('Ctrl Pts',(-22.1481505269216,0.635776147244211,
-1.23942987885813));
#60481=CARTESIAN_POINT('Ctrl Pts',(-22.0686068997046,1.38639819444309,-0.135269288664905));
#60482=CARTESIAN_POINT('Ctrl Pts',(-21.9890632724875,0.863364322481949,
1.09316045513743));
#60483=CARTESIAN_POINT('Ctrl Pts',(-21.9095196452704,-0.4528248522834,1.31732584699667));
#60484=CARTESIAN_POINT('Ctrl Pts',(-21.85012092602,-1.12503488038791,0.581010094305927));
#60485=CARTESIAN_POINT('Ctrl Pts',(-21.8172367491753,-1.1785273363336,0.095348805201107));
#60486=CARTESIAN_POINT('Ctrl Pts',(-21.8108671147362,-1.17766074088617,
0.00108845803827095));
#60487=CARTESIAN_POINT('Ctrl Pts',(-22.2121328852638,-1.17731562723721,
0.00107155510022956));
#60488=CARTESIAN_POINT('Ctrl Pts',(-22.192768960812,-1.17478496411128,-0.285697287951891));
#60489=CARTESIAN_POINT('Ctrl Pts',(-22.1468904939546,-0.92489945401143,
-0.969080044767785));
#60490=CARTESIAN_POINT('Ctrl Pts',(-22.0744974846914,0.220250981920178,
-1.37545890821731));
#60491=CARTESIAN_POINT('Ctrl Pts',(-21.9949538574744,1.27617351522542,-0.558371616639268));
#60492=CARTESIAN_POINT('Ctrl Pts',(-21.9154102302573,1.15970130793088,0.771680361039824));
#60493=CARTESIAN_POINT('Ctrl Pts',(-21.8358666030402,-0.0221649839953902,
1.39280523287201));
#60494=CARTESIAN_POINT('Ctrl Pts',(-21.7681074880424,-1.01159016239307,
0.831933682326423));
#60495=CARTESIAN_POINT('Ctrl Pts',(-21.7268629154503,-1.17530822785005,
0.218449926120964));
#60496=CARTESIAN_POINT('Ctrl Pts',(-21.7121328852638,-1.17589839182392,
-0.000355803537386394));
#60497=CARTESIAN_POINT('Origin',(-35.5608671147362,0.,0.));
#60498=CARTESIAN_POINT('',(-22.8108671147362,-1.17666012157462,-0.000924768044772844));
#60499=CARTESIAN_POINT('',(-22.7121328852638,-1.17968287648054,-0.000118772304556619));
#60500=CARTESIAN_POINT('',(-35.5608671147362,-1.17775,1.38253677383905E-12));
#60501=CARTESIAN_POINT('Ctrl Pts',(-22.8108671147362,-1.17666012157462,
-0.000924768044772949));
#60502=CARTESIAN_POINT('Ctrl Pts',(-22.8020779247101,-1.17761224020395,
-0.131271169296472));
#60503=CARTESIAN_POINT('Ctrl Pts',(-22.7667741922784,-1.09743454109949,
-0.653698313999505));
#60504=CARTESIAN_POINT('Ctrl Pts',(-22.7049559174411,-0.330948914727013,
-1.35309665207331));
#60505=CARTESIAN_POINT('Ctrl Pts',(-22.625412290224,0.959349655377068,-1.00997325347698));
#60506=CARTESIAN_POINT('Ctrl Pts',(-22.5458686630069,1.36831314295389,0.260992101088554));
#60507=CARTESIAN_POINT('Ctrl Pts',(-22.4663250357899,0.520235081592649,
1.29218930265316));
#60508=CARTESIAN_POINT('Ctrl Pts',(-22.3879911863663,-0.785605176845554,
1.13864963108566));
#60509=CARTESIAN_POINT('Ctrl Pts',(-22.3361718793484,-1.17820505033083,
0.372553377872414));
#60510=CARTESIAN_POINT('Ctrl Pts',(-22.3108671147362,-1.17958641441151,
-0.000329593618060599));
#60511=CARTESIAN_POINT('Ctrl Pts',(-22.7121328852638,-1.17968287648054,
-0.000118772304556725));
#60512=CARTESIAN_POINT('Ctrl Pts',(-22.7117040909852,-1.17969191172516,
-0.00643596420863167));
#60513=CARTESIAN_POINT('Ctrl Pts',(-22.6847607543009,-1.17678034422692,
-0.403368869626029));
#60514=CARTESIAN_POINT('Ctrl Pts',(-22.6313028752108,-0.734089160829106,
-1.18385421703197));
#60515=CARTESIAN_POINT('Ctrl Pts',(-22.5517592479938,0.59901410027068,-1.25760876702895));
#60516=CARTESIAN_POINT('Ctrl Pts',(-22.4722156207767,1.38181524937403,-0.176023634289684));
#60517=CARTESIAN_POINT('Ctrl Pts',(-22.3926719935596,0.89517073805671,1.06727084329994));
#60518=CARTESIAN_POINT('Ctrl Pts',(-22.3131283663426,-0.413848985342271,
1.33008523056319));
#60519=CARTESIAN_POINT('Ctrl Pts',(-22.2529486635773,-1.11656292156274,
0.604460393264336));
#60520=CARTESIAN_POINT('Ctrl Pts',(-22.2192835032177,-1.17825013848407,
0.106968189992137));
#60521=CARTESIAN_POINT('Ctrl Pts',(-22.2121328852638,-1.17731562723721,
0.00107155510022956));
#60522=CARTESIAN_POINT('Origin',(-35.5608671147362,0.,0.));
#60523=CARTESIAN_POINT('',(-23.3108671147362,-1.17623098844965,0.000705324900118179));
#60524=CARTESIAN_POINT('',(-23.2121328852638,-1.17695757629942,-0.00101259305823678));
#60525=CARTESIAN_POINT('',(-35.5608671147362,-1.17775,1.38253677383905E-12));
#60526=CARTESIAN_POINT('Ctrl Pts',(-23.3108671147362,-1.17623098844965,
0.000705324900118123));
#60527=CARTESIAN_POINT('Ctrl Pts',(-23.2944985124776,-1.17490938811235,
-0.242268570117102));
#60528=CARTESIAN_POINT('Ctrl Pts',(-23.2516153678133,-0.983020868014358,
-0.880735622124971));
#60529=CARTESIAN_POINT('Ctrl Pts',(-23.1822176807434,0.063859941221911,
-1.39151702897166));
#60530=CARTESIAN_POINT('Ctrl Pts',(-23.1026740535264,1.20512786551627,-0.698616176285083));
#60531=CARTESIAN_POINT('Ctrl Pts',(-23.0231304263093,1.23926924751441,0.636089196713827));
#60532=CARTESIAN_POINT('Ctrl Pts',(-22.9435867990922,0.134919091615136,
1.38643231812041));
#60533=CARTESIAN_POINT('Ctrl Pts',(-22.8728323619012,-0.957657495158324,
0.920915194534099));
#60534=CARTESIAN_POINT('Ctrl Pts',(-22.8285924671158,-1.17473996304328,
0.261947679446613));
#60535=CARTESIAN_POINT('Ctrl Pts',(-22.8108671147362,-1.17666012157462,
-0.000924768044772949));
#60536=CARTESIAN_POINT('Ctrl Pts',(-23.2121328852638,-1.17695757629942,
-0.00101259305823675));
#60537=CARTESIAN_POINT('Ctrl Pts',(-23.2041246787526,-1.17792417914125,
-0.119701061165631));
#60538=CARTESIAN_POINT('Ctrl Pts',(-23.1696019298358,-1.10678344897941,
-0.630225684678308));
#60539=CARTESIAN_POINT('Ctrl Pts',(-23.1085646385132,-0.370638116920458,
-1.34276769752508));
#60540=CARTESIAN_POINT('Ctrl Pts',(-23.0290210112962,0.929202144692953,
-1.03777698834055));
#60541=CARTESIAN_POINT('Ctrl Pts',(-22.949477384079,1.37540323075928,0.220598404455005));
#60542=CARTESIAN_POINT('Ctrl Pts',(-22.869933756862,0.558049247935703,1.27631451457294));
#60543=CARTESIAN_POINT('Ctrl Pts',(-22.7908189239236,-0.764803540982205,
1.16013602633681));
#60544=CARTESIAN_POINT('Ctrl Pts',(-22.7382186333909,-1.17913321635846,
0.384188307066044));
#60545=CARTESIAN_POINT('Ctrl Pts',(-22.7121328852638,-1.17968287648054,
-0.000118772304556725));
#60546=CARTESIAN_POINT('Origin',(-35.5608671147362,0.,0.));
#60547=CARTESIAN_POINT('',(-23.8108671147362,-1.17924338756027,0.000656574873420682));
#60548=CARTESIAN_POINT('',(-23.7121328852638,-1.17604479913671,0.000547799251428352));
#60549=CARTESIAN_POINT('',(-35.5608671147362,-1.17775,1.38253677383905E-12));
#60550=CARTESIAN_POINT('Ctrl Pts',(-23.8108671147362,-1.17924338756027,
0.000656574873420736));
#60551=CARTESIAN_POINT('Ctrl Pts',(-23.7869191002451,-1.17688497172179,
-0.352505813248667));
#60552=CARTESIAN_POINT('Ctrl Pts',(-23.7364565433482,-0.82034060012706,
-1.10080786323156));
#60553=CARTESIAN_POINT('Ctrl Pts',(-23.6594794440458,0.453490285739293,
-1.31709691927021));
#60554=CARTESIAN_POINT('Ctrl Pts',(-23.5799358168287,1.35318020387053,-0.330607123129397));
#60555=CARTESIAN_POINT('Ctrl Pts',(-23.5003921896117,1.00973089745727,0.959604735675643));
#60556=CARTESIAN_POINT('Ctrl Pts',(-23.4208485623946,-0.261337717362417,
1.36824717485357));
#60557=CARTESIAN_POINT('Ctrl Pts',(-23.3576735374361,-1.08016351082504,
0.694480989205406));
#60558=CARTESIAN_POINT('Ctrl Pts',(-23.3210130548833,-1.17705017127962,
0.151310645819719));
#60559=CARTESIAN_POINT('Ctrl Pts',(-23.3108671147362,-1.17623098844965,
0.000705324900118123));
#60560=CARTESIAN_POINT('Ctrl Pts',(-23.7121328852638,-1.17604479913671,
0.000547799251428352));
#60561=CARTESIAN_POINT('Ctrl Pts',(-23.6965452665201,-1.17507642505556,
-0.23092491432183));
#60562=CARTESIAN_POINT('Ctrl Pts',(-23.6544431053707,-0.996915032030405,
-0.857508140843176));
#60563=CARTESIAN_POINT('Ctrl Pts',(-23.5858264018155,0.0228686033435479,
-1.39279385775939));
#60564=CARTESIAN_POINT('Ctrl Pts',(-23.5062827745985,1.18403960412511,-0.733790105612224));
#60565=CARTESIAN_POINT('Ctrl Pts',(-23.4267391473814,1.25745742089477,0.599331742750071));
#60566=CARTESIAN_POINT('Ctrl Pts',(-23.3471955201644,0.175674593553903,
1.38185966740868));
#60567=CARTESIAN_POINT('Ctrl Pts',(-23.2756600994585,-0.942338256566478,
0.943926606442159));
#60568=CARTESIAN_POINT('Ctrl Pts',(-23.2306392211583,-1.17472383309582,
0.273267129189906));
#60569=CARTESIAN_POINT('Ctrl Pts',(-23.2121328852638,-1.17695757629942,
-0.00101259305823675));
#60570=CARTESIAN_POINT('Origin',(-35.5608671147362,0.,0.));
#60571=CARTESIAN_POINT('',(-24.3108671147362,-1.17827283352878,-0.00103052933429097));
#60572=CARTESIAN_POINT('',(-24.2121328852638,-1.17896945751039,0.000810547160777966));
#60573=CARTESIAN_POINT('',(-35.5608671147362,-1.17775,1.38253677383905E-12));
#60574=CARTESIAN_POINT('Ctrl Pts',(-24.3108671147362,-1.17827283352878,
-0.00103052933429112));
#60575=CARTESIAN_POINT('Ctrl Pts',(-24.3058542304182,-1.17895298703858,
-0.0751143629464088));
#60576=CARTESIAN_POINT('Ctrl Pts',(-24.2743268036945,-1.13879400230303,
-0.540313240337936));
#60577=CARTESIAN_POINT('Ctrl Pts',(-24.2162848345652,-0.519582222535895,
-1.29245195192535));
#60578=CARTESIAN_POINT('Ctrl Pts',(-24.1367412073481,0.806346330376981,
-1.13587117645381));
#60579=CARTESIAN_POINT('Ctrl Pts',(-24.057197580131,1.39150085408669,0.0642114248945288));
#60580=CARTESIAN_POINT('Ctrl Pts',(-23.977653952914,0.698311748651915,1.20530429174781));
#60581=CARTESIAN_POINT('Ctrl Pts',(-23.8981103256969,-0.636402205599313,
1.2391085371021));
#60582=CARTESIAN_POINT('Ctrl Pts',(-23.842514712971,-1.1606462882032,0.467110064893475));
#60583=CARTESIAN_POINT('Ctrl Pts',(-23.8134336426507,-1.17949614087667,
0.038505271174667));
#60584=CARTESIAN_POINT('Ctrl Pts',(-23.8108671147362,-1.17924338756027,
0.000656574873420736));
#60585=CARTESIAN_POINT('Ctrl Pts',(-24.2121328852638,-1.17896945751039,
0.000810547160777922));
#60586=CARTESIAN_POINT('Ctrl Pts',(-24.1889658542875,-1.17628369526718,
-0.341042935736306));
#60587=CARTESIAN_POINT('Ctrl Pts',(-24.1392842809056,-0.83953713219871,
-1.07875537338835));
#60588=CARTESIAN_POINT('Ctrl Pts',(-24.0630881651179,0.4145208696013,-1.32987599117216));
#60589=CARTESIAN_POINT('Ctrl Pts',(-23.9835445379008,1.34286127481651,-0.370298933065331));
#60590=CARTESIAN_POINT('Ctrl Pts',(-23.9040009106838,1.03754224644608,0.929464248947089));
#60591=CARTESIAN_POINT('Ctrl Pts',(-23.8244572834667,-0.220945812915096,
1.37534746554696));
#60592=CARTESIAN_POINT('Ctrl Pts',(-23.7605012749934,-1.06961445595894,
0.71795034584099));
#60593=CARTESIAN_POINT('Ctrl Pts',(-23.7230598089258,-1.17672362954916,
0.162810214865867));
#60594=CARTESIAN_POINT('Ctrl Pts',(-23.7121328852638,-1.17604479913671,
0.000547799251428352));
#60595=CARTESIAN_POINT('Origin',(-35.5608671147362,0.,0.));
#60596=CARTESIAN_POINT('',(-24.8108671147362,-1.17581964054164,-0.000162966847959915));
#60597=CARTESIAN_POINT('',(-24.7121328852638,-1.17861332264333,-0.000947007987461695));
#60598=CARTESIAN_POINT('',(-35.5608671147362,-1.17775,1.38253677383905E-12));
#60599=CARTESIAN_POINT('Ctrl Pts',(-24.8108671147362,-1.17581964054164,
-0.000162966847959863));
#60600=CARTESIAN_POINT('Ctrl Pts',(-24.7982748181856,-1.17604985957002,
-0.187245202631063));
#60601=CARTESIAN_POINT('Ctrl Pts',(-24.7591679792295,-1.04559083977625,
-0.767947470306765));
#60602=CARTESIAN_POINT('Ctrl Pts',(-24.6935465978676,-0.134218671713418,
-1.38650030009895));
#60603=CARTESIAN_POINT('Ctrl Pts',(-24.6140029706505,1.09381437731624,-0.862535704760827));
#60604=CARTESIAN_POINT('Ctrl Pts',(-24.5344593434334,1.31698232935204,0.453822959077054));
#60605=CARTESIAN_POINT('Ctrl Pts',(-24.4549157162164,0.330265310438215,
1.35326366933134));
#60606=CARTESIAN_POINT('Ctrl Pts',(-24.3803849733173,-0.878555344404979,
1.03115338381769));
#60607=CARTESIAN_POINT('Ctrl Pts',(-24.3323687728239,-1.17535546554516,
0.31673568251358));
#60608=CARTESIAN_POINT('Ctrl Pts',(-24.3108671147362,-1.17827283352878,
-0.00103052933429112));
#60609=CARTESIAN_POINT('Ctrl Pts',(-24.7121328852638,-1.17861332264333,
-0.000947007987461626));
#60610=CARTESIAN_POINT('Ctrl Pts',(-24.7079009844607,-1.17916029092104,
-0.063442223242721));
#60611=CARTESIAN_POINT('Ctrl Pts',(-24.6771545412518,-1.14617599158811,
-0.516916385756128));
#60612=CARTESIAN_POINT('Ctrl Pts',(-24.6198935556373,-0.557404403734147,
-1.27659626896248));
#60613=CARTESIAN_POINT('Ctrl Pts',(-24.5403499284203,0.772558932325985,
-1.15911621475782));
#60614=CARTESIAN_POINT('Ctrl Pts',(-24.4608063012032,1.39278803690711,0.0232204108402372));
#60615=CARTESIAN_POINT('Ctrl Pts',(-24.3812626739862,0.733491003577628,
1.18422491567347));
#60616=CARTESIAN_POINT('Ctrl Pts',(-24.3017190467691,-0.599649346990552,
1.25730599453155));
#60617=CARTESIAN_POINT('Ctrl Pts',(-24.2453424505283,-1.15407282652745,
0.490451662275239));
#60618=CARTESIAN_POINT('Ctrl Pts',(-24.2154803966932,-1.17935753571579,
0.0502065376244371));
#60619=CARTESIAN_POINT('Ctrl Pts',(-24.2121328852638,-1.17896945751039,
0.000810547160777922));
#60620=CARTESIAN_POINT('Origin',(-35.5608671147362,0.,0.));
#60621=CARTESIAN_POINT('',(-25.3108671147362,-1.17767278411775,0.00108839386667727));
#60622=CARTESIAN_POINT('',(-25.2121328852638,-1.17589484267592,-0.000349556156004835));
#60623=CARTESIAN_POINT('',(-35.5608671147362,-1.17775,1.38253677383905E-12));
#60624=CARTESIAN_POINT('Ctrl Pts',(-25.3108671147362,-1.17767278411775,
0.00108839386667732));
#60625=CARTESIAN_POINT('Ctrl Pts',(-25.2906954059531,-1.17492606912136,
-0.2974126674257));
#60626=CARTESIAN_POINT('Ctrl Pts',(-25.2440091547643,-0.907874136102811,
-0.992648780792579));
#60627=CARTESIAN_POINT('Ctrl Pts',(-25.1708083611699,0.262028899865992,
-1.36811497676401));
#60628=CARTESIAN_POINT('Ctrl Pts',(-25.0912647339529,1.29258315287295,-0.519255743271084));
#60629=CARTESIAN_POINT('Ctrl Pts',(-25.0117211067357,1.13566746379413,0.806633216332175));
#60630=CARTESIAN_POINT('Ctrl Pts',(-24.9321774795188,-0.0645629044702633,
1.39148459042037));
#60631=CARTESIAN_POINT('Ctrl Pts',(-24.8652261488522,-1.0248656128002,0.807789446248808));
#60632=CARTESIAN_POINT('Ctrl Pts',(-24.8247893605913,-1.17556510667638,
0.206678165844237));
#60633=CARTESIAN_POINT('Ctrl Pts',(-24.8108671147362,-1.17581964054164,
-0.000162966847959863));
#60634=CARTESIAN_POINT('Ctrl Pts',(-25.2121328852638,-1.17589484267592,
-0.00034955615600487));
#60635=CARTESIAN_POINT('Ctrl Pts',(-25.2003215722281,-1.17635967926637,
-0.175800821169687));
#60636=CARTESIAN_POINT('Ctrl Pts',(-25.1619957167867,-1.05711946252861,
-0.744512129245651));
#60637=CARTESIAN_POINT('Ctrl Pts',(-25.0971553189397,-0.174976478479087,
-1.38194823897649));
#60638=CARTESIAN_POINT('Ctrl Pts',(-25.0176116917226,1.06794887502363,-0.894361729708357));
#60639=CARTESIAN_POINT('Ctrl Pts',(-24.9380680645055,1.32977124419901,0.414856772070276));
#60640=CARTESIAN_POINT('Ctrl Pts',(-24.8585244372885,0.369959725584168,
1.34295476642992));
#60641=CARTESIAN_POINT('Ctrl Pts',(-24.7832127108746,-0.860580059283745,
1.0535685672263));
#60642=CARTESIAN_POINT('Ctrl Pts',(-24.7344155268664,-1.17573331702244,
0.328115167186435));
#60643=CARTESIAN_POINT('Ctrl Pts',(-24.7121328852638,-1.17861332264333,
-0.000947007987461626));
#60644=CARTESIAN_POINT('Origin',(-35.5608671147362,0.,0.));
#60645=CARTESIAN_POINT('',(-25.8108671147362,-1.17958164686523,-0.000336615057284358));
#60646=CARTESIAN_POINT('',(-25.7121328852638,-1.17732722815968,0.00107272862214718));
#60647=CARTESIAN_POINT('',(-35.5608671147362,-1.17775,1.38253677383905E-12));
#60648=CARTESIAN_POINT('Ctrl Pts',(-25.8108671147362,-1.17958164686523,
-0.000336615057284393));
#60649=CARTESIAN_POINT('Ctrl Pts',(-25.8096305361263,-1.17965043763247,
-0.0185586411613626));
#60650=CARTESIAN_POINT('Ctrl Pts',(-25.7818794151106,-1.17099829896009,
-0.427428002609933));
#60651=CARTESIAN_POINT('Ctrl Pts',(-25.7276137516893,-0.697702759742729,
-1.20565691349503));
#60652=CARTESIAN_POINT('Ctrl Pts',(-25.6480701244723,0.637028101537958,
-1.23878687911276));
#60653=CARTESIAN_POINT('Ctrl Pts',(-25.5685264972552,1.38653415839583,-0.133868448906134));
#60654=CARTESIAN_POINT('Ctrl Pts',(-25.4889828700381,0.862259388766268,
1.09403221181801));
#60655=CARTESIAN_POINT('Ctrl Pts',(-25.4094392428211,-0.454155603459752,
1.31686765540699));
#60656=CARTESIAN_POINT('Ctrl Pts',(-25.3500673243871,-1.12531837282715,
0.580205633210485));
#60657=CARTESIAN_POINT('Ctrl Pts',(-25.3172099483588,-1.17853646683388,
0.0949496818871333));
#60658=CARTESIAN_POINT('Ctrl Pts',(-25.3108671147362,-1.17767278411775,
0.00108839386667732));
#60659=CARTESIAN_POINT('Ctrl Pts',(-25.7121328852638,-1.17732722815968,
0.00107272862214714));
#60660=CARTESIAN_POINT('Ctrl Pts',(-25.6927421599956,-1.17478830088982,
-0.286085832571626));
#60661=CARTESIAN_POINT('Ctrl Pts',(-25.6468368923217,-0.924343956719117,
-0.969864019612402));
#60662=CARTESIAN_POINT('Ctrl Pts',(-25.574417082242,0.221640587522368,-1.3752356718737));
#60663=CARTESIAN_POINT('Ctrl Pts',(-25.494873455025,1.27673702398653,-0.557081928277323));
#60664=CARTESIAN_POINT('Ctrl Pts',(-25.4153298278079,1.1589210357743,0.772851690863756));
#60665=CARTESIAN_POINT('Ctrl Pts',(-25.3357862005909,-0.0235722168554084,
1.39278212719136));
#60666=CARTESIAN_POINT('Ctrl Pts',(-25.2680538864095,-1.01203908044992,
0.831133417830471));
#60667=CARTESIAN_POINT('Ctrl Pts',(-25.2268361146338,-1.17531619413885,
0.218059708330772));
#60668=CARTESIAN_POINT('Ctrl Pts',(-25.2121328852638,-1.17589484267592,
-0.00034955615600487));
#60669=CARTESIAN_POINT('Origin',(-35.5608671147362,0.,0.));
#60670=CARTESIAN_POINT('',(-26.3108671147362,-1.17665049820237,-0.000921216280392121));
#60671=CARTESIAN_POINT('',(-26.2121328852638,-1.1796810081197,-0.000126156119591159));
#60672=CARTESIAN_POINT('',(-35.5608671147362,-1.17775,1.38253677383905E-12));
#60673=CARTESIAN_POINT('Ctrl Pts',(-26.3108671147362,-1.17665049820237,
-0.00092121628039208));
#60674=CARTESIAN_POINT('Ctrl Pts',(-26.3020511238937,-1.17760133621249,
-0.131667774133514));
#60675=CARTESIAN_POINT('Ctrl Pts',(-26.2667205906455,-1.09710611574738,
-0.65450390914198));
#60676=CARTESIAN_POINT('Ctrl Pts',(-26.2048755149917,-0.329581621862289,
-1.35343034122248));
#60677=CARTESIAN_POINT('Ctrl Pts',(-26.1253318877746,0.960369609154678,
-1.00900344291933));
#60678=CARTESIAN_POINT('Ctrl Pts',(-26.0457882605576,1.36804874678321,0.262374466051626));
#60679=CARTESIAN_POINT('Ctrl Pts',(-25.9662446333405,0.518929230876408,
1.2927142713504));
#60680=CARTESIAN_POINT('Ctrl Pts',(-25.8879375847333,-0.786308508212076,
1.13790828330489));
#60681=CARTESIAN_POINT('Ctrl Pts',(-25.8361450785319,-1.17817543580043,
0.372155446866836));
#60682=CARTESIAN_POINT('Ctrl Pts',(-25.8108671147362,-1.17958164686523,
-0.000336615057284393));
#60683=CARTESIAN_POINT('Ctrl Pts',(-26.2121328852638,-1.1796810081197,-0.000126156119591359));
#60684=CARTESIAN_POINT('Ctrl Pts',(-26.2116772901687,-1.17969117920181,
-0.00683821842843334));
#60685=CARTESIAN_POINT('Ctrl Pts',(-26.1847071526679,-1.17659452910613,
-0.40416657589943));
#60686=CARTESIAN_POINT('Ctrl Pts',(-26.1312224727615,-0.732892659131677,
-1.1845953120885));
#60687=CARTESIAN_POINT('Ctrl Pts',(-26.0516788455444,0.600284440673691,
-1.25700290115665));
#60688=CARTESIAN_POINT('Ctrl Pts',(-25.9721352183273,1.38199239250399,-0.174627404184641));
#60689=CARTESIAN_POINT('Ctrl Pts',(-25.8925915911103,0.894091946110794,
1.06817474934159));
#60690=CARTESIAN_POINT('Ctrl Pts',(-25.8130479638932,-0.415192648070296,
1.32966641238302));
#60691=CARTESIAN_POINT('Ctrl Pts',(-25.7528950619444,-1.116860453876,0.603655417092753));
#60692=CARTESIAN_POINT('Ctrl Pts',(-25.7192567024013,-1.17825998613265,
0.106569818137628));
#60693=CARTESIAN_POINT('Ctrl Pts',(-25.7121328852638,-1.17732722815968,
0.00107272862214714));
#60694=CARTESIAN_POINT('Origin',(-35.5608671147362,0.,0.));
#60695=CARTESIAN_POINT('',(-26.8108671147362,-1.17623821978682,0.000710373043126506));
#60696=CARTESIAN_POINT('',(-26.7121328852638,-1.17694686483815,-0.00101009995142842));
#60697=CARTESIAN_POINT('',(-35.5608671147362,-1.17775,1.38253677383905E-12));
#60698=CARTESIAN_POINT('Ctrl Pts',(-26.8108671147362,-1.17623821978682,
0.000710373043126492));
#60699=CARTESIAN_POINT('Ctrl Pts',(-26.7944717116611,-1.17490448726406,
-0.242657602767575));
#60700=CARTESIAN_POINT('Ctrl Pts',(-26.7515617661804,-0.98253499608713,
-0.881531533240058));
#60701=CARTESIAN_POINT('Ctrl Pts',(-26.6821372782941,0.065265851241496,
-1.39145179674781));
#60702=CARTESIAN_POINT('Ctrl Pts',(-26.6025936510769,1.20583310898822,-0.697398198505544));
#60703=CARTESIAN_POINT('Ctrl Pts',(-26.52305002386,1.23862593155623,0.637340988551213));
#60704=CARTESIAN_POINT('Ctrl Pts',(-26.4435063966428,0.133518217557687,
1.38656792822826));
#60705=CARTESIAN_POINT('Ctrl Pts',(-26.3727787602683,-0.958173793744215,
0.920123888731101));
#60706=CARTESIAN_POINT('Ctrl Pts',(-26.3285656662994,-1.17474164236858,
0.261559171599099));
#60707=CARTESIAN_POINT('Ctrl Pts',(-26.3108671147362,-1.17665049820237,
-0.00092121628039208));
#60708=CARTESIAN_POINT('Ctrl Pts',(-26.7121328852638,-1.17694686483815,
-0.00101009995142851));
#60709=CARTESIAN_POINT('Ctrl Pts',(-26.7040978779362,-1.1779136851793,-0.120098518176512));
#60710=CARTESIAN_POINT('Ctrl Pts',(-26.6695483282028,-1.10646967436812,
-0.631031077485085));
#60711=CARTESIAN_POINT('Ctrl Pts',(-26.6084842360638,-0.369281239830358,
-1.34314149259879));
#60712=CARTESIAN_POINT('Ctrl Pts',(-26.5289406088467,0.930250205829247,
-1.03683762363535));
#60713=CARTESIAN_POINT('Ctrl Pts',(-26.4493969816297,1.37517964341989,0.221987953625214));
#60714=CARTESIAN_POINT('Ctrl Pts',(-26.3698533544126,0.556759417277243,
1.27687769755144));
#60715=CARTESIAN_POINT('Ctrl Pts',(-26.2907653222907,-0.765527226002879,
1.15940251126422));
#60716=CARTESIAN_POINT('Ctrl Pts',(-26.2381918325744,-1.17909924660449,
0.383787718128221));
#60717=CARTESIAN_POINT('Ctrl Pts',(-26.2121328852638,-1.1796810081197,-0.000126156119591359));
#60718=CARTESIAN_POINT('Origin',(-35.5608671147362,0.,0.));
#60719=CARTESIAN_POINT('',(-27.3108671147362,-1.17925193811534,0.00065078897648006));
#60720=CARTESIAN_POINT('',(-27.2121328852638,-1.17605037721591,0.000553511253033878));
#60721=CARTESIAN_POINT('',(-35.5608671147362,-1.17775,1.38253677383905E-12));
#60722=CARTESIAN_POINT('Ctrl Pts',(-27.3108671147362,-1.17925193811534,
0.000650788976480016));
#60723=CARTESIAN_POINT('Ctrl Pts',(-27.2868922994286,-1.1769076025239,-0.352900079711213));
#60724=CARTESIAN_POINT('Ctrl Pts',(-27.2364029417154,-0.819671542274753,
-1.10156128989161));
#60725=CARTESIAN_POINT('Ctrl Pts',(-27.1593990415964,0.454820805275012,
-1.3166380554655));
#60726=CARTESIAN_POINT('Ctrl Pts',(-27.0798554143794,1.35351354764217,-0.329239746021173));
#60727=CARTESIAN_POINT('Ctrl Pts',(-27.0003117871623,1.00876082929865,0.960624444454579));
#60728=CARTESIAN_POINT('Ctrl Pts',(-26.9207681599452,-0.262720015497096,
1.36798242951735));
#60729=CARTESIAN_POINT('Ctrl Pts',(-26.8576199358032,-1.08051755755227,
0.69367545683447));
#60730=CARTESIAN_POINT('Ctrl Pts',(-26.8209862540668,-1.17706139108464,
0.150915552176598));
#60731=CARTESIAN_POINT('Ctrl Pts',(-26.8108671147362,-1.17623821978682,
0.000710373043126492));
#60732=CARTESIAN_POINT('Ctrl Pts',(-27.2121328852638,-1.17605037721591,
0.000553511253033739));
#60733=CARTESIAN_POINT('Ctrl Pts',(-27.1965184657036,-1.17506995411779,
-0.231314439735884));
#60734=CARTESIAN_POINT('Ctrl Pts',(-27.1543895037377,-0.996446651052049,
-0.858306279729821));
#60735=CARTESIAN_POINT('Ctrl Pts',(-27.0857459993661,0.0242758243513772,
-1.39277004117091));
#60736=CARTESIAN_POINT('Ctrl Pts',(-27.0062023721491,1.18478039693156,-0.732593416758471));
#60737=CARTESIAN_POINT('Ctrl Pts',(-26.926658744932,1.2568512341643,0.60060193007585));
#60738=CARTESIAN_POINT('Ctrl Pts',(-26.847115117715,0.174278318748489,1.38203645785679));
#60739=CARTESIAN_POINT('Ctrl Pts',(-26.7756064978256,-0.94287278904871,
0.943138512528417));
#60740=CARTESIAN_POINT('Ctrl Pts',(-26.7306124203419,-1.17472329618662,
0.272878710877991));
#60741=CARTESIAN_POINT('Ctrl Pts',(-26.7121328852638,-1.17694686483815,
-0.00101009995142851));
#60742=CARTESIAN_POINT('Origin',(-35.5608671147362,0.,0.));
#60743=CARTESIAN_POINT('',(-27.8108671147362,-1.17826087657773,-0.00103275332089385));
#60744=CARTESIAN_POINT('',(-27.7121328852638,-1.17897957473222,0.000805758147836705));
#60745=CARTESIAN_POINT('',(-35.5608671147362,-1.17775,1.38253677383905E-12));
#60746=CARTESIAN_POINT('Ctrl Pts',(-27.8108671147362,-1.17826087657773,
-0.00103275332089375));
#60747=CARTESIAN_POINT('Ctrl Pts',(-27.8058274296017,-1.17894535395326,
-0.0755146158255072));
#60748=CARTESIAN_POINT('Ctrl Pts',(-27.7742732020616,-1.13853377759971,
-0.541116554034106));
#60749=CARTESIAN_POINT('Ctrl Pts',(-27.7162044321158,-0.51827610678078,
-1.2929762608614));
#60750=CARTESIAN_POINT('Ctrl Pts',(-27.6366608048988,0.807493565332879,
-1.13505589111593));
#60751=CARTESIAN_POINT('Ctrl Pts',(-27.5571171776817,1.39143526674366,0.0656173183921381));
#60752=CARTESIAN_POINT('Ctrl Pts',(-27.4775735504646,0.697093592772551,
1.20600922754614));
#60753=CARTESIAN_POINT('Ctrl Pts',(-27.3980299232476,-0.637653834900464,
1.23846490497216));
#60754=CARTESIAN_POINT('Ctrl Pts',(-27.3424611113381,-1.16086530360064,
0.466309558213219));
#60755=CARTESIAN_POINT('Ctrl Pts',(-27.3134068418343,-1.17950028090973,
0.0381035372145209));
#60756=CARTESIAN_POINT('Ctrl Pts',(-27.3108671147362,-1.17925193811534,
0.000650788976480016));
#60757=CARTESIAN_POINT('Ctrl Pts',(-27.7121328852638,-1.17897957473222,
0.00080575814783667));
#60758=CARTESIAN_POINT('Ctrl Pts',(-27.6889390534711,-1.17630249771759,
-0.341435519304642));
#60759=CARTESIAN_POINT('Ctrl Pts',(-27.6392306792727,-0.83888794977059,
-1.07951518110267));
#60760=CARTESIAN_POINT('Ctrl Pts',(-27.5630077626685,0.415864320577861,
-1.32945649424924));
#60761=CARTESIAN_POINT('Ctrl Pts',(-27.4834641354515,1.34323472714235,-0.368941961600966));
#60762=CARTESIAN_POINT('Ctrl Pts',(-27.4039205082344,1.03660261703927,0.930512072774181));
#60763=CARTESIAN_POINT('Ctrl Pts',(-27.3243768810174,-0.222335305564666,
1.37512352722605));
#60764=CARTESIAN_POINT('Ctrl Pts',(-27.2604476733605,-1.06998394645003,
0.717145118413367));
#60765=CARTESIAN_POINT('Ctrl Pts',(-27.2230330081093,-1.17673479152724,
0.162416021733489));
#60766=CARTESIAN_POINT('Ctrl Pts',(-27.2121328852638,-1.17605037721591,
0.000553511253033739));
#60767=CARTESIAN_POINT('Origin',(-35.5608671147362,0.,0.));
#60768=CARTESIAN_POINT('',(-28.3108671147362,-1.17581803868898,-0.000156443803798287));
#60769=CARTESIAN_POINT('',(-28.2121328852638,-1.17860195998943,-0.000950464435633125));
#60770=CARTESIAN_POINT('',(-35.5608671147362,-1.17775,1.38253677383905E-12));
#60771=CARTESIAN_POINT('Ctrl Pts',(-28.3108671147362,-1.17581803868898,
-0.00015644380379834));
#60772=CARTESIAN_POINT('Ctrl Pts',(-28.2982480173692,-1.17603949646834,
-0.187637492819666));
#60773=CARTESIAN_POINT('Ctrl Pts',(-28.2591143775965,-1.04518687140584,
-0.768751257994004));
#60774=CARTESIAN_POINT('Ctrl Pts',(-28.1934661954182,-0.132817729326718,
-1.38663520249108));
#60775=CARTESIAN_POINT('Ctrl Pts',(-28.1139225682011,1.09468529645522,-0.861430110766812));
#60776=CARTESIAN_POINT('Ctrl Pts',(-28.0343789409841,1.31652312948372,0.455153362665139));
#60777=CARTESIAN_POINT('Ctrl Pts',(-27.954835313767,0.32889784917371,1.35359666770419));
#60778=CARTESIAN_POINT('Ctrl Pts',(-27.8803313716844,-0.879162171581557,
1.03038146243381));
#60779=CARTESIAN_POINT('Ctrl Pts',(-27.8323419720074,-1.17534421540685,
0.316345678846432));
#60780=CARTESIAN_POINT('Ctrl Pts',(-27.8108671147362,-1.17826087657773,
-0.00103275332089375));
#60781=CARTESIAN_POINT('Ctrl Pts',(-28.2121328852638,-1.17860195998943,
-0.00095046443563316));
#60782=CARTESIAN_POINT('Ctrl Pts',(-28.2078741836442,-1.17915367573901,
-0.063843037399876));
#60783=CARTESIAN_POINT('Ctrl Pts',(-28.1771009396189,-1.14592906312012,
-0.517718893020072));
#60784=CARTESIAN_POINT('Ctrl Pts',(-28.1198131531879,-0.556114288729563,
-1.27715880026799));
#60785=CARTESIAN_POINT('Ctrl Pts',(-28.0402695259709,0.773729670542738,
-1.15833505522063));
#60786=CARTESIAN_POINT('Ctrl Pts',(-27.9607258987538,1.39276386486699,0.0246276257872868));
#60787=CARTESIAN_POINT('Ctrl Pts',(-27.8811822715368,0.732294127643924,
1.18496540618255));
#60788=CARTESIAN_POINT('Ctrl Pts',(-27.8016386443197,-0.600919381158034,
1.25669948698159));
#60789=CARTESIAN_POINT('Ctrl Pts',(-27.7452888488954,-1.15430457516135,
0.48965019532849));
#60790=CARTESIAN_POINT('Ctrl Pts',(-27.7154535958768,-1.17936285758663,
0.0498051754229093));
#60791=CARTESIAN_POINT('Ctrl Pts',(-27.7121328852638,-1.17897957473222,
0.00080575814783667));
#60792=CARTESIAN_POINT('Origin',(-35.5608671147362,0.,0.));
#60793=CARTESIAN_POINT('',(-28.8108671147362,-1.17768483637225,0.00108828645020804));
#60794=CARTESIAN_POINT('',(-28.7121328852638,-1.17589135698706,-0.000343296306542437));
#60795=CARTESIAN_POINT('',(-35.5608671147362,-1.17775,1.38253677383905E-12));
#60796=CARTESIAN_POINT('Ctrl Pts',(-28.8108671147362,-1.17768483637225,
0.00108828645020802));
#60797=CARTESIAN_POINT('Ctrl Pts',(-28.7906686051367,-1.17493223102293,
-0.29780156408021));
#60798=CARTESIAN_POINT('Ctrl Pts',(-28.7439555531314,-0.907299205563009,
-0.993428524395512));
#60799=CARTESIAN_POINT('Ctrl Pts',(-28.6707279587205,0.26341106407934,-1.3678495331474));
#60800=CARTESIAN_POINT('Ctrl Pts',(-28.5911843315035,1.29310713187823,-0.517949495121513));
#60801=CARTESIAN_POINT('Ctrl Pts',(-28.5116407042864,1.13485188870017,0.807780245317151));
#60802=CARTESIAN_POINT('Ctrl Pts',(-28.4320970770694,-0.0659687813562216,
1.39141864796234));
#60803=CARTESIAN_POINT('Ctrl Pts',(-28.3651725472193,-1.02529707757759,
0.806987586918573));
#60804=CARTESIAN_POINT('Ctrl Pts',(-28.3247625597749,-1.17557418175436,
0.206287213506804));
#60805=CARTESIAN_POINT('Ctrl Pts',(-28.3108671147362,-1.17581803868898,
-0.00015644380379834));
#60806=CARTESIAN_POINT('Ctrl Pts',(-28.7121328852638,-1.17589135698706,
-0.000343296306542576));
#60807=CARTESIAN_POINT('Ctrl Pts',(-28.7002947714117,-1.17634882903018,
-0.176193974899314));
#60808=CARTESIAN_POINT('Ctrl Pts',(-28.6619421151538,-1.05673157934627,
-0.745316721421754));
#60809=CARTESIAN_POINT('Ctrl Pts',(-28.5970749164903,-0.173580114540252,
-1.38212432402709));
#60810=CARTESIAN_POINT('Ctrl Pts',(-28.5175312892732,1.06885196332402,-0.893282253114629));
#60811=CARTESIAN_POINT('Ctrl Pts',(-28.4379876620562,1.32935140794485,0.416200117042506));
#60812=CARTESIAN_POINT('Ctrl Pts',(-28.3584440348391,0.36860265983214,1.34332787598405));
#60813=CARTESIAN_POINT('Ctrl Pts',(-28.2831591092417,-0.861206308820253,
1.0528019527854));
#60814=CARTESIAN_POINT('Ctrl Pts',(-28.2343887260499,-1.17571871082606,
0.327724144762794));
#60815=CARTESIAN_POINT('Ctrl Pts',(-28.2121328852638,-1.17860195998943,
-0.00095046443563316));
#60816=CARTESIAN_POINT('Origin',(-35.5608671147362,0.,0.));
#60817=CARTESIAN_POINT('',(-29.3108671147362,-1.17957678883665,-0.00034361873145996));
#60818=CARTESIAN_POINT('',(-29.2121328852639,-1.17733884982054,0.0010738605839565));
#60819=CARTESIAN_POINT('',(-35.5608671147362,-1.17775,1.38253677383905E-12));
#60820=CARTESIAN_POINT('Ctrl Pts',(-29.3108671147362,-1.17957678883665,
-0.000343618731460009));
#60821=CARTESIAN_POINT('Ctrl Pts',(-29.3096037353098,-1.1796483764396,-0.0189607820253154));
#60822=CARTESIAN_POINT('Ctrl Pts',(-29.2818258134777,-1.17079998240224,
-0.428226805629651));
#60823=CARTESIAN_POINT('Ctrl Pts',(-29.2275333492399,-0.696484247896873,
-1.20636123381121));
#60824=CARTESIAN_POINT('Ctrl Pts',(-29.1479897220229,0.638279405527112,
-1.23814261476251));
#60825=CARTESIAN_POINT('Ctrl Pts',(-29.0684460948058,1.38666870691719,-0.132467472488888));
#60826=CARTESIAN_POINT('Ctrl Pts',(-28.9889024675888,0.86115357482053,1.0949028516653));
#60827=CARTESIAN_POINT('Ctrl Pts',(-28.9093588403717,-0.455485891015299,
1.31640811950435));
#60828=CARTESIAN_POINT('Ctrl Pts',(-28.8500137227542,-1.12560138845616,
0.579401192032053));
#60829=CARTESIAN_POINT('Ctrl Pts',(-28.8171831475423,-1.17854557045775,
0.0945505338539331));
#60830=CARTESIAN_POINT('Ctrl Pts',(-28.8108671147362,-1.17768483637225,
0.00108828645020802));
#60831=CARTESIAN_POINT('Ctrl Pts',(-29.2121328852639,-1.17733884982054,
0.0010738605839564));
#60832=CARTESIAN_POINT('Ctrl Pts',(-29.1927153591791,-1.17479172731383,
-0.286474385102847));
#60833=CARTESIAN_POINT('Ctrl Pts',(-29.1467832906887,-0.923787818965214,
-0.970647861375066));
#60834=CARTESIAN_POINT('Ctrl Pts',(-29.0743366797926,0.223029966864688,
-1.37501103163265));
#60835=CARTESIAN_POINT('Ctrl Pts',(-28.9947930525756,1.27729922940169,-0.555791671223127));
#60836=CARTESIAN_POINT('Ctrl Pts',(-28.9152494253585,1.15813958054323,0.774022231728725));
#60837=CARTESIAN_POINT('Ctrl Pts',(-28.8357057981415,-0.0249794256519103,
1.39275759970113));
#60838=CARTESIAN_POINT('Ctrl Pts',(-28.7680002847766,-1.01248741445764,
0.830333095236203));
#60839=CARTESIAN_POINT('Ctrl Pts',(-28.7268093138174,-1.17532420111746,
0.217669467608967));
#60840=CARTESIAN_POINT('Ctrl Pts',(-28.7121328852638,-1.17589135698706,
-0.000343296306542576));
#60841=CARTESIAN_POINT('Origin',(-35.5608671147362,0.,0.));
#60842=CARTESIAN_POINT('',(-29.8108671147362,-1.17664091671953,-0.000917630315069691));
#60843=CARTESIAN_POINT('',(-29.7121328852638,-1.17967903181214,-0.00013353279709416));
#60844=CARTESIAN_POINT('',(-35.5608671147362,-1.17775,1.38253677383905E-12));
#60845=CARTESIAN_POINT('Ctrl Pts',(-29.8108671147362,-1.17664091671953,
-0.000917630315069879));
#60846=CARTESIAN_POINT('Ctrl Pts',(-29.8020243230772,-1.17759042098373,
-0.13206434913897));
#60847=CARTESIAN_POINT('Ctrl Pts',(-29.7666669890126,-1.09677718246914,
-0.655309508255734));
#60848=CARTESIAN_POINT('Ctrl Pts',(-29.7047951125423,-0.328213992546994,
-1.35376264873402));
#60849=CARTESIAN_POINT('Ctrl Pts',(-29.6252514853253,0.96138858254731,-1.00803260232924));
#60850=CARTESIAN_POINT('Ctrl Pts',(-29.5457078581082,1.3677829540518,0.263756563172021));
#60851=CARTESIAN_POINT('Ctrl Pts',(-29.4661642308912,0.517622850415724,
1.29323792039148));
#60852=CARTESIAN_POINT('Ctrl Pts',(-29.3878839831004,-0.787011143946497,
1.13716667660531));
#60853=CARTESIAN_POINT('Ctrl Pts',(-29.3361182777155,-1.17814596750797,
0.371757600210271));
#60854=CARTESIAN_POINT('Ctrl Pts',(-29.3108671147362,-1.17957678883665,
-0.000343618731460009));
#60855=CARTESIAN_POINT('Ctrl Pts',(-29.7121328852638,-1.17967903181214,
-0.000133532797094274));
#60856=CARTESIAN_POINT('Ctrl Pts',(-29.7116504893523,-1.17969040234477,
-0.00724047061861174));
#60857=CARTESIAN_POINT('Ctrl Pts',(-29.684653551035,-1.17640830311254,-0.404964318864758));
#60858=CARTESIAN_POINT('Ctrl Pts',(-29.6311420703121,-0.731695409267114,
-1.18533519786117));
#60859=CARTESIAN_POINT('Ctrl Pts',(-29.551598443095,0.601554168281548,-1.25639575208381));
#60860=CARTESIAN_POINT('Ctrl Pts',(-29.4720548158779,1.38216812483898,-0.173230995812698));
#60861=CARTESIAN_POINT('Ctrl Pts',(-29.3925111886609,0.893012241438832,
1.06907756494632));
#60862=CARTESIAN_POINT('Ctrl Pts',(-29.3129675614438,-0.416535886952527,
1.3292462368244));
#60863=CARTESIAN_POINT('Ctrl Pts',(-29.2528414603115,-1.11715749969954,
0.602850456415611));
#60864=CARTESIAN_POINT('Ctrl Pts',(-29.2192299015848,-1.1782698113613,0.106171419552341));
#60865=CARTESIAN_POINT('Ctrl Pts',(-29.2121328852639,-1.17733884982054,
0.0010738605839564));
#60866=CARTESIAN_POINT('Origin',(-35.5608671147362,0.,0.));
#60867=CARTESIAN_POINT('',(-30.3108671147362,-1.17624550500564,0.000715395404373505));
#60868=CARTESIAN_POINT('',(-30.2121328852638,-1.17693618625551,-0.00100756867321319));
#60869=CARTESIAN_POINT('',(-35.5608671147362,-1.17775,1.38253677383905E-12));
#60870=CARTESIAN_POINT('Ctrl Pts',(-30.3108671147362,-1.17624550500564,
0.000715395404373449));
#60871=CARTESIAN_POINT('Ctrl Pts',(-30.2944449108447,-1.17489964449614,
-0.24304662073349));
#60872=CARTESIAN_POINT('Ctrl Pts',(-30.2515081645475,-0.982048518931031,
-0.882327361829687));
#60873=CARTESIAN_POINT('Ctrl Pts',(-30.1820568758447,0.0666716946350309,
-1.39138514407244));
#60874=CARTESIAN_POINT('Ctrl Pts',(-30.1025132486276,1.2065371214959,-0.696179508793066));
#60875=CARTESIAN_POINT('Ctrl Pts',(-30.0229696214105,1.23798135115748,0.638592129764595));
#60876=CARTESIAN_POINT('Ctrl Pts',(-29.9434259941935,0.132117207199287,
1.38670212287024));
#60877=CARTESIAN_POINT('Ctrl Pts',(-29.8727251586353,-0.958689471350472,
0.919332479554083));
#60878=CARTESIAN_POINT('Ctrl Pts',(-29.8285388654829,-1.17474339347833,
0.261170657603315));
#60879=CARTESIAN_POINT('Ctrl Pts',(-29.8108671147362,-1.17664091671953,
-0.000917630315069879));
#60880=CARTESIAN_POINT('Ctrl Pts',(-30.2121328852638,-1.17693618625551,
-0.00100756867321311));
#60881=CARTESIAN_POINT('Ctrl Pts',(-30.2040710771197,-1.17790317456817,
-0.12049594655812));
#60882=CARTESIAN_POINT('Ctrl Pts',(-30.1694947265699,-1.10615540179254,
-0.631836479916431));
#60883=CARTESIAN_POINT('Ctrl Pts',(-30.1084038336144,-0.367923985762689,
-1.34351391653814));
#60884=CARTESIAN_POINT('Ctrl Pts',(-30.0288602063974,0.931297317327677,
-1.03589720048344));
#60885=CARTESIAN_POINT('Ctrl Pts',(-29.9493165791803,1.37495465224026,0.223377276180953));
#60886=CARTESIAN_POINT('Ctrl Pts',(-29.8697729519633,0.555469018255743,
1.2774395770404));
#60887=CARTESIAN_POINT('Ctrl Pts',(-29.7907117206578,-0.766250209985431,
1.15866871809116));
#60888=CARTESIAN_POINT('Ctrl Pts',(-29.738165031758,-1.17906542924158,0.383387226930625));
#60889=CARTESIAN_POINT('Ctrl Pts',(-29.7121328852638,-1.17967903181214,
-0.000133532797094274));
#60890=CARTESIAN_POINT('Origin',(-35.5608671147362,0.,0.));
#60891=CARTESIAN_POINT('',(-30.8108671147362,-1.17926042646981,0.000644971907101031));
#60892=CARTESIAN_POINT('',(-30.7121328852638,-1.17605601445831,0.000559203359190574));
#60893=CARTESIAN_POINT('',(-35.5608671147362,-1.17775,1.38253677383905E-12));
#60894=CARTESIAN_POINT('Ctrl Pts',(-30.8108671147362,-1.17926042646981,
0.000644971907101054));
#60895=CARTESIAN_POINT('Ctrl Pts',(-30.7868654986121,-1.1769303683839,-0.353294409864568));
#60896=CARTESIAN_POINT('Ctrl Pts',(-30.7363493400824,-0.819001798932681,
-1.10231448839058));
#60897=CARTESIAN_POINT('Ctrl Pts',(-30.659318639147,0.456150860510873,-1.31617784758222));
#60898=CARTESIAN_POINT('Ctrl Pts',(-30.57977501193,1.35384550969123,-0.327872032811375));
#60899=CARTESIAN_POINT('Ctrl Pts',(-30.5002313847129,1.00778973135526,0.961643172588391));
#60900=CARTESIAN_POINT('Ctrl Pts',(-30.4206877574958,-0.264102045436351,
1.3677162876881));
#60901=CARTESIAN_POINT('Ctrl Pts',(-30.3575663341703,-1.080871079543,0.692869917692197));
#60902=CARTESIAN_POINT('Ctrl Pts',(-30.3209594532504,-1.1770726095736,0.150520427665763));
#60903=CARTESIAN_POINT('Ctrl Pts',(-30.3108671147362,-1.17624550500564,
0.000715395404373449));
#60904=CARTESIAN_POINT('Ctrl Pts',(-30.7121328852638,-1.17605601445831,
0.000559203359190626));
#60905=CARTESIAN_POINT('Ctrl Pts',(-30.6964916648872,-1.17506353315699,
-0.231703946270628));
#60906=CARTESIAN_POINT('Ctrl Pts',(-30.6543359021048,-0.995977674532915,
-0.859104347736037));
#60907=CARTESIAN_POINT('Ctrl Pts',(-30.5856655969168,0.0256830205774446,
-1.39274480278519));
#60908=CARTESIAN_POINT('Ctrl Pts',(-30.5061219696997,1.18551998026519,-0.731395980043076));
#60909=CARTESIAN_POINT('Ctrl Pts',(-30.4265783424827,1.25624376438813,0.601871504282349));
#60910=CARTESIAN_POINT('Ctrl Pts',(-30.3470347152656,0.172881866032571,
1.38221183746495));
#60911=CARTESIAN_POINT('Ctrl Pts',(-30.2755528961927,-0.943406691408323,
0.942350301898318));
#60912=CARTESIAN_POINT('Ctrl Pts',(-30.2305856195254,-1.17472283931786,
0.272490292481629));
#60913=CARTESIAN_POINT('Ctrl Pts',(-30.2121328852638,-1.17693618625551,
-0.00100756867321311));
#60914=CARTESIAN_POINT('Origin',(-35.5608671147362,0.,0.));
#60915=CARTESIAN_POINT('',(-31.3108671147362,-1.17824890665216,-0.00103493412604925));
#60916=CARTESIAN_POINT('',(-31.2121328852638,-1.17898964596467,0.000800932373318346));
#60917=CARTESIAN_POINT('',(-35.5608671147362,-1.17775,1.38253677383905E-12));
#60918=CARTESIAN_POINT('Ctrl Pts',(-31.3108671147362,-1.17824890665216,
-0.00103493412604934));
#60919=CARTESIAN_POINT('Ctrl Pts',(-31.3058006287853,-1.17893768761402,
-0.0759148480283834));
#60920=CARTESIAN_POINT('Ctrl Pts',(-31.2742196004287,-1.13827309184918,
-0.541919893813802));
#60921=CARTESIAN_POINT('Ctrl Pts',(-31.2161240296664,-0.516969461947962,
-1.29349924987385));
#60922=CARTESIAN_POINT('Ctrl Pts',(-31.1365804024493,0.808639975965988,
-1.13423944706605));
#60923=CARTESIAN_POINT('Ctrl Pts',(-31.0570367752323,1.39136825896598,0.067023144904906));
#60924=CARTESIAN_POINT('Ctrl Pts',(-30.9774931480152,0.695874725271205,
1.20671293220041));
#60925=CARTESIAN_POINT('Ctrl Pts',(-30.8979495207982,-0.638904813258247,
1.23782000856604));
#60926=CARTESIAN_POINT('Ctrl Pts',(-30.8424075097052,-1.16108388648063,
0.465509085426306));
#60927=CARTESIAN_POINT('Ctrl Pts',(-30.8133800410178,-1.17950437938413,
0.0377017921632874));
#60928=CARTESIAN_POINT('Ctrl Pts',(-30.8108671147362,-1.17926042646981,
0.000644971907101054));
#60929=CARTESIAN_POINT('Ctrl Pts',(-31.2121328852638,-1.17898964596467,
0.000800932373318424));
#60930=CARTESIAN_POINT('Ctrl Pts',(-31.1889122526546,-1.17632142805659,
-0.341828155202142));
#60931=CARTESIAN_POINT('Ctrl Pts',(-31.1391770776397,-0.838238088557327,
-1.08027477832003));
#60932=CARTESIAN_POINT('Ctrl Pts',(-31.0629273602191,0.417207347022933,
-1.32903564016216));
#60933=CARTESIAN_POINT('Ctrl Pts',(-30.9833837330021,1.34360680823865,-0.367584613505395));
#60934=CARTESIAN_POINT('Ctrl Pts',(-30.903840105785,1.03566192942565,0.931558946696078));
#60935=CARTESIAN_POINT('Ctrl Pts',(-30.824296478568,-0.223724571245162,
1.3748981851222));
#60936=CARTESIAN_POINT('Ctrl Pts',(-30.7603940717276,-1.07035290206037,
0.716339876975727));
#60937=CARTESIAN_POINT('Ctrl Pts',(-30.7230062072929,-1.17674595862744,
0.162021797746519));
#60938=CARTESIAN_POINT('Ctrl Pts',(-30.7121328852638,-1.17605601445831,
0.000559203359190626));
#60939=CARTESIAN_POINT('Origin',(-35.5608671147362,0.,0.));
#60940=CARTESIAN_POINT('',(-31.8108671147362,-1.17581650239264,-0.000149915200615911));
#60941=CARTESIAN_POINT('',(-31.7121328852638,-1.17859056986776,-0.000953879663846968));
#60942=CARTESIAN_POINT('',(-35.5608671147362,-1.17775,1.38253677383905E-12));
#60943=CARTESIAN_POINT('Ctrl Pts',(-31.8108671147362,-1.17581650239264,
-0.000149915200616038));
#60944=CARTESIAN_POINT('Ctrl Pts',(-31.7982212165527,-1.1760291537976,-0.188029754032307));
#60945=CARTESIAN_POINT('Ctrl Pts',(-31.7590607759636,-1.0447823457967,-0.769555013578587));
#60946=CARTESIAN_POINT('Ctrl Pts',(-31.6933857929688,-0.131416651354211,
-1.38676868934885));
#60947=CARTESIAN_POINT('Ctrl Pts',(-31.6138421657517,1.09555509809422,-0.860323637389223));
#60948=CARTESIAN_POINT('Ctrl Pts',(-31.5342985385347,1.31606258565414,0.45648330161381));
#60949=CARTESIAN_POINT('Ctrl Pts',(-31.4547549113176,0.327530052156675,
1.35392828426963));
#60950=CARTESIAN_POINT('Ctrl Pts',(-31.3802777700514,-0.879768336219877,
1.02960936733916));
#60951=CARTESIAN_POINT('Ctrl Pts',(-31.332315171191,-1.17533307641041,0.315955705199351));
#60952=CARTESIAN_POINT('Ctrl Pts',(-31.3108671147362,-1.17824890665216,
-0.00103493412604934));
#60953=CARTESIAN_POINT('Ctrl Pts',(-31.7121328852638,-1.17859056986776,
-0.00095387966384702));
#60954=CARTESIAN_POINT('Ctrl Pts',(-31.7078473828277,-1.17914702414124,
-0.0642438336544744));
#60955=CARTESIAN_POINT('Ctrl Pts',(-31.677047337986,-1.14568168278089,-0.51852142935964));
#60956=CARTESIAN_POINT('Ctrl Pts',(-31.6197327507386,-0.554823606020508,
-1.27772002779702));
#60957=CARTESIAN_POINT('Ctrl Pts',(-31.5401891235215,0.774899618904291,
-1.1575527132071));
#60958=CARTESIAN_POINT('Ctrl Pts',(-31.4606454963045,1.39273827103593,0.0260348155934577));
#60959=CARTESIAN_POINT('Ctrl Pts',(-31.3811018690874,0.73109650415408,1.18570468702998));
#60960=CARTESIAN_POINT('Ctrl Pts',(-31.3015582418703,-0.602188801882199,
1.25609169654084));
#60961=CARTESIAN_POINT('Ctrl Pts',(-31.2452352472625,-1.154535882638,0.488848760380386));
#60962=CARTESIAN_POINT('Ctrl Pts',(-31.2154267950603,-1.17936813992108,
0.0494037989323538));
#60963=CARTESIAN_POINT('Ctrl Pts',(-31.2121328852638,-1.17898964596467,
0.000800932373318424));
#60964=CARTESIAN_POINT('Origin',(-35.5608671147362,0.,0.));
#60965=CARTESIAN_POINT('',(-32.3108671147362,-1.1776968972288,0.00108813574317774));
#60966=CARTESIAN_POINT('',(-32.2121328852638,-1.17588793485307,-0.000337024215327775));
#60967=CARTESIAN_POINT('',(-35.5608671147362,-1.17775,1.38253677383905E-12));
#60968=CARTESIAN_POINT('Ctrl Pts',(-32.3108671147362,-1.1776968972288,0.00108813574317767));
#60969=CARTESIAN_POINT('Ctrl Pts',(-32.2906418043202,-1.17493849100873,
-0.298190476586958));
#60970=CARTESIAN_POINT('Ctrl Pts',(-32.2439019514985,-0.906723625724865,
-0.994208119680003));
#60971=CARTESIAN_POINT('Ctrl Pts',(-32.1706475562712,0.264792959390405,
-1.3675826931817));
#60972=CARTESIAN_POINT('Ctrl Pts',(-32.0911039290541,1.29362979082703,-0.516642718223328));
#60973=CARTESIAN_POINT('Ctrl Pts',(-32.011560301837,1.1340351551021,0.808926449684369));
#60974=CARTESIAN_POINT('Ctrl Pts',(-31.93201667462,-0.0673745908983318,
1.39135128508784));
#60975=CARTESIAN_POINT('Ctrl Pts',(-31.8651189455863,-1.02572796862834,
0.806185680098539));
#60976=CARTESIAN_POINT('Ctrl Pts',(-31.8247357589584,-1.17558328948551,
0.20589623537659));
#60977=CARTESIAN_POINT('Ctrl Pts',(-31.8108671147362,-1.17581650239264,
-0.000149915200616038));
#60978=CARTESIAN_POINT('Ctrl Pts',(-32.2121328852638,-1.17588793485307,
-0.000337024215328035));
#60979=CARTESIAN_POINT('Ctrl Pts',(-32.2002679705952,-1.17633799208892,
-0.176587098471389));
#60980=CARTESIAN_POINT('Ctrl Pts',(-32.1618885135209,-1.05634314907566,
-0.746121290085078));
#60981=CARTESIAN_POINT('Ctrl Pts',(-32.096994514041,-0.172183573404041,
-1.38229899814921));
#60982=CARTESIAN_POINT('Ctrl Pts',(-32.0174508868238,1.06975396049637,-0.892201864620813));
#60983=CARTESIAN_POINT('Ctrl Pts',(-31.9379072596068,1.3289302146337,0.417543037140155));
#60984=CARTESIAN_POINT('Ctrl Pts',(-31.8583636323897,0.367245217795309,
1.34369961421373));
#60985=CARTESIAN_POINT('Ctrl Pts',(-31.7831055076088,-0.861831888195839,
1.05203514828171));
#60986=CARTESIAN_POINT('Ctrl Pts',(-31.7343619252334,-1.17570422352421,
0.327333162035316));
#60987=CARTESIAN_POINT('Ctrl Pts',(-31.7121328852638,-1.17859056986776,
-0.00095387966384702));
#60988=CARTESIAN_POINT('Origin',(-35.5608671147362,0.,0.));
#60989=CARTESIAN_POINT('',(-32.8108671147362,-1.17957184097153,-0.000350604622900076));
#60990=CARTESIAN_POINT('',(-32.7121328852638,-1.1773504918584,0.00107495084775092));
#60991=CARTESIAN_POINT('',(-35.5608671147362,-1.17775,1.38253677383905E-12));
#60992=CARTESIAN_POINT('Ctrl Pts',(-32.8108671147362,-1.17957184097153,
-0.000350604622899962));
#60993=CARTESIAN_POINT('Ctrl Pts',(-32.8095769344933,-1.17964627158723,
-0.0193629176176901));
#60994=CARTESIAN_POINT('Ctrl Pts',(-32.7817722118448,-1.17060124696026,
-0.429025645350123));
#60995=CARTESIAN_POINT('Ctrl Pts',(-32.7274529467905,-0.69526502492905,
-1.20706432189118));
#60996=CARTESIAN_POINT('Ctrl Pts',(-32.6479093195736,0.639530057869942,
-1.23749708685117));
#60997=CARTESIAN_POINT('Ctrl Pts',(-32.5683656923564,1.38680183990368,-0.131066360639972));
#60998=CARTESIAN_POINT('Ctrl Pts',(-32.4888220651394,0.860046881755779,
1.09577237368332));
#60999=CARTESIAN_POINT('Ctrl Pts',(-32.4092784379223,-0.456815713582613,
1.31594723981434));
#61000=CARTESIAN_POINT('Ctrl Pts',(-32.3499601211213,-1.1258839276056,0.578596770904729));
#61001=CARTESIAN_POINT('Ctrl Pts',(-32.3171563467259,-1.1785546470622,0.094151361166444));
#61002=CARTESIAN_POINT('Ctrl Pts',(-32.3108671147362,-1.1776968972288,0.00108813574317767));
#61003=CARTESIAN_POINT('Ctrl Pts',(-32.7121328852638,-1.1773504918584,0.00107495084775085));
#61004=CARTESIAN_POINT('Ctrl Pts',(-32.6926885583627,-1.17479524368154,
-0.28686294584429));
#61005=CARTESIAN_POINT('Ctrl Pts',(-32.6467296890558,-0.923231040420216,
-0.971431569472807));
#61006=CARTESIAN_POINT('Ctrl Pts',(-32.5742562773433,0.224419118509842,
-1.37478498777756));
#61007=CARTESIAN_POINT('Ctrl Pts',(-32.4947126501262,1.27786013090699,-0.554500846765326));
#61008=CARTESIAN_POINT('Ctrl Pts',(-32.4151690229092,1.15735694303011,0.775191982424803));
#61009=CARTESIAN_POINT('Ctrl Pts',(-32.3356253956921,-0.0263866089456238,
1.39273165043428));
#61010=CARTESIAN_POINT('Ctrl Pts',(-32.2679466831437,-1.01293516475784,
0.82953271490403));
#61011=CARTESIAN_POINT('Ctrl Pts',(-32.2267825130009,-1.17533224851651,
0.217279203848309));
#61012=CARTESIAN_POINT('Ctrl Pts',(-32.2121328852638,-1.17588793485307,
-0.000337024215328035));
#61013=CARTESIAN_POINT('Origin',(-35.5608671147362,0.,0.));
#61014=CARTESIAN_POINT('',(-33.3108671147362,-1.17663137595576,-0.000914001560779414));
#61015=CARTESIAN_POINT('',(-33.2121328852639,-1.179676948955,-0.000140904201940406));
#61016=CARTESIAN_POINT('',(-35.5608671147362,-1.17775,1.38253677383905E-12));
#61017=CARTESIAN_POINT('Ctrl Pts',(-33.3108671147362,-1.17663137595576,
-0.000914001560779511));
#61018=CARTESIAN_POINT('Ctrl Pts',(-33.3019975222608,-1.1775794950042,-0.132460896041139));
#61019=CARTESIAN_POINT('Ctrl Pts',(-33.2666133873797,-1.09644774808449,
-0.656115154141397));
#61020=CARTESIAN_POINT('Ctrl Pts',(-33.204714710093,-0.326846022470247,
-1.35409354000658));
#61021=CARTESIAN_POINT('Ctrl Pts',(-33.1251710828758,0.962406571507915,
-1.00706075074908));
#61022=CARTESIAN_POINT('Ctrl Pts',(-33.0456274556588,1.36751576661517,0.26513840054929));
#61023=CARTESIAN_POINT('Ctrl Pts',(-32.9660838284418,0.516315940709615,
1.29376024423113));
#61024=CARTESIAN_POINT('Ctrl Pts',(-32.8878303814675,-0.787713083824443,
1.1364248141512));
#61025=CARTESIAN_POINT('Ctrl Pts',(-32.836091476899,-1.17811664522137,0.371359837535488));
#61026=CARTESIAN_POINT('Ctrl Pts',(-32.8108671147362,-1.17957184097153,
-0.000350604622899962));
#61027=CARTESIAN_POINT('Ctrl Pts',(-33.2121328852639,-1.179676948955,-0.000140904201940543));
#61028=CARTESIAN_POINT('Ctrl Pts',(-33.2116236885358,-1.17968958197449,
-0.0076427229676073));
#61029=CARTESIAN_POINT('Ctrl Pts',(-33.1845999494021,-1.17622166758078,
-0.405762103065146));
#61030=CARTESIAN_POINT('Ctrl Pts',(-33.1310616678627,-0.730497410775578,
-1.1860738687982));
#61031=CARTESIAN_POINT('Ctrl Pts',(-33.0515180406456,0.602823280911789,
-1.25578732295739));
#61032=CARTESIAN_POINT('Ctrl Pts',(-32.9719744134286,1.38234244666654,-0.171834409267923));
#61033=CARTESIAN_POINT('Ctrl Pts',(-32.8924307862115,0.891931624897046,
1.06997928849094));
#61034=CARTESIAN_POINT('Ctrl Pts',(-32.8128871589945,-0.417878700488076,
1.32882470468588));
#61035=CARTESIAN_POINT('Ctrl Pts',(-32.7527878586786,-1.11745405938805,
0.602045511337059));
#61036=CARTESIAN_POINT('Ctrl Pts',(-32.7192031007684,-1.17827961403218,
0.105772994234821));
#61037=CARTESIAN_POINT('Ctrl Pts',(-32.7121328852638,-1.1773504918584,0.00107495084775085));
#61038=CARTESIAN_POINT('Origin',(-35.5608671147362,0.,0.));
#61039=CARTESIAN_POINT('',(-33.8108671147362,-1.17625258863493,0.000721924261463078));
#61040=CARTESIAN_POINT('',(-33.7121328852638,-1.17692552717653,-0.001004960261487));
#61041=CARTESIAN_POINT('',(-35.5608671147362,-1.17775,1.38253677383905E-12));
#61042=CARTESIAN_POINT('Ctrl Pts',(-33.8108671147362,-1.17625258863493,
0.000721924261462958));
#61043=CARTESIAN_POINT('Ctrl Pts',(-33.7944181100282,-1.17489470568404,
-0.243434697208882));
#61044=CARTESIAN_POINT('Ctrl Pts',(-33.7514545629146,-0.981561844828172,
-0.883125560569472));
#61045=CARTESIAN_POINT('Ctrl Pts',(-33.6819764733953,0.0680777368036397,
-1.39131546907066));
#61046=CARTESIAN_POINT('Ctrl Pts',(-33.6024328461782,1.20723976173548,-0.694960952389941));
#61047=CARTESIAN_POINT('Ctrl Pts',(-33.5228892189612,1.23733558104474,0.639843063744817));
#61048=CARTESIAN_POINT('Ctrl Pts',(-33.4433455917441,0.130716022946506,
1.38683466763195));
#61049=CARTESIAN_POINT('Ctrl Pts',(-33.3726715570025,-0.95920451437908,
0.918541050994175));
#61050=CARTESIAN_POINT('Ctrl Pts',(-33.3285120646665,-1.17474521115347,
0.260782166896676));
#61051=CARTESIAN_POINT('Ctrl Pts',(-33.3108671147362,-1.17663137595576,
-0.000914001560779511));
#61052=CARTESIAN_POINT('Ctrl Pts',(-33.7121328852638,-1.17692552717653,
-0.00100496026148728));
#61053=CARTESIAN_POINT('Ctrl Pts',(-33.7040442763033,-1.17789265561524,
-0.12089336944156));
#61054=CARTESIAN_POINT('Ctrl Pts',(-33.669441124937,-1.10584072736996,-0.632642166838988));
#61055=CARTESIAN_POINT('Ctrl Pts',(-33.6083234311651,-0.366566277470248,
-1.34388474473925));
#61056=CARTESIAN_POINT('Ctrl Pts',(-33.528779803948,0.932343436689741,-1.03495583798244));
#61057=CARTESIAN_POINT('Ctrl Pts',(-33.4492361767309,1.37472827927823,0.224766432947515));
#61058=CARTESIAN_POINT('Ctrl Pts',(-33.3696925495139,0.554178040687849,
1.2780001196717));
#61059=CARTESIAN_POINT('Ctrl Pts',(-33.2906581190248,-0.76697248715969,
1.15793466444302));
#61060=CARTESIAN_POINT('Ctrl Pts',(-33.2381382309415,-1.1790317640579,0.38298683302465));
#61061=CARTESIAN_POINT('Ctrl Pts',(-33.2121328852639,-1.179676948955,-0.000140904201940543));
#61062=CARTESIAN_POINT('Origin',(-35.5608671147362,0.,0.));
#61063=CARTESIAN_POINT('',(-34.3108671147362,-1.17925499677644,0.000722179416794065));
#61064=CARTESIAN_POINT('',(-34.2121328852638,-1.17605840265479,0.000574308414346136));
#61065=CARTESIAN_POINT('',(-35.5608671147362,-1.17775,1.38253677383905E-12));
#61066=CARTESIAN_POINT('Ctrl Pts',(-34.3108671147362,-1.17925499677644,
0.000722179416794018));
#61067=CARTESIAN_POINT('Ctrl Pts',(-34.2868386977957,-1.17693533461402,
-0.353580965932757));
#61068=CARTESIAN_POINT('Ctrl Pts',(-34.2362957384495,-0.818353920066329,
-1.10320287134604));
#61069=CARTESIAN_POINT('Ctrl Pts',(-34.1592382366976,0.457492926185055,
-1.31564139210814));
#61070=CARTESIAN_POINT('Ctrl Pts',(-34.0796946094806,1.3541695165413,-0.326543447000047));
#61071=CARTESIAN_POINT('Ctrl Pts',(-34.0001509822635,1.00682106773482,0.962681709799215));
#61072=CARTESIAN_POINT('Ctrl Pts',(-33.9206073550465,-0.265485630343504,
1.36743779586005));
#61073=CARTESIAN_POINT('Ctrl Pts',(-33.8575127325373,-1.0812236919471,0.692066684536782));
#61074=CARTESIAN_POINT('Ctrl Pts',(-33.8209326524339,-1.17708350954923,
0.150127175290172));
#61075=CARTESIAN_POINT('Ctrl Pts',(-33.8108671147362,-1.17625258863493,
0.000721924261462958));
#61076=CARTESIAN_POINT('Ctrl Pts',(-34.2121328852638,-1.17605840265479,
0.000574308414346206));
#61077=CARTESIAN_POINT('Ctrl Pts',(-34.1964648640707,-1.17505531307848,
-0.232088160436699));
#61078=CARTESIAN_POINT('Ctrl Pts',(-34.1542823004719,-0.995513626366357,
-0.85991809699752));
#61079=CARTESIAN_POINT('Ctrl Pts',(-34.0855851944674,0.0270938664892442,
-1.39270766067608));
#61080=CARTESIAN_POINT('Ctrl Pts',(-34.0060415672503,1.18625641663401,-0.730203319351427));
#61081=CARTESIAN_POINT('Ctrl Pts',(-33.9264979400333,1.25563603260232,0.603143373819632));
#61082=CARTESIAN_POINT('Ctrl Pts',(-33.8469543128163,0.171484699201278,
1.3823842729852));
#61083=CARTESIAN_POINT('Ctrl Pts',(-33.7754992945597,-0.943939764166423,
0.941562544723186));
#61084=CARTESIAN_POINT('Ctrl Pts',(-33.7305588187089,-1.17472239876083,
0.272102054697359));
#61085=CARTESIAN_POINT('Ctrl Pts',(-33.7121328852638,-1.17692552717653,
-0.00100496026148728));
#61086=CARTESIAN_POINT('Origin',(-0.2,3.28582941601228E-17,0.));
#61087=CARTESIAN_POINT('',(-0.2,1.38699088616441,0.466999498604503));
#61088=CARTESIAN_POINT('Ctrl Pts',(-0.2,-0.207979487136895,-1.16121778488279));
#61089=CARTESIAN_POINT('Ctrl Pts',(-0.199999999999999,-0.17996785785622,
-1.16987676038429));
#61090=CARTESIAN_POINT('Ctrl Pts',(-0.200000000000005,-0.151667340461406,
-1.17740349654605));
#61091=CARTESIAN_POINT('Ctrl Pts',(-0.200000000000004,-0.123132736344806,
-1.18376041834314));
#61092=CARTESIAN_POINT('Ctrl Pts',(-0.200000000000001,-0.0760735798974293,
-1.1942442286722));
#61093=CARTESIAN_POINT('Ctrl Pts',(-0.199999999999998,-0.0283788177258679,
-1.20154929893047));
#61094=CARTESIAN_POINT('Ctrl Pts',(-0.199999999999998,0.0196878622471927,
-1.20583213317713));
#61095=CARTESIAN_POINT('Ctrl Pts',(-0.199999999999998,0.0380691674922849,
-1.20746994306219));
#61096=CARTESIAN_POINT('Ctrl Pts',(-0.200000000000004,0.0565050987880124,
-1.2086652918681));
#61097=CARTESIAN_POINT('Ctrl Pts',(-0.200000000000004,0.0749816324965036,
-1.20942512509166));
#61098=CARTESIAN_POINT('Ctrl Pts',(-0.200000000000004,0.0864312154600023,
-1.20989598037592));
#61099=CARTESIAN_POINT('Ctrl Pts',(-0.200000000000005,0.09789848461842,
-1.21019959627083));
#61100=CARTESIAN_POINT('Ctrl Pts',(-0.200000000000005,0.109373451700485,
-1.21033736826952));
#61101=CARTESIAN_POINT('Ctrl Pts',(-0.200000000000004,0.159816976356299,
-1.2109430088054));
#61102=CARTESIAN_POINT('Ctrl Pts',(-0.199999999999996,0.21028424266955,
-1.20834757047201));
#61103=CARTESIAN_POINT('Ctrl Pts',(-0.199999999999995,0.260486404812435,
-1.20272430978437));
#61104=CARTESIAN_POINT('Ctrl Pts',(-0.199999999999995,0.296855798949691,
-1.19865048954325));
#61105=CARTESIAN_POINT('Ctrl Pts',(-0.199999999999997,0.333086695276272,
-1.19298646331018));
#61106=CARTESIAN_POINT('Ctrl Pts',(-0.199999999999996,0.369073996782841,
-1.18578183454027));
#61107=CARTESIAN_POINT('Ctrl Pts',(-0.199999999999995,0.384213139928643,
-1.18275099027872));
#61108=CARTESIAN_POINT('Ctrl Pts',(-0.199999999999998,0.399309200131859,
-1.17944734014573));
#61109=CARTESIAN_POINT('Ctrl Pts',(-0.199999999999998,0.414354411325149,
-1.17587387674941));
#61110=CARTESIAN_POINT('Ctrl Pts',(-0.199999999999997,0.427366804737433,
-1.17278323807642));
#61111=CARTESIAN_POINT('Ctrl Pts',(-0.199999999999993,0.440344323191234,
-1.16948974515456));
#61112=CARTESIAN_POINT('Ctrl Pts',(-0.199999999999993,0.453257211519439,
-1.16600226357088));
#61113=CARTESIAN_POINT('Ctrl Pts',(-0.199999999999993,0.503975772807244,
-1.15230431746102));
#61114=CARTESIAN_POINT('Ctrl Pts',(-0.199999999999988,0.5537718606903,-1.1356014144362));
#61115=CARTESIAN_POINT('Ctrl Pts',(-0.199999999999992,0.602349869633212,
-1.11606206524489));
#61116=CARTESIAN_POINT('Ctrl Pts',(-0.199999999999996,0.651837272735973,
-1.09615693387296));
#61117=CARTESIAN_POINT('Ctrl Pts',(-0.2,0.700061744369224,-1.07330810109062));
#61118=CARTESIAN_POINT('Ctrl Pts',(-0.2,0.746713474323926,-1.04764073086544));
#61119=CARTESIAN_POINT('Ctrl Pts',(-0.2,0.773395470711291,-1.03296053186132));
#61120=CARTESIAN_POINT('Ctrl Pts',(-0.199999999999994,0.799562953931442,
-1.01735738288161));
#61121=CARTESIAN_POINT('Ctrl Pts',(-0.199999999999993,0.825155999701759,
-1.00084728202755));
#61122=CARTESIAN_POINT('Ctrl Pts',(-0.199999999999992,0.84136793032273,
-0.990388948463293));
#61123=CARTESIAN_POINT('Ctrl Pts',(-0.199999999999994,0.857349325029275,
-0.979566585249447));
#61124=CARTESIAN_POINT('Ctrl Pts',(-0.199999999999994,0.873084385111579,
-0.968383188012168));
#61125=CARTESIAN_POINT('Ctrl Pts',(-0.199999999999993,0.880884272467831,
-0.962839565156282));
#61126=CARTESIAN_POINT('Ctrl Pts',(-0.199999999999998,0.888622356506473,
-0.95720800218513));
#61127=CARTESIAN_POINT('Ctrl Pts',(-0.199999999999998,0.89628698404453,
-0.951496475501582));
#61128=CARTESIAN_POINT('Ctrl Pts',(-0.199999999999999,0.940230294863368,
-0.918750801813058));
#61129=CARTESIAN_POINT('Ctrl Pts',(-0.2,0.981849241670539,-0.883317934714933));
#61130=CARTESIAN_POINT('Ctrl Pts',(-0.199999999999999,1.02082692352098,
-0.845344163653151));
#61131=CARTESIAN_POINT('Ctrl Pts',(-0.199999999999999,1.02628931308357,
-0.840022463622452));
#61132=CARTESIAN_POINT('Ctrl Pts',(-0.199999999999995,1.03169981019787,
-0.8346507797186));
#61133=CARTESIAN_POINT('Ctrl Pts',(-0.199999999999996,1.03705751954036,
-0.829229435958842));
#61134=CARTESIAN_POINT('Ctrl Pts',(-0.199999999999998,1.07393371359335,
-0.791915257131079));
#61135=CARTESIAN_POINT('Ctrl Pts',(-0.200000000000001,1.10831166419257,
-0.752252087056621));
#61136=CARTESIAN_POINT('Ctrl Pts',(-0.200000000000003,1.14017701794897,
-0.710537394505997));
#61137=CARTESIAN_POINT('Ctrl Pts',(-0.200000000000005,1.15714800209,-0.688320808079979));
#61138=CARTESIAN_POINT('Ctrl Pts',(-0.200000000000006,1.17340579040207,
-0.665521567859066));
#61139=CARTESIAN_POINT('Ctrl Pts',(-0.200000000000005,1.18894441677493,
-0.642180190235135));
#61140=CARTESIAN_POINT('Ctrl Pts',(-0.200000000000005,1.19826943417516,
-0.628172597333051));
#61141=CARTESIAN_POINT('Ctrl Pts',(-0.199999999999999,1.20733539801163,
-0.613969703735576));
#61142=CARTESIAN_POINT('Ctrl Pts',(-0.199999999999999,1.21614051436765,
-0.599579836608104));
#61143=CARTESIAN_POINT('Ctrl Pts',(-0.199999999999999,1.22219283654289,
-0.589688756423258));
#61144=CARTESIAN_POINT('Ctrl Pts',(-0.199999999999997,1.22812251980414,
-0.579707981684439));
#61145=CARTESIAN_POINT('Ctrl Pts',(-0.199999999999997,1.23391867616795,
-0.569658683741284));
#61146=CARTESIAN_POINT('Ctrl Pts',(-0.199999999999996,1.2613223359756,-0.522146586956005));
#61147=CARTESIAN_POINT('Ctrl Pts',(-0.199999999999998,1.28580053533619,
-0.473016095229739));
#61148=CARTESIAN_POINT('Ctrl Pts',(-0.199999999999998,1.30735107827001,
-0.422603250496398));
#61149=CARTESIAN_POINT('Ctrl Pts',(-0.199999999999998,1.32936794320409,
-0.371099546072548));
#61150=CARTESIAN_POINT('Ctrl Pts',(-0.200000000000001,1.34832961329657,
-0.318256565595133));
#61151=CARTESIAN_POINT('Ctrl Pts',(-0.200000000000001,1.36419558884076,
-0.264393162206011));
#61152=CARTESIAN_POINT('Ctrl Pts',(-0.200000000000001,1.37307857615403,
-0.234236306888627));
#61153=CARTESIAN_POINT('Ctrl Pts',(-0.200000000000008,1.38099045666224,
-0.203758954279961));
#61154=CARTESIAN_POINT('Ctrl Pts',(-0.200000000000009,1.38791810504401,
-0.173013380822985));
#61155=CARTESIAN_POINT('Ctrl Pts',(-0.200000000000009,1.39266339253719,
-0.151953336034936));
#61156=CARTESIAN_POINT('Ctrl Pts',(-0.200000000000011,1.3969467919497,-0.130767392506577));
#61157=CARTESIAN_POINT('Ctrl Pts',(-0.200000000000013,1.40076280465425,
-0.109471897823214));
#61158=CARTESIAN_POINT('Ctrl Pts',(-0.200000000000014,1.40337099863038,
-0.0949167101830787));
#61159=CARTESIAN_POINT('Ctrl Pts',(-0.199999999999992,1.40576157137632,
-0.0803042164079611));
#61160=CARTESIAN_POINT('Ctrl Pts',(-0.199999999999993,1.40792789131239,
-0.0656738373046273));
#61161=CARTESIAN_POINT('Ctrl Pts',(-0.199999999999995,1.41645918627998,
-0.00805719557944552));
#61162=CARTESIAN_POINT('Ctrl Pts',(-0.200000000000006,1.42153315207724,
0.0499141617019763));
#61163=CARTESIAN_POINT('Ctrl Pts',(-0.200000000000005,1.42311910879787,
0.107898749183097));
#61164=CARTESIAN_POINT('Ctrl Pts',(-0.200000000000003,1.42476833679356,
0.168196614660305));
#61165=CARTESIAN_POINT('Ctrl Pts',(-0.199999999999996,1.42264651610737,
0.22850989730486));
#61166=CARTESIAN_POINT('Ctrl Pts',(-0.199999999999997,1.41666493374304,
0.28847860395704));
#61167=CARTESIAN_POINT('Ctrl Pts',(-0.199999999999998,1.41105131042735,
0.344758315473251));
#61168=CARTESIAN_POINT('Ctrl Pts',(-0.199999999999995,1.40203806422657,
0.400735686869312));
#61169=CARTESIAN_POINT('Ctrl Pts',(-0.199999999999995,1.38950159942899,
0.456116958127017));
#61170=CARTESIAN_POINT('Ctrl Pts',(-0.199999999999995,1.38867986533664,
0.459747062738241));
#61171=CARTESIAN_POINT('Ctrl Pts',(-0.2,1.38784297517085,0.463374604186691));
#61172=CARTESIAN_POINT('Ctrl Pts',(-0.2,1.38699088616441,0.466999498604503));
#61173=CARTESIAN_POINT('',(-0.2,-1.79227059055215E-16,1.4635));
#61174=CARTESIAN_POINT('Origin',(-0.2,0.,0.));
#61175=CARTESIAN_POINT('',(-0.2,0.501864481801965,1.37604662611724));
#61176=CARTESIAN_POINT('Origin',(-0.2,0.,0.));
#61177=CARTESIAN_POINT('Ctrl Pts',(-0.2,0.50202173509711,1.37727613462792));
#61178=CARTESIAN_POINT('Ctrl Pts',(-0.2,0.467209610033743,1.38655883583692));
#61179=CARTESIAN_POINT('Ctrl Pts',(-0.199999999999991,0.432087726974528,
1.39445148143947));
#61180=CARTESIAN_POINT('Ctrl Pts',(-0.199999999999991,0.396707563583374,
1.40089474981437));
#61181=CARTESIAN_POINT('Ctrl Pts',(-0.19999999999999,0.33987401238208,1.41124500792484));
#61182=CARTESIAN_POINT('Ctrl Pts',(-0.200000000000006,0.282373290930486,
1.417857743763));
#61183=CARTESIAN_POINT('Ctrl Pts',(-0.200000000000005,0.224536309947567,
1.42084361738228));
#61184=CARTESIAN_POINT('Ctrl Pts',(-0.200000000000004,0.194463123061523,
1.42239616618141));
#61185=CARTESIAN_POINT('Ctrl Pts',(-0.2,0.164299125551568,1.42296729002729));
#61186=CARTESIAN_POINT('Ctrl Pts',(-0.199999999999999,0.134092360305547,
1.42256735698774));
#61187=CARTESIAN_POINT('Ctrl Pts',(-0.199999999999998,0.121186218285078,
1.42239648160386));
#61188=CARTESIAN_POINT('Ctrl Pts',(-0.199999999999994,0.108271378161479,
1.42204813448602));
#61189=CARTESIAN_POINT('Ctrl Pts',(-0.199999999999994,0.0953682127448282,
1.42152399163123));
#61190=CARTESIAN_POINT('Ctrl Pts',(-0.199999999999996,0.0378376022185237,
1.41918702566471));
#61191=CARTESIAN_POINT('Ctrl Pts',(-0.200000000000007,-0.0195396042662414,
1.41335923195479));
#61192=CARTESIAN_POINT('Ctrl Pts',(-0.200000000000003,-0.0764338051951725,
1.40414978072417));
#61193=CARTESIAN_POINT('Ctrl Pts',(-0.2,-0.114252001240382,1.39802815802059));
#61194=CARTESIAN_POINT('Ctrl Pts',(-0.199999999999994,-0.15185661385594,
1.39041128430496));
#61195=CARTESIAN_POINT('Ctrl Pts',(-0.199999999999992,-0.189145373564116,
1.38131971234083));
#61196=CARTESIAN_POINT('Ctrl Pts',(-0.199999999999991,-0.204522753083807,
1.37757047118567));
#61197=CARTESIAN_POINT('Ctrl Pts',(-0.199999999999998,-0.219846350113962,
1.37357033828829));
#61198=CARTESIAN_POINT('Ctrl Pts',(-0.199999999999998,-0.235108670748314,
1.36932034708906));
#61199=CARTESIAN_POINT('Ctrl Pts',(-0.199999999999998,-0.248545656240996,
1.36557864414255));
#61200=CARTESIAN_POINT('Ctrl Pts',(-0.199999999999987,-0.261938666183503,
1.3616420272537));
#61201=CARTESIAN_POINT('Ctrl Pts',(-0.199999999999987,-0.275257297963859,
1.35751930035212));
#61202=CARTESIAN_POINT('Ctrl Pts',(-0.199999999999989,-0.329002504954751,
1.34088269575589));
#61203=CARTESIAN_POINT('Ctrl Pts',(-0.2,-0.381618224871022,1.32119875338036));
#61204=CARTESIAN_POINT('Ctrl Pts',(-0.200000000000001,-0.432796645025925,
1.29856457497461));
#61205=CARTESIAN_POINT('Ctrl Pts',(-0.200000000000002,-0.482685261313613,
1.27650082548696));
#61206=CARTESIAN_POINT('Ctrl Pts',(-0.200000000000003,-0.531208941724398,
1.25163303504481));
#61207=CARTESIAN_POINT('Ctrl Pts',(-0.200000000000002,-0.57805281350073,
1.22401270646073));
#61208=CARTESIAN_POINT('Ctrl Pts',(-0.200000000000002,-0.605369225972023,
1.20790626052479));
#61209=CARTESIAN_POINT('Ctrl Pts',(-0.199999999999991,-0.632113797838164,
1.19086314281957));
#61210=CARTESIAN_POINT('Ctrl Pts',(-0.199999999999989,-0.658217585593046,
1.17288853171812));
#61211=CARTESIAN_POINT('Ctrl Pts',(-0.199999999999988,-0.675175610796268,
1.16121153254318));
#61212=CARTESIAN_POINT('Ctrl Pts',(-0.199999999999995,-0.691863102147501,
1.14914134267626));
#61213=CARTESIAN_POINT('Ctrl Pts',(-0.199999999999995,-0.708259846095076,
1.13667865309989));
#61214=CARTESIAN_POINT('Ctrl Pts',(-0.199999999999994,-0.718423561459792,
1.12895350779433));
#61215=CARTESIAN_POINT('Ctrl Pts',(-0.200000000000005,-0.72847844599448,
1.12107500079026));
#61216=CARTESIAN_POINT('Ctrl Pts',(-0.200000000000005,-0.738398879101225,
1.11306041296684));
#61217=CARTESIAN_POINT('Ctrl Pts',(-0.200000000000004,-0.779407630315877,
1.07992998059534));
#61218=CARTESIAN_POINT('Ctrl Pts',(-0.199999999999987,-0.818192292478104,
1.04442585590619));
#61219=CARTESIAN_POINT('Ctrl Pts',(-0.199999999999988,-0.854466407805115,
1.00660336811821));
#61220=CARTESIAN_POINT('Ctrl Pts',(-0.199999999999988,-0.860634784543826,
1.00017169220363));
#61221=CARTESIAN_POINT('Ctrl Pts',(-0.199999999999995,-0.866730468954246,
0.993672901300179));
#61222=CARTESIAN_POINT('Ctrl Pts',(-0.199999999999996,-0.872751928881112,
0.987107177684735));
#61223=CARTESIAN_POINT('Ctrl Pts',(-0.2,-0.908388068815388,0.94824998219203));
#61224=CARTESIAN_POINT('Ctrl Pts',(-0.200000000000001,-0.941428229725658,
0.907049875606388));
#61225=CARTESIAN_POINT('Ctrl Pts',(-0.2,-0.971787759829015,0.863805062866217));
#61226=CARTESIAN_POINT('Ctrl Pts',(-0.199999999999999,-0.986409690306514,
0.842977248889962));
#61227=CARTESIAN_POINT('Ctrl Pts',(-0.2,-1.00040912668513,0.821674881056962));
#61228=CARTESIAN_POINT('Ctrl Pts',(-0.2,-1.01377269674601,0.799930439499796));
#61229=CARTESIAN_POINT('Ctrl Pts',(-0.2,-1.02415577823187,0.783035679527426));
#61230=CARTESIAN_POINT('Ctrl Pts',(-0.200000000000001,-1.03415494874593,
0.765874035875678));
#61231=CARTESIAN_POINT('Ctrl Pts',(-0.2,-1.04376284041761,0.748460746768354));
#61232=CARTESIAN_POINT('Ctrl Pts',(-0.2,-1.04834541507807,0.740155314094317));
#61233=CARTESIAN_POINT('Ctrl Pts',(-0.199999999999998,-1.05283734842709,
0.731795409508619));
#61234=CARTESIAN_POINT('Ctrl Pts',(-0.199999999999997,-1.05723350309492,
0.72339177859167));
#61235=CARTESIAN_POINT('Ctrl Pts',(-0.199999999999995,-1.08157589449212,
0.676859186270714));
#61236=CARTESIAN_POINT('Ctrl Pts',(-0.199999999999994,-1.10302971579605,
0.628908125843251));
#61237=CARTESIAN_POINT('Ctrl Pts',(-0.199999999999993,-1.12153136716694,
0.579842458254082));
#61238=CARTESIAN_POINT('Ctrl Pts',(-0.199999999999993,-1.13995375954158,
0.530986982473522));
#61239=CARTESIAN_POINT('Ctrl Pts',(-0.199999999999998,-1.15544931532854,
0.481025232927459));
#61240=CARTESIAN_POINT('Ctrl Pts',(-0.2,-1.16790446064798,0.430251413185659));
#61241=CARTESIAN_POINT('Ctrl Pts',(-0.200000000000002,-1.17443020194359,
0.403649008819676));
#61242=CARTESIAN_POINT('Ctrl Pts',(-0.2,-1.18012045949723,0.376823695199568));
#61243=CARTESIAN_POINT('Ctrl Pts',(-0.200000000000001,-1.18495316181998,
0.349818803045841));
#61244=CARTESIAN_POINT('Ctrl Pts',(-0.200000000000001,-1.18825456893228,
0.33137070981168));
#61245=CARTESIAN_POINT('Ctrl Pts',(-0.199999999999997,-1.19115569092218,
0.312838829634385));
#61246=CARTESIAN_POINT('Ctrl Pts',(-0.199999999999997,-1.19364840917177,
0.294237378020598));
#61247=CARTESIAN_POINT('Ctrl Pts',(-0.199999999999996,-1.19498882449599,
0.284234775119132));
#61248=CARTESIAN_POINT('Ctrl Pts',(-0.199999999999996,-1.19621114658957,
0.274210923601008));
#61249=CARTESIAN_POINT('Ctrl Pts',(-0.199999999999996,-1.19731245520782,
0.264185232341623));
#61250=CARTESIAN_POINT('Ctrl Pts',(-0.199999999999996,-1.20281983502613,
0.214049158954717));
#61251=CARTESIAN_POINT('Ctrl Pts',(-0.200000000000007,-1.20531936750276,
0.163767737011937));
#61252=CARTESIAN_POINT('Ctrl Pts',(-0.200000000000006,-1.2047212293548,
0.113609796366066));
#61253=CARTESIAN_POINT('Ctrl Pts',(-0.200000000000005,-1.20413275350728,
0.0642621051471473));
#61254=CARTESIAN_POINT('Ctrl Pts',(-0.200000000000007,-1.20054580644529,
0.0150329753455555));
#61255=CARTESIAN_POINT('Ctrl Pts',(-0.200000000000009,-1.19382633959115,
-0.0338080607322077));
#61256=CARTESIAN_POINT('Ctrl Pts',(-0.200000000000011,-1.18710687273702,
-0.0826490968099709));
#61257=CARTESIAN_POINT('Ctrl Pts',(-0.200000000000001,-1.17725493947779,
-0.131102982562808));
#61258=CARTESIAN_POINT('Ctrl Pts',(-0.2,-1.1640875192389,-0.178872328917063));
#61259=CARTESIAN_POINT('Ctrl Pts',(-34.8014778394209,-0.510216505387977,
1.0614961988296));
#61260=CARTESIAN_POINT('Ctrl Pts',(-34.7749632970153,-0.863898086752264,
0.891496362124812));
#61261=CARTESIAN_POINT('Ctrl Pts',(-34.7219342122039,-1.38177714701916,
0.173082322994189));
#61262=CARTESIAN_POINT('Ctrl Pts',(-34.6423905849868,-0.891720964097157,
-1.07138127409762));
#61263=CARTESIAN_POINT('Ctrl Pts',(-34.5628469577698,0.41872224072349,-1.32812088037402));
#61264=CARTESIAN_POINT('Ctrl Pts',(-34.4833033305527,1.34388692616717,-0.366485362373245));
#61265=CARTESIAN_POINT('Ctrl Pts',(-34.4037597033356,1.03476789300364,0.932740929113639));
#61266=CARTESIAN_POINT('Ctrl Pts',(-34.3242160761186,-0.225138742279001,
1.37459976780186));
#61267=CARTESIAN_POINT('Ctrl Pts',(-34.2446724489015,-1.27812685049181,
0.55389298243285));
#61268=CARTESIAN_POINT('Ctrl Pts',(-34.1651288216845,-1.1569721580061,-0.775796455775922));
#61269=CARTESIAN_POINT('Ctrl Pts',(-34.0855851944674,0.0270938664892442,
-1.39270766067608));
#61270=CARTESIAN_POINT('Ctrl Pts',(-34.0060415672503,1.18625641663401,-0.730203319351427));
#61271=CARTESIAN_POINT('Ctrl Pts',(-33.9264979400333,1.25563603260232,0.603143373819632));
#61272=CARTESIAN_POINT('Ctrl Pts',(-33.8469543128163,0.171484699201278,
1.3823842729852));
#61273=CARTESIAN_POINT('Ctrl Pts',(-33.7674106855991,-1.07020426635795,
0.891662136491004));
#61274=CARTESIAN_POINT('Ctrl Pts',(-33.6878670583821,-1.32871925846032,
-0.418214763006971));
#61275=CARTESIAN_POINT('Ctrl Pts',(-33.6083234311651,-0.366566277470248,
-1.34388474473925));
#61276=CARTESIAN_POINT('Ctrl Pts',(-33.528779803948,0.932343436689741,-1.03495583798244));
#61277=CARTESIAN_POINT('Ctrl Pts',(-33.4492361767309,1.37472827927823,0.224766432947515));
#61278=CARTESIAN_POINT('Ctrl Pts',(-33.3696925495139,0.554178040687849,
1.2780001196717));
#61279=CARTESIAN_POINT('Ctrl Pts',(-33.2901489222968,-0.775484290456672,
1.15716111629985));
#61280=CARTESIAN_POINT('Ctrl Pts',(-33.2106052950798,-1.39272494414946,
-0.0267384097234227));
#61281=CARTESIAN_POINT('Ctrl Pts',(-33.1310616678627,-0.730497410775578,
-1.1860738687982));
#61282=CARTESIAN_POINT('Ctrl Pts',(-33.0515180406456,0.602823280911789,
-1.25578732295739));
#61283=CARTESIAN_POINT('Ctrl Pts',(-32.9719744134286,1.38234244666654,-0.171834409267923));
#61284=CARTESIAN_POINT('Ctrl Pts',(-32.8924307862115,0.891931624897046,
1.06997928849094));
#61285=CARTESIAN_POINT('Ctrl Pts',(-32.8128871589945,-0.417878700488076,
1.32882470468588));
#61286=CARTESIAN_POINT('Ctrl Pts',(-32.7333435317774,-1.34379233452526,
0.366905798459168));
#61287=CARTESIAN_POINT('Ctrl Pts',(-32.6537999045604,-1.03519118905535,
-0.932082027005969));
#61288=CARTESIAN_POINT('Ctrl Pts',(-32.5742562773433,0.224419118509842,
-1.37478498777756));
#61289=CARTESIAN_POINT('Ctrl Pts',(-32.4947126501262,1.27786013090699,-0.554500846765326));
#61290=CARTESIAN_POINT('Ctrl Pts',(-32.4151690229092,1.15735694303011,0.775191982424803));
#61291=CARTESIAN_POINT('Ctrl Pts',(-32.3356253956921,-0.0263866089456238,
1.39273165043428));
#61292=CARTESIAN_POINT('Ctrl Pts',(-32.2560817684751,-1.18588931814518,
0.730796981615063));
#61293=CARTESIAN_POINT('Ctrl Pts',(-32.1765381412579,-1.25593954855088,
-0.602506061058643));
#61294=CARTESIAN_POINT('Ctrl Pts',(-32.096994514041,-0.172183573404041,
-1.38229899814921));
#61295=CARTESIAN_POINT('Ctrl Pts',(-32.0174508868238,1.06975396049637,-0.892201864620813));
#61296=CARTESIAN_POINT('Ctrl Pts',(-31.9379072596068,1.3289302146337,0.417543037140155));
#61297=CARTESIAN_POINT('Ctrl Pts',(-31.8583636323897,0.367245217795309,
1.34369961421373));
#61298=CARTESIAN_POINT('Ctrl Pts',(-31.7788200051727,-0.931820516628637,
1.03542659228985));
#61299=CARTESIAN_POINT('Ctrl Pts',(-31.6992763779556,-1.37484163028206,
-0.224071852035116));
#61300=CARTESIAN_POINT('Ctrl Pts',(-31.6197327507386,-0.554823606020508,
-1.27772002779702));
#61301=CARTESIAN_POINT('Ctrl Pts',(-31.5401891235215,0.774899618904291,
-1.1575527132071));
#61302=CARTESIAN_POINT('Ctrl Pts',(-31.4606454963045,1.39273827103593,0.0260348155934577));
#61303=CARTESIAN_POINT('Ctrl Pts',(-31.3811018690874,0.73109650415408,1.18570468702998));
#61304=CARTESIAN_POINT('Ctrl Pts',(-31.3015582418703,-0.602188801882199,
1.25609169654084));
#61305=CARTESIAN_POINT('Ctrl Pts',(-31.2220146146532,-1.38225546190224,
0.172532725222116));
#61306=CARTESIAN_POINT('Ctrl Pts',(-31.1424709874362,-0.892472047174996,
-1.06952856354678));
#61307=CARTESIAN_POINT('Ctrl Pts',(-31.0629273602191,0.417207347022933,
-1.32903564016216));
#61308=CARTESIAN_POINT('Ctrl Pts',(-30.9833837330021,1.34360680823865,-0.367584613505395));
#61309=CARTESIAN_POINT('Ctrl Pts',(-30.903840105785,1.03566192942565,0.931558946696078));
#61310=CARTESIAN_POINT('Ctrl Pts',(-30.824296478568,-0.223724571245162,
1.3748981851222));
#61311=CARTESIAN_POINT('Ctrl Pts',(-30.7447528513509,-1.27757984317515,
0.555146329848009));
#61312=CARTESIAN_POINT('Ctrl Pts',(-30.6652092241338,-1.15774840952399,
-0.774607205928161));
#61313=CARTESIAN_POINT('Ctrl Pts',(-30.5856655969168,0.0256830205774446,
-1.39274480278519));
#61314=CARTESIAN_POINT('Ctrl Pts',(-30.5061219696997,1.18551998026519,-0.731395980043076));
#61315=CARTESIAN_POINT('Ctrl Pts',(-30.4265783424827,1.25624376438813,0.601871504282349));
#61316=CARTESIAN_POINT('Ctrl Pts',(-30.3470347152656,0.172881866032571,
1.38221183746495));
#61317=CARTESIAN_POINT('Ctrl Pts',(-30.2674910880486,-1.0693030983587,0.892742172786554));
#61318=CARTESIAN_POINT('Ctrl Pts',(-30.1879474608315,-1.3291409808946,-0.416871630286474));
#61319=CARTESIAN_POINT('Ctrl Pts',(-30.1084038336144,-0.367923985762689,
-1.34351391653814));
#61320=CARTESIAN_POINT('Ctrl Pts',(-30.0288602063974,0.931297317327677,
-1.03589720048344));
#61321=CARTESIAN_POINT('Ctrl Pts',(-29.9493165791803,1.37495465224026,0.223377276180953));
#61322=CARTESIAN_POINT('Ctrl Pts',(-29.8697729519633,0.555469018255743,
1.2774395770404));
#61323=CARTESIAN_POINT('Ctrl Pts',(-29.7902293247462,-0.774314743530089,
1.15794403197352));
#61324=CARTESIAN_POINT('Ctrl Pts',(-29.7106856975291,-1.39275124567373,
-0.02533122392278));
#61325=CARTESIAN_POINT('Ctrl Pts',(-29.6311420703121,-0.731695409267114,
-1.18533519786117));
#61326=CARTESIAN_POINT('Ctrl Pts',(-29.551598443095,0.601554168281548,-1.25639575208381));
#61327=CARTESIAN_POINT('Ctrl Pts',(-29.4720548158779,1.38216812483898,-0.173230995812698));
#61328=CARTESIAN_POINT('Ctrl Pts',(-29.3925111886609,0.893012241438832,
1.06907756494632));
#61329=CARTESIAN_POINT('Ctrl Pts',(-29.3129675614438,-0.416535886952527,
1.3292462368244));
#61330=CARTESIAN_POINT('Ctrl Pts',(-29.2334239342268,-1.34342093911796,
0.368263334545493));
#61331=CARTESIAN_POINT('Ctrl Pts',(-29.1538803070097,-1.03613240544832,
-0.93103562854009));
#61332=CARTESIAN_POINT('Ctrl Pts',(-29.0743366797926,0.223029966864688,
-1.37501103163265));
#61333=CARTESIAN_POINT('Ctrl Pts',(-28.9947930525756,1.27729922940169,-0.555791671223127));
#61334=CARTESIAN_POINT('Ctrl Pts',(-28.9152494253585,1.15813958054323,0.774022231728725));
#61335=CARTESIAN_POINT('Ctrl Pts',(-28.8357057981415,-0.0249794256519103,
1.39275759970113));
#61336=CARTESIAN_POINT('Ctrl Pts',(-28.7561621709244,-1.18515033982969,
0.7319947918071));
#61337=CARTESIAN_POINT('Ctrl Pts',(-28.6766185437074,-1.2565476596182,-0.601236793900022));
#61338=CARTESIAN_POINT('Ctrl Pts',(-28.5970749164903,-0.173580114540252,
-1.38212432402709));
#61339=CARTESIAN_POINT('Ctrl Pts',(-28.5175312892732,1.06885196332402,-0.893282253114629));
#61340=CARTESIAN_POINT('Ctrl Pts',(-28.4379876620562,1.32935140794485,0.416200117042506));
#61341=CARTESIAN_POINT('Ctrl Pts',(-28.3584440348391,0.36860265983214,1.34332787598405));
#61342=CARTESIAN_POINT('Ctrl Pts',(-28.278900407622,-0.930773880350019,
1.03636754430526));
#61343=CARTESIAN_POINT('Ctrl Pts',(-28.199356780405,-1.37506732329578,-0.222682643318531));
#61344=CARTESIAN_POINT('Ctrl Pts',(-28.1198131531879,-0.556114288729563,
-1.27715880026799));
#61345=CARTESIAN_POINT('Ctrl Pts',(-28.0402695259709,0.773729670542738,
-1.15833505522063));
#61346=CARTESIAN_POINT('Ctrl Pts',(-27.9607258987538,1.39276386486699,0.0246276257872868));
#61347=CARTESIAN_POINT('Ctrl Pts',(-27.8811822715368,0.732294127643924,
1.18496540618255));
#61348=CARTESIAN_POINT('Ctrl Pts',(-27.8016386443197,-0.600919381158034,
1.25669948698159));
#61349=CARTESIAN_POINT('Ctrl Pts',(-27.7220950171026,-1.3820804350321,0.173929222192942));
#61350=CARTESIAN_POINT('Ctrl Pts',(-27.6425513898856,-0.893552207796699,
-1.06862629350621));
#61351=CARTESIAN_POINT('Ctrl Pts',(-27.5630077626685,0.415864320577861,
-1.32945649424924));
#61352=CARTESIAN_POINT('Ctrl Pts',(-27.4834641354515,1.34323472714235,-0.368941961600966));
#61353=CARTESIAN_POINT('Ctrl Pts',(-27.4039205082344,1.03660261703927,0.930512072774181));
#61354=CARTESIAN_POINT('Ctrl Pts',(-27.3243768810174,-0.222335305564666,
1.37512352722605));
#61355=CARTESIAN_POINT('Ctrl Pts',(-27.2448332538003,-1.27701828964825,
0.556436870754451));
#61356=CARTESIAN_POINT('Ctrl Pts',(-27.1652896265832,-1.15853045599325,
-0.773437059990814));
#61357=CARTESIAN_POINT('Ctrl Pts',(-27.0857459993661,0.0242758243513772,
-1.39277004117091));
#61358=CARTESIAN_POINT('Ctrl Pts',(-27.0062023721491,1.18478039693156,-0.732593416758471));
#61359=CARTESIAN_POINT('Ctrl Pts',(-26.926658744932,1.2568512341643,0.60060193007585));
#61360=CARTESIAN_POINT('Ctrl Pts',(-26.847115117715,0.174278318748489,1.38203645785679));
#61361=CARTESIAN_POINT('Ctrl Pts',(-26.7675714904979,-1.06840055550726,
0.893822105467825));
#61362=CARTESIAN_POINT('Ctrl Pts',(-26.6880278632809,-1.32956149573086,
-0.415528497579976));
#61363=CARTESIAN_POINT('Ctrl Pts',(-26.6084842360638,-0.369281239830358,
-1.34314149259879));
#61364=CARTESIAN_POINT('Ctrl Pts',(-26.5289406088467,0.930250205829247,
-1.03683762363535));
#61365=CARTESIAN_POINT('Ctrl Pts',(-26.4493969816297,1.37517964341989,0.221987953625214));
#61366=CARTESIAN_POINT('Ctrl Pts',(-26.3698533544126,0.556759417277243,
1.27687769755144));
#61367=CARTESIAN_POINT('Ctrl Pts',(-26.2903097271956,-0.773144400091584,
1.15872578284863));
#61368=CARTESIAN_POINT('Ctrl Pts',(-26.2107660999785,-1.39277612861249,
-0.0239240213665873));
#61369=CARTESIAN_POINT('Ctrl Pts',(-26.1312224727615,-0.732892659131677,
-1.1845953120885));
#61370=CARTESIAN_POINT('Ctrl Pts',(-26.0516788455444,0.600284440673691,
-1.25700290115665));
#61371=CARTESIAN_POINT('Ctrl Pts',(-25.9721352183273,1.38199239250399,-0.174627404184641));
#61372=CARTESIAN_POINT('Ctrl Pts',(-25.8925915911103,0.894091946110794,
1.06817474934159));
#61373=CARTESIAN_POINT('Ctrl Pts',(-25.8130479638932,-0.415192648070296,
1.32966641238302));
#61374=CARTESIAN_POINT('Ctrl Pts',(-25.7335043366761,-1.34304817235933,
0.369620494498651));
#61375=CARTESIAN_POINT('Ctrl Pts',(-25.6539607094591,-1.03707256407851,
-0.929988279531947));
#61376=CARTESIAN_POINT('Ctrl Pts',(-25.574417082242,0.221640587522368,-1.3752356718737));
#61377=CARTESIAN_POINT('Ctrl Pts',(-25.494873455025,1.27673702398653,-0.557081928277323));
#61378=CARTESIAN_POINT('Ctrl Pts',(-25.4153298278079,1.1589210357743,0.772851690863756));
#61379=CARTESIAN_POINT('Ctrl Pts',(-25.3357862005909,-0.0235722168554084,
1.39278212719136));
#61380=CARTESIAN_POINT('Ctrl Pts',(-25.2562425733738,-1.18441015166521,
0.733191854744411));
#61381=CARTESIAN_POINT('Ctrl Pts',(-25.1766989461567,-1.25715448794894,
-0.599966912971858));
#61382=CARTESIAN_POINT('Ctrl Pts',(-25.0971553189397,-0.174976478479087,
-1.38194823897649));
#61383=CARTESIAN_POINT('Ctrl Pts',(-25.0176116917226,1.06794887502363,-0.894361729708357));
#61384=CARTESIAN_POINT('Ctrl Pts',(-24.9380680645055,1.32977124419901,0.414856772070276));
#61385=CARTESIAN_POINT('Ctrl Pts',(-24.8585244372885,0.369959725584168,
1.34295476642992));
#61386=CARTESIAN_POINT('Ctrl Pts',(-24.7789808100714,-0.929726293898997,
1.03730743835374));
#61387=CARTESIAN_POINT('Ctrl Pts',(-24.6994371828544,-1.37529161258391,
-0.221293207278282));
#61388=CARTESIAN_POINT('Ctrl Pts',(-24.6198935556373,-0.557404403734147,
-1.27659626896248));
#61389=CARTESIAN_POINT('Ctrl Pts',(-24.5403499284203,0.772558932325985,
-1.15911621475782));
#61390=CARTESIAN_POINT('Ctrl Pts',(-24.4608063012032,1.39278803690711,0.0232204108402372));
#61391=CARTESIAN_POINT('Ctrl Pts',(-24.3812626739862,0.733491003577628,
1.18422491567347));
#61392=CARTESIAN_POINT('Ctrl Pts',(-24.3017190467691,-0.599649346990552,
1.25730599453155));
#61393=CARTESIAN_POINT('Ctrl Pts',(-24.222175419552,-1.38190399727711,0.175325541609601));
#61394=CARTESIAN_POINT('Ctrl Pts',(-24.142631792335,-0.894631456243355,
-1.06772293256774));
#61395=CARTESIAN_POINT('Ctrl Pts',(-24.0630881651179,0.4145208696013,-1.32987599117216));
#61396=CARTESIAN_POINT('Ctrl Pts',(-23.9835445379008,1.34286127481651,-0.370298933065331));
#61397=CARTESIAN_POINT('Ctrl Pts',(-23.9040009106838,1.03754224644608,0.929464248947089));
#61398=CARTESIAN_POINT('Ctrl Pts',(-23.8244572834667,-0.220945812915096,
1.37534746554696));
#61399=CARTESIAN_POINT('Ctrl Pts',(-23.7449136562496,-1.27645543248829,
0.557726843627128));
#61400=CARTESIAN_POINT('Ctrl Pts',(-23.6653700290326,-1.15931131978672,
-0.772266124496938));
#61401=CARTESIAN_POINT('Ctrl Pts',(-23.5858264018155,0.0228686033435479,
-1.39279385775939));
#61402=CARTESIAN_POINT('Ctrl Pts',(-23.5062827745985,1.18403960412511,-0.733790105612224));
#61403=CARTESIAN_POINT('Ctrl Pts',(-23.4267391473814,1.25745742089477,0.599331742750071));
#61404=CARTESIAN_POINT('Ctrl Pts',(-23.3471955201644,0.175674593553903,
1.38185966740868));
#61405=CARTESIAN_POINT('Ctrl Pts',(-23.2676518929473,-1.06749692198837,
0.894901125698542));
#61406=CARTESIAN_POINT('Ctrl Pts',(-23.1881082657303,-1.32998065329578,
-0.41418494068481));
#61407=CARTESIAN_POINT('Ctrl Pts',(-23.1085646385132,-0.370638116920458,
-1.34276769752508));
#61408=CARTESIAN_POINT('Ctrl Pts',(-23.0290210112962,0.929202144692953,
-1.03777698834055));
#61409=CARTESIAN_POINT('Ctrl Pts',(-22.949477384079,1.37540323075928,0.220598404455005));
#61410=CARTESIAN_POINT('Ctrl Pts',(-22.869933756862,0.558049247935703,1.27631451457294));
#61411=CARTESIAN_POINT('Ctrl Pts',(-22.7903901296449,-0.771973267395321,
1.15950635084856));
#61412=CARTESIAN_POINT('Ctrl Pts',(-22.7108465024279,-1.39279958974781,
-0.0225167943877718));
#61413=CARTESIAN_POINT('Ctrl Pts',(-22.6313028752108,-0.734089160829106,
-1.18385421703197));
#61414=CARTESIAN_POINT('Ctrl Pts',(-22.5517592479938,0.59901410027068,-1.25760876702895));
#61415=CARTESIAN_POINT('Ctrl Pts',(-22.4722156207767,1.38181524937403,-0.176023634289684));
#61416=CARTESIAN_POINT('Ctrl Pts',(-22.3926719935596,0.89517073805671,1.06727084329994));
#61417=CARTESIAN_POINT('Ctrl Pts',(-22.3131283663426,-0.413848985342271,
1.33008523056319));
#61418=CARTESIAN_POINT('Ctrl Pts',(-22.2335847391255,-1.3426740345616,0.370977277127896));
#61419=CARTESIAN_POINT('Ctrl Pts',(-22.1540411119085,-1.03801166402214,
-0.92893998115333));
#61420=CARTESIAN_POINT('Ctrl Pts',(-22.0744974846914,0.220250981920178,
-1.37545890821731));
#61421=CARTESIAN_POINT('Ctrl Pts',(-21.9949538574744,1.27617351522542,-0.558371616639268));
#61422=CARTESIAN_POINT('Ctrl Pts',(-21.9154102302573,1.15970130793088,0.771680361039824));
#61423=CARTESIAN_POINT('Ctrl Pts',(-21.8358666030402,-0.0221649839953902,
1.39280523287201));
#61424=CARTESIAN_POINT('Ctrl Pts',(-21.7563229758232,-1.18366875440587,
0.734388169209185));
#61425=CARTESIAN_POINT('Ctrl Pts',(-21.6767793486061,-1.25776003292443,
-0.598696419572632));
#61426=CARTESIAN_POINT('Ctrl Pts',(-21.5972357213891,-0.176372663794721,
-1.38177074317598));
#61427=CARTESIAN_POINT('Ctrl Pts',(-21.517692094172,1.06704469651685,-0.895440293300685));
#61428=CARTESIAN_POINT('Ctrl Pts',(-21.4381484669549,1.33018972296772,0.413513003595081));
#61429=CARTESIAN_POINT('Ctrl Pts',(-21.3586048397379,0.371316413666049,
1.34258028593203));
#61430=CARTESIAN_POINT('Ctrl Pts',(-21.2790612125208,-0.92867775834492,
1.03824627347591));
#61431=CARTESIAN_POINT('Ctrl Pts',(-21.1995175853038,-1.37551449791751,
-0.219903545332743));
#61432=CARTESIAN_POINT('Ctrl Pts',(-21.1199739580867,-0.558693949717291,
-1.27603243445472));
#61433=CARTESIAN_POINT('Ctrl Pts',(-21.0404303308696,0.771387405449101,
-1.15989619102127));
#61434=CARTESIAN_POINT('Ctrl Pts',(-20.9608867036526,1.39281078713163,0.0218131721888098));
#61435=CARTESIAN_POINT('Ctrl Pts',(-20.8813430764355,0.734687130733419,
1.18348321625862));
#61436=CARTESIAN_POINT('Ctrl Pts',(-20.8017994492184,-0.598378700676205,
1.25791121857157));
#61437=CARTESIAN_POINT('Ctrl Pts',(-20.7222558220014,-1.38172614881739,
0.17672168204673));
#61438=CARTESIAN_POINT('Ctrl Pts',(-20.6427121947843,-0.895709791413247,
-1.06681848165356));
#61439=CARTESIAN_POINT('Ctrl Pts',(-20.5631685675673,0.413176995464697,
-1.3302941305027));
#61440=CARTESIAN_POINT('Ctrl Pts',(-20.4836249403502,1.34248645164237,-0.371655526513227));
#61441=CARTESIAN_POINT('Ctrl Pts',(-20.4040813131332,1.03848081668687,0.928415476284475));
#61442=CARTESIAN_POINT('Ctrl Pts',(-20.3245376859161,-0.219556094714919,
1.37556999985631));
#61443=CARTESIAN_POINT('Ctrl Pts',(-20.244994058699,-1.27589127226986,0.559016247149181));
#61444=CARTESIAN_POINT('Ctrl Pts',(-20.165450431482,-1.16009100010727,-0.771094400641886));
#61445=CARTESIAN_POINT('Ctrl Pts',(-20.0859068042649,0.0214613589905084,
-1.39281625252631));
#61446=CARTESIAN_POINT('Ctrl Pts',(-20.0063631770478,1.1832976026021,-0.734986045382691));
#61447=CARTESIAN_POINT('Ctrl Pts',(-19.9268195498308,1.25806232396071,0.598060943601679));
#61448=CARTESIAN_POINT('Ctrl Pts',(-19.8472759226137,0.177070689023417,
1.38168146630109));
#61449=CARTESIAN_POINT('Ctrl Pts',(-19.7677322953967,-1.06659219872449,
0.895979232377189));
#61450=CARTESIAN_POINT('Ctrl Pts',(-19.6881886681796,-1.33039845316146,
-0.412840960972545));
#61451=CARTESIAN_POINT('Ctrl Pts',(-19.6086450409626,-0.371994615647838,
-1.3423925316986));
#61452=CARTESIAN_POINT('Ctrl Pts',(-19.5291014137455,0.928153134988703,
-1.03871529364008));
#61453=CARTESIAN_POINT('Ctrl Pts',(-19.4495577865284,1.37562541403019,0.219208630088832));
#61454=CARTESIAN_POINT('Ctrl Pts',(-19.3700141593114,0.55933850891441,1.27575002867982));
#61455=CARTESIAN_POINT('Ctrl Pts',(-19.2904705320943,-0.77080134663684,
1.16028573517647));
#61456=CARTESIAN_POINT('Ctrl Pts',(-19.2109269048773,-1.39282162905571,
-0.0211095444228931));
#61457=CARTESIAN_POINT('Ctrl Pts',(-19.1313832776602,-0.735284913137964,
-1.18311191344811));
#61458=CARTESIAN_POINT('Ctrl Pts',(-19.0518396504431,0.597743148369296,
-1.25821334908223));
#61459=CARTESIAN_POINT('Ctrl Pts',(-18.9722960232261,1.38163669562993,-0.177419684702549));
#61460=CARTESIAN_POINT('Ctrl Pts',(-18.892752396009,0.896248616175358,1.06636584774406));
#61461=CARTESIAN_POINT('Ctrl Pts',(-18.813208768792,-0.412504900140071,
1.33050269093737));
#61462=CARTESIAN_POINT('Ctrl Pts',(-18.7336651415749,-1.3422985261067,0.372333681048236));
#61463=CARTESIAN_POINT('Ctrl Pts',(-18.6541215143579,-1.03894970432056,
-0.927890734474365));
#61464=CARTESIAN_POINT('Ctrl Pts',(-18.5745778871408,0.21886115147667,-1.37568074043561));
#61465=CARTESIAN_POINT('Ctrl Pts',(-18.4950342599237,1.27560870369364,-0.55966073499237));
#61466=CARTESIAN_POINT('Ctrl Pts',(-18.4154906327066,1.16048039621642,0.770508243452683));
#61467=CARTESIAN_POINT('Ctrl Pts',(-18.3359470054896,-0.0207577285084573,
1.39282691671949));
#61468=CARTESIAN_POINT('Ctrl Pts',(-18.2564033782725,-1.18292614880853,
0.735583733980142));
#61469=CARTESIAN_POINT('Ctrl Pts',(-18.1768597510555,-1.25836429392647,
-0.597425314999374));
#61470=CARTESIAN_POINT('Ctrl Pts',(-18.0973161238384,-0.177768669061831,
-1.38159183680678));
#61471=CARTESIAN_POINT('Ctrl Pts',(-18.0177724966214,1.06613942872675,-0.896517942790525));
#61472=CARTESIAN_POINT('Ctrl Pts',(-17.9382288694043,1.33060684382376,0.412168812988731));
#61473=CARTESIAN_POINT('Ctrl Pts',(-17.8586852421873,0.372672722692757,
1.34220443487269));
#61474=CARTESIAN_POINT('Ctrl Pts',(-17.7791416149702,-0.927628274758204,
1.03918404871335));
#61475=CARTESIAN_POINT('Ctrl Pts',(-17.6995979877531,-1.37573597906903,
-0.218513658900598));
#61476=CARTESIAN_POINT('Ctrl Pts',(-17.6200543605361,-0.559982925362541,
-1.27546729732031));
#61477=CARTESIAN_POINT('Ctrl Pts',(-17.540510733319,0.770215091108087,-1.16067498321473));
#61478=CARTESIAN_POINT('Ctrl Pts',(-17.460967106102,1.39283211551731,0.0204059112696104));
#61479=CARTESIAN_POINT('Ctrl Pts',(-17.3814234788849,0.735882507890194,
1.18274030869519));
#61480=CARTESIAN_POINT('Ctrl Pts',(-17.3018798516679,-0.597107443512156,
1.25851515848381));
#61481=CARTESIAN_POINT('Ctrl Pts',(-17.2223362244507,-1.38154688983449,
0.178117642079035));
#61482=CARTESIAN_POINT('Ctrl Pts',(-17.1427925972337,-0.896787212205539,
-1.06591294168697));
#61483=CARTESIAN_POINT('Ctrl Pts',(-17.0632489700166,0.411832699539931,
-1.33071091181399));
#61484=CARTESIAN_POINT('Ctrl Pts',(-16.9837053427996,1.34211025800256,-0.373011740559811));
#61485=CARTESIAN_POINT('Ctrl Pts',(-16.9041617155825,1.03941832680352,0.927365755856943));
#61486=CARTESIAN_POINT('Ctrl Pts',(-16.8246180883655,-0.218166152382787,
1.37579112992694));
#61487=CARTESIAN_POINT('Ctrl Pts',(-16.7450744611484,-1.27532580956886,
0.56030508000436));
#61488=CARTESIAN_POINT('Ctrl Pts',(-16.6655308339313,-1.16086949615897,
-0.76992188962178));
#61489=CARTESIAN_POINT('Ctrl Pts',(-16.5859872067143,0.0200540927288029,
-1.39283722544883));
#61490=CARTESIAN_POINT('Ctrl Pts',(-16.5064435794972,1.18255439311996,-0.736181234849029));
#61491=CARTESIAN_POINT('Ctrl Pts',(-16.4268999522802,1.25866594274463,0.596789533927942));
#61492=CARTESIAN_POINT('Ctrl Pts',(-16.3473563250631,0.17846660373185,1.38150185471594));
#61493=CARTESIAN_POINT('Ctrl Pts',(-16.267812697846,-1.0656863866392,0.897056424403193));
#61494=CARTESIAN_POINT('Ctrl Pts',(-16.188269070629,-1.33081489490141,-0.411496559815159));
#61495=CARTESIAN_POINT('Ctrl Pts',(-16.1087254434119,-0.373350734627734,
-1.34201599550232));
#61496=CARTESIAN_POINT('Ctrl Pts',(-16.0291818161949,0.927103177787362,
-1.0396525385761));
#61497=CARTESIAN_POINT('Ctrl Pts',(-15.9496381889778,1.37584619300581,0.217818631945427));
#61498=CARTESIAN_POINT('Ctrl Pts',(-15.8700945617608,0.560627198897243,
1.27518424044833));
#61499=CARTESIAN_POINT('Ctrl Pts',(-15.7905509345437,-0.769628639012477,
1.16106393503672));
#61500=CARTESIAN_POINT('Ctrl Pts',(-15.7110073073266,-1.39284224651372,
-0.019702272908519));
#61501=CARTESIAN_POINT('Ctrl Pts',(-15.6314636801096,-0.736479914837584,
-1.1823684020947));
#61502=CARTESIAN_POINT('Ctrl Pts',(-15.5519200528925,0.596471586267007,
-1.2588166466993));
#61503=CARTESIAN_POINT('Ctrl Pts',(-15.4723764256754,1.38145673145398,-0.178815553998048));
#61504=CARTESIAN_POINT('Ctrl Pts',(-15.3928327984584,0.897325579366346,
1.06545976359786));
#61505=CARTESIAN_POINT('Ctrl Pts',(-15.3132891712414,-0.41116039383583,
1.3309187930794));
#61506=CARTESIAN_POINT('Ctrl Pts',(-15.2337455440242,-1.34192164737798,
0.373689704874937));
#61507=CARTESIAN_POINT('Ctrl Pts',(-15.1542019168072,-1.03988668401616,
-0.926840540566187));
#61508=CARTESIAN_POINT('Ctrl Pts',(-15.0746582895901,0.217471097610649,
-1.37590116830213));
#61509=CARTESIAN_POINT('Ctrl Pts',(-14.9951146623731,1.27504258996775,-0.560949282020663));
#61510=CARTESIAN_POINT('Ctrl Pts',(-14.915571035156,1.16125829983559,0.76933533929888));
#61511=CARTESIAN_POINT('Ctrl Pts',(-14.836027407939,-0.0193504518311904,
1.39284717871167));
#61512=CARTESIAN_POINT('Ctrl Pts',(-14.7564837807219,-1.18218233563127,
0.736778547836819));
#61513=CARTESIAN_POINT('Ctrl Pts',(-14.6769401535049,-1.25896727033822,
-0.596153600549652));
#61514=CARTESIAN_POINT('Ctrl Pts',(-14.5973965262878,-0.179164492855332,
-1.38141152005153));
#61515=CARTESIAN_POINT('Ctrl Pts',(-14.5178528990707,1.06523307257745,-0.897594677077771));
#61516=CARTESIAN_POINT('Ctrl Pts',(-14.4383092718537,1.33102260634132,0.410824201623429));
#61517=CARTESIAN_POINT('Ctrl Pts',(-14.3587656446366,0.37402865127972,1.34182721363559));
#61518=CARTESIAN_POINT('Ctrl Pts',(-14.2792220174196,-0.926577844210213,
1.04012076310873));
#61519=CARTESIAN_POINT('Ctrl Pts',(-14.1996783902025,-1.3759560558124,-0.217123549400712));
#61520=CARTESIAN_POINT('Ctrl Pts',(-14.1201347629855,-0.561271329354032,
-1.27490085813617));
#61521=CARTESIAN_POINT('Ctrl Pts',(-14.0405911357683,0.769041990499703,
-1.16145259054315));
#61522=CARTESIAN_POINT('Ctrl Pts',(-13.9610475085513,1.39285202204237,0.0189986295192388));
#61523=CARTESIAN_POINT('Ctrl Pts',(-13.8815038813343,0.737077133827655,
1.18199619374158));
#61524=CARTESIAN_POINT('Ctrl Pts',(-13.8019602541172,-0.595835576796184,
1.25911781365174));
#61525=CARTESIAN_POINT('Ctrl Pts',(-13.7224166269001,-1.38136622051142,
0.179513420281436));
#61526=CARTESIAN_POINT('Ctrl Pts',(-13.6428729996831,-0.897863717520344,
-1.0650063135924));
#61527=CARTESIAN_POINT('Ctrl Pts',(-13.563329372466,0.410487983199367,-1.33112633468056));
#61528=CARTESIAN_POINT('Ctrl Pts',(-13.483785745249,1.34173269428113,-0.374367573820533));
#61529=CARTESIAN_POINT('Ctrl Pts',(-13.4042421180319,1.04035477583892,0.92631508873616));
#61530=CARTESIAN_POINT('Ctrl Pts',(-13.3246984908148,-0.216775987337669,
1.37601085553309));
#61531=CARTESIAN_POINT('Ctrl Pts',(-13.2451548635978,-1.27475904496258,
0.561593340876897));
#61532=CARTESIAN_POINT('Ctrl Pts',(-13.1656112363807,-1.16164680714707,
-0.768748592633631));
#61533=CARTESIAN_POINT('Ctrl Pts',(-13.0860676091637,0.0186468059951288,
-1.39285677650551));
#61534=CARTESIAN_POINT('Ctrl Pts',(-13.0065239819466,1.18180997643742,-0.737375672791089));
#61535=CARTESIAN_POINT('Ctrl Pts',(-12.9269803547296,1.25926827663031,0.595517515026806));
#61536=CARTESIAN_POINT('Ctrl Pts',(-12.8474367275125,0.179862336254169,
1.38132083283659));
#61537=CARTESIAN_POINT('Ctrl Pts',(-12.7678931002954,-1.0647794866572,0.898132700676888));
#61538=CARTESIAN_POINT('Ctrl Pts',(-12.6883494730784,-1.33122997809048,
-0.410151738585083));
#61539=CARTESIAN_POINT('Ctrl Pts',(-12.6088058458613,-0.374706472475756,
-1.34163808932065));
#61540=CARTESIAN_POINT('Ctrl Pts',(-12.5292622186442,0.926052274160795,
-1.04058872219181));
#61541=CARTESIAN_POINT('Ctrl Pts',(-12.4497185914272,1.37606556746074,0.216428411443782));
#61542=CARTESIAN_POINT('Ctrl Pts',(-12.3701749642101,0.561915316568623,
1.27461715045607));
#61543=CARTESIAN_POINT('Ctrl Pts',(-12.2906313369931,-0.768455145719422,
1.1618409496349));
#61544=CARTESIAN_POINT('Ctrl Pts',(-12.211087709776,-1.39286144210078,-0.0182949812813028));
#61545=CARTESIAN_POINT('Ctrl Pts',(-12.1315440825589,-0.737674164708033,
-1.18162368373076));
#61546=CARTESIAN_POINT('Ctrl Pts',(-12.0520004553419,0.595199415261899,
-1.25941865926429));
#61547=CARTESIAN_POINT('Ctrl Pts',(-11.9724568281248,1.3812753570299,-0.180211240751194));
#61548=CARTESIAN_POINT('Ctrl Pts',(-11.8929132009078,0.898401626530242,
1.06455259178631));
#61549=CARTESIAN_POINT('Ctrl Pts',(-11.8133695736907,-0.409815467802085,
1.33133353656448));
#61550=CARTESIAN_POINT('Ctrl Pts',(-11.7338259464736,-1.34154339876018,
0.375045347223708));
#61551=CARTESIAN_POINT('Ctrl Pts',(-11.6542823192566,-1.04082260215243,
-0.925789400500909));
#61552=CARTESIAN_POINT('Ctrl Pts',(-11.5747386920395,0.216080821741205,
-1.37612019159185));
#61553=CARTESIAN_POINT('Ctrl Pts',(-11.4951950648225,1.27447517462567,-0.562237256408714));
#61554=CARTESIAN_POINT('Ctrl Pts',(-11.4156514376054,1.16203501799428,0.768161649775757));
#61555=CARTESIAN_POINT('Ctrl Pts',(-11.3361078103884,-0.0179431554001853,
1.39286601882789));
#61556=CARTESIAN_POINT('Ctrl Pts',(-11.2565641831713,-1.18143731563344,
0.737972609559454));
#61557=CARTESIAN_POINT('Ctrl Pts',(-11.1770205559542,-1.2595689615441,-0.5948812775217));
#61558=CARTESIAN_POINT('Ctrl Pts',(-11.0974769287372,-0.18056013375031,
-1.38122979309427));
#61559=CARTESIAN_POINT('Ctrl Pts',(-11.0179333015201,1.06432562899421,-0.898670495063273));
#61560=CARTESIAN_POINT('Ctrl Pts',(-10.938389674303,1.33143701009596,0.409479170871799));
#61561=CARTESIAN_POINT('Ctrl Pts',(-10.858846047086,0.375384198042811,1.34144862260576));
#61562=CARTESIAN_POINT('Ctrl Pts',(-10.7793024198689,-0.925526467773234,
1.04105641570588));
#61563=CARTESIAN_POINT('Ctrl Pts',(-10.6997587926519,-1.37617472792294,
-0.215733218252087));
#61564=CARTESIAN_POINT('Ctrl Pts',(-10.6202151654348,-0.562559160376593,
-1.27433311748048));
#61565=CARTESIAN_POINT('Ctrl Pts',(-10.5406715382178,0.767868104821389,
-1.1622290122128));
#61566=CARTESIAN_POINT('Ctrl Pts',(-10.4611279110007,1.39287050668653,0.0175913283742381));
#61567=CARTESIAN_POINT('Ctrl Pts',(-10.3815842837836,0.73827100732634,1.18125087215736));
#61568=CARTESIAN_POINT('Ctrl Pts',(-10.3020406565666,-0.594563101826563,
1.25971918346015));
#61569=CARTESIAN_POINT('Ctrl Pts',(-10.2224970293495,-1.38118414103261,
0.180909015229188));
#61570=CARTESIAN_POINT('Ctrl Pts',(-10.1429534021325,-0.898939306258771,
-1.06409859829537));
#61571=CARTESIAN_POINT('Ctrl Pts',(-10.0634097749154,0.40914284781568,-1.33154039867832));
#61572=CARTESIAN_POINT('Ctrl Pts',(-9.98386614769835,1.34135376086346,-0.375723024911412));
#61573=CARTESIAN_POINT('Ctrl Pts',(-9.90432252048127,1.04129016283722,0.9252634759946));
#61574=CARTESIAN_POINT('Ctrl Pts',(-9.82477889326422,-0.215385600998657,
1.3762291764505));
#61575=CARTESIAN_POINT('Ctrl Pts',(-9.74523526604716,-1.27419097902953,
0.562881028451743));
#61576=CARTESIAN_POINT('Ctrl Pts',(-9.6656916388301,-1.16242293227811,-0.767574510875076));
#61577=CARTESIAN_POINT('Ctrl Pts',(-9.58614801161304,0.0172395002259546,
-1.39287490567643));
#61578=CARTESIAN_POINT('Ctrl Pts',(-9.50660438439598,1.18106435331442,-0.738569357989597));
#61579=CARTESIAN_POINT('Ctrl Pts',(-9.42706075717891,1.25986932500286,0.59424488819676));
#61580=CARTESIAN_POINT('Ctrl Pts',(-9.34751712996187,0.181257885165623,
1.3811384008478));
#61581=CARTESIAN_POINT('Ctrl Pts',(-9.26797350274479,-1.06387149970427,
0.89920806009964));
#61582=CARTESIAN_POINT('Ctrl Pts',(-9.18842987552775,-1.33164370230497,
-0.408806498655169));
#61583=CARTESIAN_POINT('Ctrl Pts',(-9.10888624831068,-0.37606182780791,
-1.34125881353932));
#61584=CARTESIAN_POINT('Ctrl Pts',(-9.02934262109362,0.925000425181733,
-1.04152384353156));
#61585=CARTESIAN_POINT('Ctrl Pts',(-8.94979899387657,1.37628353717109,0.215037970003031));
#61586=CARTESIAN_POINT('Ctrl Pts',(-8.87025536665949,0.563202860613652,
1.27404875928191));
#61587=CARTESIAN_POINT('Ctrl Pts',(-8.79071173944245,-0.767280867955522,
1.16261677817781));
#61588=CARTESIAN_POINT('Ctrl Pts',(-8.71116811222538,-1.39287921579729,
-0.0168876709777203));
#61589=CARTESIAN_POINT('Ctrl Pts',(-8.63162448500833,-0.738867661530245,
-1.1808777591165));
#61590=CARTESIAN_POINT('Ctrl Pts',(-8.55208085779126,0.59392663665258,-1.26001938616266));
#61591=CARTESIAN_POINT('Ctrl Pts',(-8.47253723057421,1.38109257254281,-0.181606743537313));
#61592=CARTESIAN_POINT('Ctrl Pts',(-8.39299360335714,0.899476756568682,
1.06364433323544));
#61593=CARTESIAN_POINT('Ctrl Pts',(-8.3134499761401,-0.408470123411764,
1.33174692096928));
#61594=CARTESIAN_POINT('Ctrl Pts',(-8.23390634892301,-1.3411637806394,0.376400606710692));
#61595=CARTESIAN_POINT('Ctrl Pts',(-8.15436272170597,-1.04175745777397,
-0.924737315351474));
#61596=CARTESIAN_POINT('Ctrl Pts',(-8.0748190944889,0.214690325287459,-1.37633781008121));
#61597=CARTESIAN_POINT('Ctrl Pts',(-7.99527546727185,1.27390645824667,-0.563524656841738));
#61598=CARTESIAN_POINT('Ctrl Pts',(-7.91573184005478,1.16281054989956,0.766987176081464));
#61599=CARTESIAN_POINT('Ctrl Pts',(-7.83618821283773,-0.016535840652032,
1.39288343704887));
#61600=CARTESIAN_POINT('Ctrl Pts',(-7.75664458562066,-1.18069108957553,
0.739165917929196));
#61601=CARTESIAN_POINT('Ctrl Pts',(-7.67710095840361,-1.26016936692994,
-0.593608347214357));
#61602=CARTESIAN_POINT('Ctrl Pts',(-7.59755733118654,-0.181955590322025,
-1.38104665612053));
#61603=CARTESIAN_POINT('Ctrl Pts',(-7.51801370396949,1.06341709890332,-0.899745395648787));
#61604=CARTESIAN_POINT('Ctrl Pts',(-7.43847007675242,1.3318500546647,0.408133722106875));
#61605=CARTESIAN_POINT('Ctrl Pts',(-7.35892644953538,0.376739361598168,
1.34106866216976));
#61606=CARTESIAN_POINT('Ctrl Pts',(-7.2793828223183,-0.92447414652058,1.04199100554956));
#61607=CARTESIAN_POINT('Ctrl Pts',(-7.19983919510125,-1.37639199517741,
-0.214342666874064));
#61608=CARTESIAN_POINT('Ctrl Pts',(-7.12029556788419,-0.563846417115518,
-1.27376407593289));
#61609=CARTESIAN_POINT('Ctrl Pts',(-7.04075194066713,0.766693435271625,
-1.16300424743101));
#61610=CARTESIAN_POINT('Ctrl Pts',(-6.96120831345008,1.39288756943087,0.0161840092713161));
#61611=CARTESIAN_POINT('Ctrl Pts',(-6.88166468623301,0.73946412716746,1.1805043447034));
#61612=CARTESIAN_POINT('Ctrl Pts',(-6.80212105901595,-0.593290019902356,
1.26031926729517));
#61613=CARTESIAN_POINT('Ctrl Pts',(-6.7225774317989,-1.38100065158391,0.182304425497526));
#61614=CARTESIAN_POINT('Ctrl Pts',(-6.64303380458182,-0.900013977322796,
-1.06318979672246));
#61615=CARTESIAN_POINT('Ctrl Pts',(-6.56349017736478,0.407797294762003,
-1.33195310338462));
#61616=CARTESIAN_POINT('Ctrl Pts',(-6.4839465501477,1.34097345813645,-0.377078092448702));
#61617=CARTESIAN_POINT('Ctrl Pts',(-6.40440292293066,1.04222448684345,0.924210918705832));
#61618=CARTESIAN_POINT('Ctrl Pts',(-6.32485929571359,-0.213994994785076,
1.37644609245625));
#61619=CARTESIAN_POINT('Ctrl Pts',(-6.24531566849654,-1.27362161234968,
0.564168141414408));
#61620=CARTESIAN_POINT('Ctrl Pts',(-6.16577204127946,-1.16319787075975,
-0.766399645544771));
#61621=CARTESIAN_POINT('Ctrl Pts',(-6.08622841406241,0.0158321768580185,
-1.39289161294304));
#61622=CARTESIAN_POINT('Ctrl Pts',(-6.00668478684535,1.18031752451205,-0.739762289225985));
#61623=CARTESIAN_POINT('Ctrl Pts',(-5.92714115962829,1.26046908724875,0.592971654736946));
#61624=CARTESIAN_POINT('Ctrl Pts',(-5.84759753241124,0.182653249041503,
1.38095455893587));
#61625=CARTESIAN_POINT('Ctrl Pts',(-5.76805390519417,-1.06296242670733,
0.900282501573585));
#61626=CARTESIAN_POINT('Ctrl Pts',(-5.68851027797711,-1.3320560671225,-0.407460841398637));
#61627=CARTESIAN_POINT('Ctrl Pts',(-5.60896665076006,-0.377416799240644,
-1.34087816854557));
#61628=CARTESIAN_POINT('Ctrl Pts',(-5.52942302354299,0.923947631924043,
-1.0424579016407));
#61629=CARTESIAN_POINT('Ctrl Pts',(-5.44987939632593,1.37650010191426,0.213647309042655));
#61630=CARTESIAN_POINT('Ctrl Pts',(-5.37033576910888,0.564489829717927,
1.27347906750608));
#61631=CARTESIAN_POINT('Ctrl Pts',(-5.29079214189181,-0.76610580691961,
1.16339141987348));
#61632=CARTESIAN_POINT('Ctrl Pts',(-5.21124851467476,-1.39289556758514,
-0.0154803434345617));
#61633=CARTESIAN_POINT('Ctrl Pts',(-5.13170488745769,-0.740060404085762,
-1.1801306290134));
#61634=CARTESIAN_POINT('Ctrl Pts',(-5.05216126024064,0.592653251738383,
-1.26061882678114));
#61635=CARTESIAN_POINT('Ctrl Pts',(-4.97261763302358,1.38090837817934,-0.183002060931766));
#61636=CARTESIAN_POINT('Ctrl Pts',(-4.89307400580652,0.900550968384048,
1.06273498887245));
#61637=CARTESIAN_POINT('Ctrl Pts',(-4.81353037858945,-0.407124362038215,
1.33215894587174));
#61638=CARTESIAN_POINT('Ctrl Pts',(-4.7339867513724,-1.34078279340317,0.377755481952438));
#61639=CARTESIAN_POINT('Ctrl Pts',(-4.65444312415534,-1.04269124992645,
-0.923684286191978));
#61640=CARTESIAN_POINT('Ctrl Pts',(-4.57489949693828,0.213299609668962,
-1.37655402354802));
#61641=CARTESIAN_POINT('Ctrl Pts',(-4.49535586972123,1.27333644141125,-0.564811482005513));
#61642=CARTESIAN_POINT('Ctrl Pts',(-4.41581224250416,1.1635848947598,0.765811919414912));
#61643=CARTESIAN_POINT('Ctrl Pts',(-4.33626861528711,-0.0151285090234098,
1.39289943335687));
#61644=CARTESIAN_POINT('Ctrl Pts',(-4.25672498807004,-1.17994365821935,
0.740358471727794));
#61645=CARTESIAN_POINT('Ctrl Pts',(-4.17718136085298,-1.26076848588279,
-0.592334810927032));
#61646=CARTESIAN_POINT('Ctrl Pts',(-4.09763773363592,-0.183350861145989,
-1.38086210931729));
#61647=CARTESIAN_POINT('Ctrl Pts',(-4.01809410641886,1.06250748323233,-0.900819377736997));
#61648=CARTESIAN_POINT('Ctrl Pts',(-3.9385504792018,1.3322617396258,0.406787856702201));
#61649=CARTESIAN_POINT('Ctrl Pts',(-3.85900685198474,0.378094140562434,
1.34068733271538));
#61650=CARTESIAN_POINT('Ctrl Pts',(-3.77946322476769,-0.923420881526489,
1.04292453168578));
#61651=CARTESIAN_POINT('Ctrl Pts',(-3.69991959755062,-1.37660785735405,
-0.21295189668622));
#61652=CARTESIAN_POINT('Ctrl Pts',(-3.62037597033357,-0.565133098256669,
-1.27319373407426));
#61653=CARTESIAN_POINT('Ctrl Pts',(-3.5408323431165,0.765517983049464,-1.16377829540639));
#61654=CARTESIAN_POINT('Ctrl Pts',(-3.46128871589945,1.39290321025801,0.0147766736470439));
#61655=CARTESIAN_POINT('Ctrl Pts',(-3.38174508868238,0.740656492133029,
1.17975661214186));
#61656=CARTESIAN_POINT('Ctrl Pts',(-3.30220146146532,-0.592016332323219,
1.2609180645441));
#61657=CARTESIAN_POINT('Ctrl Pts',(-3.22265783424827,-1.38081575235259,
0.183699649662051));
#61658=CARTESIAN_POINT('Ctrl Pts',(-3.1431142070312,-0.901087729615471,
-1.06227990980161));
#61659=CARTESIAN_POINT('Ctrl Pts',(-3.06357057981415,0.406451325412254,
-1.33236444837786));
#61660=CARTESIAN_POINT('Ctrl Pts',(-2.98402695259708,1.34059178648789,-0.378432775049564));
#61661=CARTESIAN_POINT('Ctrl Pts',(-2.90448332538003,1.04315774690456,0.923157417945318));
#61662=CARTESIAN_POINT('Ctrl Pts',(-2.82493969816297,-0.212604170117943,
1.37666160332707));
#61663=CARTESIAN_POINT('Ctrl Pts',(-2.74539607094591,-1.2730509455016,0.565454678454453));
#61664=CARTESIAN_POINT('Ctrl Pts',(-2.66585244372885,-1.16397162180588,
-0.765223997848736));
#61665=CARTESIAN_POINT('Ctrl Pts',(-2.58630881651179,0.0144248373372911,
-1.3929068982755));
#61666=CARTESIAN_POINT('Ctrl Pts',(-2.50676518929473,1.17956949077493,-0.740954465306795));
#61667=CARTESIAN_POINT('Ctrl Pts',(-2.42722156207767,1.26106756278956,0.591697815993344));
#61668=CARTESIAN_POINT('Ctrl Pts',(-2.34767793486061,0.184048426393107,
1.38076930720073));
#61669=CARTESIAN_POINT('Ctrl Pts',(-2.26813430764355,-1.06205226847233,
0.901356024168364));
#61670=CARTESIAN_POINT('Ctrl Pts',(-2.18859068042649,-1.33246707235384,
-0.406114768505075));
#61671=CARTESIAN_POINT('Ctrl Pts',(-2.10904705320943,-0.378771384950898,
-1.34049615412855));
#61672=CARTESIAN_POINT('Ctrl Pts',(-2.02950342599237,0.922893894627693,
-1.04339089670334));
#61673=CARTESIAN_POINT('Ctrl Pts',(-1.94995979877531,1.37671526305346,0.21225643214144));
#61674=CARTESIAN_POINT('Ctrl Pts',(-1.87041617155825,0.56577621956083,1.2729080716121));
#61675=CARTESIAN_POINT('Ctrl Pts',(-1.79087254434119,-0.764929958104375,
1.16416488170923));
#61676=CARTESIAN_POINT('Ctrl Pts',(-1.71132891712414,-1.39291050827911,
-0.0140730148512983));
#61677=CARTESIAN_POINT('Ctrl Pts',(-1.63178528990707,-0.74125237059894,
-1.17938226616436));
#61678=CARTESIAN_POINT('Ctrl Pts',(-1.55224166269001,0.591379222800219,
-1.26121703368907));
#61679=CARTESIAN_POINT('Ctrl Pts',(-1.47269803547295,1.3807228481852,-0.18439709057274));
#61680=CARTESIAN_POINT('Ctrl Pts',(-1.3931544082559,0.901624120319131,1.06182436804775));
#61681=CARTESIAN_POINT('Ctrl Pts',(-1.31361078103883,-0.405777918272958,
1.33256997446379));
#61682=CARTESIAN_POINT('Ctrl Pts',(-1.23406715382177,-1.34040094379007,
0.379109281433699));
#61683=CARTESIAN_POINT('Ctrl Pts',(-1.15452352660471,-1.04362301661124,
-0.922629004235279));
#61684=CARTESIAN_POINT('Ctrl Pts',(-1.07497989938766,0.211906852253127,
-1.3767713178738));
#61685=CARTESIAN_POINT('Ctrl Pts',(-0.995436272170595,1.27276858673064,
-0.566093011994411));
#61686=CARTESIAN_POINT('Ctrl Pts',(-0.915892644953538,1.16435148089155,
0.76462692514249));
#61687=CARTESIAN_POINT('Ctrl Pts',(-0.836349017736476,-0.0137086904440423,
1.39293100582981));
#61688=CARTESIAN_POINT('Ctrl Pts',(-0.75680539051942,-1.17921869337341,
0.741518007289884));
#61689=CARTESIAN_POINT('Ctrl Pts',(-0.67726176330236,-1.26132138808091,
-0.590999433913082));
#61690=CARTESIAN_POINT('Ctrl Pts',(-0.597718136085294,-0.184831240778329,
-1.38079239774389));
#61691=CARTESIAN_POINT('Ctrl Pts',(-0.518174508868238,1.06175884240671,
-0.901671642965467));
#61692=CARTESIAN_POINT('Ctrl Pts',(-0.438630881651178,1.33236304935347,
0.405021101276792));
#61693=CARTESIAN_POINT('Ctrl Pts',(-0.35908725443412,0.380047119706207,
1.34111457344272));
#61694=CARTESIAN_POINT('Ctrl Pts',(-0.279543627217059,-0.923604039966345,
1.04221933963793));
#61695=CARTESIAN_POINT('Ctrl Pts',(-0.226514542405686,-1.22368627072144,
0.208991815207804));
#61696=CARTESIAN_POINT('Ctrl Pts',(-0.2,-1.1640875192389,-0.178872328917063));
#61697=CARTESIAN_POINT('Ctrl Pts',(-34.7464852262806,-0.551480035116971,
1.14734422509872));
#61698=CARTESIAN_POINT('Ctrl Pts',(-34.719970683875,-0.933765454838236,
0.963595728282564));
#61699=CARTESIAN_POINT('Ctrl Pts',(-34.6669415990636,-1.49352775050342,
0.187080277793629));
#61700=CARTESIAN_POINT('Ctrl Pts',(-34.5873979718465,-0.963838494838092,
-1.1580287513703));
#61701=CARTESIAN_POINT('Ctrl Pts',(-34.5078543446294,0.452586213068269,
-1.43553205749614));
#61702=CARTESIAN_POINT('Ctrl Pts',(-34.4283107174124,1.45257317513127,-0.396124700743783));
#61703=CARTESIAN_POINT('Ctrl Pts',(-34.3487670901953,1.11845427959544,1.00817593102252));
#61704=CARTESIAN_POINT('Ctrl Pts',(-34.2692234629783,-0.243346736507173,
1.48576990397941));
#61705=CARTESIAN_POINT('Ctrl Pts',(-34.1896798357612,-1.38149478299821,
0.598688827541391));
#61706=CARTESIAN_POINT('Ctrl Pts',(-34.1101362085442,-1.25054175940707,
-0.83853864419688));
#61707=CARTESIAN_POINT('Ctrl Pts',(-34.0305925813271,0.0292850707204112,
-1.50534226452188));
#61708=CARTESIAN_POINT('Ctrl Pts',(-33.95104895411,1.28219436924234,-0.789258183429619));
#61709=CARTESIAN_POINT('Ctrl Pts',(-33.871505326893,1.35718503035677,0.651922322116352));
#61710=CARTESIAN_POINT('Ctrl Pts',(-33.7919616996759,0.185353446897111,
1.49418397750811));
#61711=CARTESIAN_POINT('Ctrl Pts',(-33.7124180724589,-1.1567565536606,0.963774909575826));
#61712=CARTESIAN_POINT('Ctrl Pts',(-33.6328744452418,-1.43617882914026,
-0.452037693320334));
#61713=CARTESIAN_POINT('Ctrl Pts',(-33.5533308180247,-0.396212159812758,
-1.45257081728134));
#61714=CARTESIAN_POINT('Ctrl Pts',(-33.4737871908077,1.00774629157814,-1.11865742453962));
#61715=CARTESIAN_POINT('Ctrl Pts',(-33.3942435635906,1.48590880876346,0.242944316826441));
#61716=CARTESIAN_POINT('Ctrl Pts',(-33.3146999363735,0.598996939754183,
1.38135780288018));
#61717=CARTESIAN_POINT('Ctrl Pts',(-33.2351563091566,-0.838201232648247,
1.25074599961759));
#61718=CARTESIAN_POINT('Ctrl Pts',(-33.1556126819394,-1.50536094578838,
-0.0289008665489891));
#61719=CARTESIAN_POINT('Ctrl Pts',(-33.0760690547224,-0.789576059365041,
-1.28199705793266));
#61720=CARTESIAN_POINT('Ctrl Pts',(-32.9965254275053,0.651576341838971,
-1.35734855625107));
#61721=CARTESIAN_POINT('Ctrl Pts',(-32.9169818002883,1.4941387685048,-0.185731439607652));
#61722=CARTESIAN_POINT('Ctrl Pts',(-32.8374381730712,0.964066192735147,
1.15651338081008));
#61723=CARTESIAN_POINT('Ctrl Pts',(-32.7578945458541,-0.45167445189681,
1.43629280328175));
#61724=CARTESIAN_POINT('Ctrl Pts',(-32.6783509186371,-1.45247093343298,
0.396579139408509));
#61725=CARTESIAN_POINT('Ctrl Pts',(-32.59880729142,-1.1189118095244,-1.00746374050411));
#61726=CARTESIAN_POINT('Ctrl Pts',(-32.519263664203,0.242568913490285,-1.48597010353709));
#61727=CARTESIAN_POINT('Ctrl Pts',(-32.4397200369859,1.38120649258727,-0.599345852627567));
#61728=CARTESIAN_POINT('Ctrl Pts',(-32.3601764097689,1.25095766374634,0.837885284336153));
#61729=CARTESIAN_POINT('Ctrl Pts',(-32.2806327825517,-0.0285206140419742,
1.50536819444095));
#61730=CARTESIAN_POINT('Ctrl Pts',(-32.2010891553348,-1.28179758182883,
0.789899857861043));
#61731=CARTESIAN_POINT('Ctrl Pts',(-32.1215455281176,-1.35751309302076,
-0.651233466973292));
#61732=CARTESIAN_POINT('Ctrl Pts',(-32.0420019009006,-0.18610884223578,
-1.49409180610823));
#61733=CARTESIAN_POINT('Ctrl Pts',(-31.9624582736835,1.15626982951559,-0.964358287974677));
#61734=CARTESIAN_POINT('Ctrl Pts',(-31.8829146464665,1.436406846299,0.451311641927037));
#61735=CARTESIAN_POINT('Ctrl Pts',(-31.8033710192494,0.396946009130357,
1.45237071440808));
#61736=CARTESIAN_POINT('Ctrl Pts',(-31.7238273920324,-1.00718108059297,
1.1191662508893));
#61737=CARTESIAN_POINT('Ctrl Pts',(-31.6442837648153,-1.4860313269786,-0.242193561996057));
#61738=CARTESIAN_POINT('Ctrl Pts',(-31.5647401375982,-0.599694714891924,
-1.38105505870149));
#61739=CARTESIAN_POINT('Ctrl Pts',(-31.4851965103812,0.837569276047795,
-1.25116926674808));
#61740=CARTESIAN_POINT('Ctrl Pts',(-31.4056528831641,1.50537535048078,0.0281403695611341));
#61741=CARTESIAN_POINT('Ctrl Pts',(-31.3261092559471,0.790223604150294,
1.28159801875546));
#61742=CARTESIAN_POINT('Ctrl Pts',(-31.24656562873,-0.650890549604056,1.35767754591078));
#61743=CARTESIAN_POINT('Ctrl Pts',(-31.1670220015129,-1.49404474888693,
0.18648623154965));
#61744=CARTESIAN_POINT('Ctrl Pts',(-31.0874783742959,-0.964650321421056,
-1.15602620368936));
#61745=CARTESIAN_POINT('Ctrl Pts',(-31.0079347470788,0.450948803023003,
-1.43652079806952));
#61746=CARTESIAN_POINT('Ctrl Pts',(-30.9283911198618,1.45227040279163,-0.397312853315405));
#61747=CARTESIAN_POINT('Ctrl Pts',(-30.8488474926447,1.1194206208098,1.0068983563101));
#61748=CARTESIAN_POINT('Ctrl Pts',(-30.7693038654276,-0.241818195028865,
1.48609245566592));
#61749=CARTESIAN_POINT('Ctrl Pts',(-30.6897602382106,-1.38090353671155,
0.600043538863403));
#61750=CARTESIAN_POINT('Ctrl Pts',(-30.6102166109935,-1.25138078991632,
-0.837253214304121));
#61751=CARTESIAN_POINT('Ctrl Pts',(-30.5306729837765,0.0277601232818883,
-1.50538241048232));
#61752=CARTESIAN_POINT('Ctrl Pts',(-30.4511293565594,1.28139837391439,-0.790547300016728));
#61753=CARTESIAN_POINT('Ctrl Pts',(-30.3715857293424,1.35784191217663,0.650547590703944));
#61754=CARTESIAN_POINT('Ctrl Pts',(-30.2920421021253,0.186863608965661,
1.49399759634295));
#61755=CARTESIAN_POINT('Ctrl Pts',(-30.2124984749082,-1.1557825041059,0.964942293319604));
#61756=CARTESIAN_POINT('Ctrl Pts',(-30.1329548476912,-1.43663465818619,
-0.450585935346916));
#61757=CARTESIAN_POINT('Ctrl Pts',(-30.0534112204741,-0.397679672150927,
-1.45216999851674));
#61758=CARTESIAN_POINT('Ctrl Pts',(-29.973867593257,1.00661556778455,-1.11967491930827));
#61759=CARTESIAN_POINT('Ctrl Pts',(-29.89432396604,1.48615348953668,0.241442812632994));
#61760=CARTESIAN_POINT('Ctrl Pts',(-29.8147803388229,0.600392324550558,
1.38075192661642));
#61761=CARTESIAN_POINT('Ctrl Pts',(-29.7352367116059,-0.836937099141528,
1.25159223324322));
#61762=CARTESIAN_POINT('Ctrl Pts',(-29.6556930843888,-1.50538937443656,
-0.0273798752314642));
#61763=CARTESIAN_POINT('Ctrl Pts',(-29.5761494571718,-0.790870945444198,
-1.28119864731679));
#61764=CARTESIAN_POINT('Ctrl Pts',(-29.4966058299547,0.65020459029722,-1.35800619180864));
#61765=CARTESIAN_POINT('Ctrl Pts',(-29.4170622027377,1.49395034847806,-0.187240974459272));
#61766=CARTESIAN_POINT('Ctrl Pts',(-29.3375185755206,0.965234203652314,
1.15553873078052));
#61767=CARTESIAN_POINT('Ctrl Pts',(-29.2579749483035,-0.45022303892228,
1.43674842664183));
#61768=CARTESIAN_POINT('Ctrl Pts',(-29.1784313210864,-1.45206950158965,
0.398046465613467));
#61769=CARTESIAN_POINT('Ctrl Pts',(-29.0988876938694,-1.11992914636859,
-1.0063327150343));
#61770=CARTESIAN_POINT('Ctrl Pts',(-29.0193440666523,0.241067414832435,
-1.486214428587));
#61771=CARTESIAN_POINT('Ctrl Pts',(-28.9398004394353,1.38060022842574,-0.600741071931139));
#61772=CARTESIAN_POINT('Ctrl Pts',(-28.8602568122182,1.2518035967153,0.836620930580172));
#61773=CARTESIAN_POINT('Ctrl Pts',(-28.7807131850012,-0.0269996254341221,
1.50539624234306));
#61774=CARTESIAN_POINT('Ctrl Pts',(-28.7011695577841,-1.2809988389754,0.791194540412063));
#61775=CARTESIAN_POINT('Ctrl Pts',(-28.621625930567,-1.35817038479635,-0.649861548405748));
#61776=CARTESIAN_POINT('Ctrl Pts',(-28.54208230335,-0.187618328006441,-1.49390300529527));
#61777=CARTESIAN_POINT('Ctrl Pts',(-28.4625386761329,1.15529488372878,-0.965526052400598));
#61778=CARTESIAN_POINT('Ctrl Pts',(-28.3829950489158,1.43686210342921,0.449860113772244));
#61779=CARTESIAN_POINT('Ctrl Pts',(-28.3034514216988,0.398413233679613,
1.45196891201676));
#61780=CARTESIAN_POINT('Ctrl Pts',(-28.2239077944817,-1.00604979807743,
1.12018330197452));
#61781=CARTESIAN_POINT('Ctrl Pts',(-28.1443641672647,-1.486275272813,-0.240692001651152));
#61782=CARTESIAN_POINT('Ctrl Pts',(-28.0648205400476,-0.601089780982883,
-1.38044844214919));
#61783=CARTESIAN_POINT('Ctrl Pts',(-27.9852769128306,0.836304708640234,
-1.25201488031906));
#61784=CARTESIAN_POINT('Ctrl Pts',(-27.9057332856135,1.50540301420138,0.0266193739141349));
#61785=CARTESIAN_POINT('Ctrl Pts',(-27.8261896583965,0.791518084899668,
1.28079894890297));
#61786=CARTESIAN_POINT('Ctrl Pts',(-27.7466460311794,-0.649518465051427,
1.35833449112927));
#61787=CARTESIAN_POINT('Ctrl Pts',(-27.6671024039623,-1.49385556679761,
0.18799566958307));
#61788=CARTESIAN_POINT('Ctrl Pts',(-27.5875587767453,-0.96581783954581,
-1.15505096296625));
#61789=CARTESIAN_POINT('Ctrl Pts',(-27.5080151495282,0.449497159919988,
-1.43697568854106));
#61790=CARTESIAN_POINT('Ctrl Pts',(-27.4284715223111,1.4518682298045,-0.398779976325944));
#61791=CARTESIAN_POINT('Ctrl Pts',(-27.3489278950941,1.12043738610985,1.00576681693199));
#61792=CARTESIAN_POINT('Ctrl Pts',(-27.269384267877,-0.240316573113117,
1.48633602221078));
#61793=CARTESIAN_POINT('Ctrl Pts',(-27.18984064066,-1.38029656779647,0.601438451683525));
#61794=CARTESIAN_POINT('Ctrl Pts',(-27.1102970134429,-1.25222608404103,
-0.835988433341909));
#61795=CARTESIAN_POINT('Ctrl Pts',(-27.0307533862258,0.0262391206957839,
-1.50540969001109));
#61796=CARTESIAN_POINT('Ctrl Pts',(-26.9512097590088,1.28059897711225,-0.791841578886351));
#61797=CARTESIAN_POINT('Ctrl Pts',(-26.8716661317917,1.35849851079693,0.649175340256163));
#61798=CARTESIAN_POINT('Ctrl Pts',(-26.7921225045747,0.188372999165078,
1.49380803298809));
#61799=CARTESIAN_POINT('Ctrl Pts',(-26.7125788773576,-1.15480696850846,
0.966109565069344));
#61800=CARTESIAN_POINT('Ctrl Pts',(-26.6330352501406,-1.43708918197015,
-0.449134177388628));
#61801=CARTESIAN_POINT('Ctrl Pts',(-26.5534916229235,-0.399146693529099,
-1.45176745495929));
#61802=CARTESIAN_POINT('Ctrl Pts',(-26.4739479957064,1.005483771616,-1.12069139875839));
#61803=CARTESIAN_POINT('Ctrl Pts',(-26.3944043684894,1.48639667677647,0.239941129242241));
#61804=CARTESIAN_POINT('Ctrl Pts',(-26.3148607412723,0.601787084010857,
1.38014460537724));
#61805=CARTESIAN_POINT('Ctrl Pts',(-26.2353171140552,-0.835672104705342,
1.25243720786774));
#61806=CARTESIAN_POINT('Ctrl Pts',(-26.1557734868382,-1.50541626977177,
-0.0258588658032874));
#61807=CARTESIAN_POINT('Ctrl Pts',(-26.0762298596211,-0.792165022351513,
-1.280398923616));
#61808=CARTESIAN_POINT('Ctrl Pts',(-25.9966862324041,0.648832174041817,
-1.35866244378887));
#61809=CARTESIAN_POINT('Ctrl Pts',(-25.917142605187,1.49376040386974,-0.188750316728418));
#61810=CARTESIAN_POINT('Ctrl Pts',(-25.83759897797,0.966401228952598,1.154562900371));
#61811=CARTESIAN_POINT('Ctrl Pts',(-25.7580553507529,-0.448771166201346,
1.43720258370922));
#61812=CARTESIAN_POINT('Ctrl Pts',(-25.6785117235359,-1.45166658748755,
0.399513385265661));
#61813=CARTESIAN_POINT('Ctrl Pts',(-25.5989680963187,-1.12094533990392,
-1.00520066214756));
#61814=CARTESIAN_POINT('Ctrl Pts',(-25.5194244691017,0.239565670062516,
-1.48645723650622));
#61815=CARTESIAN_POINT('Ctrl Pts',(-25.4398808418846,1.37999255490122,-0.602135677942593));
#61816=CARTESIAN_POINT('Ctrl Pts',(-25.3603372146676,1.2526482517857,0.835355722750746));
#61817=CARTESIAN_POINT('Ctrl Pts',(-25.2807935874506,-0.0254786092609561,
1.50542275348299));
#61818=CARTESIAN_POINT('Ctrl Pts',(-25.2012499602335,-1.280198788427,0.792488415274466));
#61819=CARTESIAN_POINT('Ctrl Pts',(-25.1217063330164,-1.35882629009462,
-0.648488966430325));
#61820=CARTESIAN_POINT('Ctrl Pts',(-25.0421627057993,-0.189127622248968,
-1.49371267944563));
#61821=CARTESIAN_POINT('Ctrl Pts',(-24.9626190785823,1.15431875856946,-0.966692831176921));
#61822=CARTESIAN_POINT('Ctrl Pts',(-24.8830754513652,1.43731589375105,0.448408126381329));
#61823=CARTESIAN_POINT('Ctrl Pts',(-24.8035318241482,0.399880051512201,
1.45156562739574));
#61824=CARTESIAN_POINT('Ctrl Pts',(-24.7239881969311,-1.00491748854471,
1.12119920953021));
#61825=CARTESIAN_POINT('Ctrl Pts',(-24.6444445697141,-1.48651770139613,
-0.239190195597884));
#61826=CARTESIAN_POINT('Ctrl Pts',(-24.564900942497,-0.602484233456529,
-1.3798404163781));
#61827=CARTESIAN_POINT('Ctrl Pts',(-24.48535731528,0.835039287498288,-1.25285921578146));
#61828=CARTESIAN_POINT('Ctrl Pts',(-24.4058136880629,1.50542914114434,0.025098351092998));
#61829=CARTESIAN_POINT('Ctrl Pts',(-24.3262700608458,0.792811757634631,
1.27999857155798));
#61830=CARTESIAN_POINT('Ctrl Pts',(-24.2467264336288,-0.648145717443526,
1.35899004970375));
#61831=CARTESIAN_POINT('Ctrl Pts',(-24.1671828064117,-1.49366485971877,
0.189504915702711));
#61832=CARTESIAN_POINT('Ctrl Pts',(-24.0876391791947,-0.966984371723771,
-1.15407454311936));
#61833=CARTESIAN_POINT('Ctrl Pts',(-24.0080955519776,0.44804505795169,-1.4374291120884));
#61834=CARTESIAN_POINT('Ctrl Pts',(-23.9285519247605,1.45146457469027,-0.400246692245398));
#61835=CARTESIAN_POINT('Ctrl Pts',(-23.8490082975435,1.1214530076211,1.00463425082552));
#61836=CARTESIAN_POINT('Ctrl Pts',(-23.7694646703264,-0.238814705872275,
1.48657807144237));
#61837=CARTESIAN_POINT('Ctrl Pts',(-23.6899210431094,-1.37968818981758,
0.602832750530412));
#61838=CARTESIAN_POINT('Ctrl Pts',(-23.6103774158923,-1.25307009984157,
-0.834722798968145));
#61839=CARTESIAN_POINT('Ctrl Pts',(-23.5308337886753,0.0247180913237032,
-1.50543543275542));
#61840=CARTESIAN_POINT('Ctrl Pts',(-23.4512901614581,1.27979827302174,-0.79313504941136));
#61841=CARTESIAN_POINT('Ctrl Pts',(-23.3717465342411,1.35915372260579,0.647802427103359));
#61842=CARTESIAN_POINT('Ctrl Pts',(-23.292202907024,0.18988219706556,1.49361694469223));
#61843=CARTESIAN_POINT('Ctrl Pts',(-23.212659279807,-1.15383025403633,0.967275850574507));
#61844=CARTESIAN_POINT('Ctrl Pts',(-23.1331156525899,-1.43754223871406,
-0.447681960935607));
#61845=CARTESIAN_POINT('Ctrl Pts',(-23.0535720253729,-0.400613307441811,
-1.4513634293776));
#61846=CARTESIAN_POINT('Ctrl Pts',(-22.9740283981558,1.00435094900806,-1.1217067341604));
#61847=CARTESIAN_POINT('Ctrl Pts',(-22.8944847709387,1.48663834664108,0.238439200909679));
#61848=CARTESIAN_POINT('Ctrl Pts',(-22.8149411437217,0.603181229142014,
1.37953587522939));
#61849=CARTESIAN_POINT('Ctrl Pts',(-22.7353975165046,-0.834406257180535,
1.25328090395256));
#61850=CARTESIAN_POINT('Ctrl Pts',(-22.6558538892876,-1.50544162831582,
-0.0243378299773199));
#61851=CARTESIAN_POINT('Ctrl Pts',(-22.5763102620705,-0.793458290584012,
-1.27959789283106));
#61852=CARTESIAN_POINT('Ctrl Pts',(-22.4967666348535,0.647459095431727,
-1.35931730879031));
#61853=CARTESIAN_POINT('Ctrl Pts',(-22.4172230076364,1.49356893436906,-0.190259466313405));
#61854=CARTESIAN_POINT('Ctrl Pts',(-22.3376793804193,0.967567267710527,
1.15358589133595));
#61855=CARTESIAN_POINT('Ctrl Pts',(-22.2581357532023,-0.447318835356281,
1.4376552736208));
#61856=CARTESIAN_POINT('Ctrl Pts',(-22.1785921259852,-1.4512621914642,0.400979897078039));
#61857=CARTESIAN_POINT('Ctrl Pts',(-22.0990484987682,-1.12196038913188,
-1.00406758311043));
#61858=CARTESIAN_POINT('Ctrl Pts',(-22.0195048715511,0.23806368073406,-1.48669852698842));
#61859=CARTESIAN_POINT('Ctrl Pts',(-21.939961244334,1.37938347262324,-0.603529669269067));
#61860=CARTESIAN_POINT('Ctrl Pts',(-21.860417617117,1.25349162810098,0.834089662155657));
#61861=CARTESIAN_POINT('Ctrl Pts',(-21.7808739898999,-0.0239575670781471,
1.50544772782514));
#61862=CARTESIAN_POINT('Ctrl Pts',(-21.7013303626828,-1.27939743099873,
0.793781481131954));
#61863=CARTESIAN_POINT('Ctrl Pts',(-21.6217867354658,-1.35948080824685,
-0.647115722450521));
#61864=CARTESIAN_POINT('Ctrl Pts',(-21.5422431082487,-0.190636723422224,
-1.49352082875232));
#61865=CARTESIAN_POINT('Ctrl Pts',(-21.4626994810317,1.1533414550338,-0.96785862311327));
#61866=CARTESIAN_POINT('Ctrl Pts',(-21.3831558538146,1.43776821680141,0.446955681236838));
#61867=CARTESIAN_POINT('Ctrl Pts',(-21.3036122265976,0.40134646113074,1.4511608609565));
#61868=CARTESIAN_POINT('Ctrl Pts',(-21.2240685993805,-1.00378415315067,
1.1222139725194));
#61869=CARTESIAN_POINT('Ctrl Pts',(-21.1445249721634,-1.48675861248054,
-0.237688145369336));
#61870=CARTESIAN_POINT('Ctrl Pts',(-21.0649813449464,-0.603878070889381,
-1.37923098200885));
#61871=CARTESIAN_POINT('Ctrl Pts',(-20.9854377177293,0.833773013913679,
-1.2537022722734));
#61872=CARTESIAN_POINT('Ctrl Pts',(-20.9058940905122,1.505453731283,0.0235773026504012));
#61873=CARTESIAN_POINT('Ctrl Pts',(-20.8263504632952,0.794104621034608,
1.27919688753752));
#61874=CARTESIAN_POINT('Ctrl Pts',(-20.7468068360781,-0.646772308181659,
1.35964422096501));
#61875=CARTESIAN_POINT('Ctrl Pts',(-20.6672632088611,-1.49347262784509,
0.191013968367933));
#61876=CARTESIAN_POINT('Ctrl Pts',(-20.587719581644,-0.96814991676412,-1.15309694514547));
#61877=CARTESIAN_POINT('Ctrl Pts',(-20.508175954427,0.446592498600472,-1.43788106824869));
#61878=CARTESIAN_POINT('Ctrl Pts',(-20.4286323272099,1.45105943786099,-0.40171299957647));
#61879=CARTESIAN_POINT('Ctrl Pts',(-20.3490886999928,1.12246748430675,1.00350065914689));
#61880=CARTESIAN_POINT('Ctrl Pts',(-20.2695450727758,-0.23731259483952,
1.48681860311361));
#61881=CARTESIAN_POINT('Ctrl Pts',(-20.1900014455587,-1.37907840339596,
0.604226433980696));
#61882=CARTESIAN_POINT('Ctrl Pts',(-20.1104578183417,-1.25391283645635,
-0.833456312474847));
#61883=CARTESIAN_POINT('Ctrl Pts',(-20.0309141911246,0.0231970367183806,
-1.50545963868902));
#61884=CARTESIAN_POINT('Ctrl Pts',(-19.9513705639075,1.27899626246024,-0.794427710271308));
#61885=CARTESIAN_POINT('Ctrl Pts',(-19.8718269366905,1.35980754693434,0.646428852647062));
#61886=CARTESIAN_POINT('Ctrl Pts',(-19.7922833094734,0.191391201126432,
1.49342433165044));
#61887=CARTESIAN_POINT('Ctrl Pts',(-19.7127396822564,-1.15285236168658,
0.968441148644485));
#61888=CARTESIAN_POINT('Ctrl Pts',(-19.6331960550393,-1.43799382795542,
-0.446229287470345));
#61889=CARTESIAN_POINT('Ctrl Pts',(-19.5536524278222,-0.402079512391888,
-1.45095792218413));
#61890=CARTESIAN_POINT('Ctrl Pts',(-19.4741088006052,1.00321710111716,-1.12272092447779));
#61891=CARTESIAN_POINT('Ctrl Pts',(-19.3945651733881,1.48687849888381,0.23693702916853));
#61892=CARTESIAN_POINT('Ctrl Pts',(-19.3150215461711,0.604574758520824,
1.37892573679429));
#61893=CARTESIAN_POINT('Ctrl Pts',(-19.235477918954,-0.83313955785933,1.25412332063643));
#61894=CARTESIAN_POINT('Ctrl Pts',(-19.1559342917369,-1.50546545004281,
-0.0228167693063023));
#61895=CARTESIAN_POINT('Ctrl Pts',(-19.0763906645199,-0.794750748821478,
-1.27879555577969));
#61896=CARTESIAN_POINT('Ctrl Pts',(-18.9968470373028,0.646085355868609,
-1.35997078614444));
#61897=CARTESIAN_POINT('Ctrl Pts',(-18.9173034100858,1.49337594017145,-0.191768421673692));
#61898=CARTESIAN_POINT('Ctrl Pts',(-18.8377597828687,0.96873231873582,1.15260770467272));
#61899=CARTESIAN_POINT('Ctrl Pts',(-18.7582161556517,-0.445866047869633,
1.43810649591444));
#61900=CARTESIAN_POINT('Ctrl Pts',(-18.6786725284346,-1.45085631393239,
0.402445999553601));
#61901=CARTESIAN_POINT('Ctrl Pts',(-18.5991289012175,-1.12297429301632,
-1.00293347907958));
#61902=CARTESIAN_POINT('Ctrl Pts',(-18.5195852740005,0.236561448380347,
-1.48693829978732));
#61903=CARTESIAN_POINT('Ctrl Pts',(-18.4400416467834,1.37877298221359,-0.604923044487492));
#61904=CARTESIAN_POINT('Ctrl Pts',(-18.3604980195663,1.25433372480018,0.832822750087366));
#61905=CARTESIAN_POINT('Ctrl Pts',(-18.2809543923493,-0.0224365004384819,
1.50547116534401));
#61906=CARTESIAN_POINT('Ctrl Pts',(-18.2014107651322,-1.27859476750868,
0.795073736664478));
#61907=CARTESIAN_POINT('Ctrl Pts',(-18.1218671379152,-1.36013393858487,
-0.645741817868261));
#61908=CARTESIAN_POINT('Ctrl Pts',(-18.0423235106981,-0.192145629985613,
-1.49332745341121));
#61909=CARTESIAN_POINT('Ctrl Pts',(-17.9627798834811,1.15236297411951,-0.969023427019504));
#61910=CARTESIAN_POINT('Ctrl Pts',(-17.883236256264,1.43821907211853,0.445502779821528));
#61911=CARTESIAN_POINT('Ctrl Pts',(-17.8036926290469,0.402812461038192,
1.45075461311227));
#61912=CARTESIAN_POINT('Ctrl Pts',(-17.7241490018299,-1.00264979305227,
1.12322758990617));
#61913=CARTESIAN_POINT('Ctrl Pts',(-17.6446053746128,-1.4869980058203,-0.236185852498931));
#61914=CARTESIAN_POINT('Ctrl Pts',(-17.5650617473958,-0.60527129185852,
-1.37862013966361));
#61915=CARTESIAN_POINT('Ctrl Pts',(-17.4855181201787,0.832505889179132,
-1.25454404893421));
#61916=CARTESIAN_POINT('Ctrl Pts',(-17.4059744929616,1.50547678459225,0.0220562301391384));
#61917=CARTESIAN_POINT('Ctrl Pts',(-17.3264308657446,0.795396673779736,
1.27839389766));
#61918=CARTESIAN_POINT('Ctrl Pts',(-17.2468872385275,-0.645398238667895,
1.36029700424524));
#61919=CARTESIAN_POINT('Ctrl Pts',(-17.1673436113104,-1.49327887137281,
0.192522826038173));
#61920=CARTESIAN_POINT('Ctrl Pts',(-17.0877999840934,-0.969314473476995,
-1.15211817004255));
#61921=CARTESIAN_POINT('Ctrl Pts',(-17.0082563568763,0.445139483349166,
-1.43833155656052));
#61922=CARTESIAN_POINT('Ctrl Pts',(-16.9287127296593,1.45065281973025,-0.403178896822321));
#61923=CARTESIAN_POINT('Ctrl Pts',(-16.8491691024422,1.12348081513121,1.00236604305328));
#61924=CARTESIAN_POINT('Ctrl Pts',(-16.7696254752252,-0.235810241548242,
1.48705761697896));
#61925=CARTESIAN_POINT('Ctrl Pts',(-16.6900818480081,-1.37846720915408,
0.605619500611681));
#61926=CARTESIAN_POINT('Ctrl Pts',(-16.610538220791,-1.25475429302508,-0.832188975154876));
#61927=CARTESIAN_POINT('Ctrl Pts',(-16.530994593574,0.0216759584325402,
-1.50548230778718));
#61928=CARTESIAN_POINT('Ctrl Pts',(-16.4514509663569,1.27819294624648,-0.79571956014662));
#61929=CARTESIAN_POINT('Ctrl Pts',(-16.3719073391399,1.36045998311514,0.645054618289458));
#61930=CARTESIAN_POINT('Ctrl Pts',(-16.2923637119228,0.192900009807252,
1.49323019405936));
#61931=CARTESIAN_POINT('Ctrl Pts',(-16.2128200847058,-1.15187329245748,
0.969605458089701));
#61932=CARTESIAN_POINT('Ctrl Pts',(-16.1332764574887,-1.43844394923324,
-0.444776158475778));
#61933=CARTESIAN_POINT('Ctrl Pts',(-16.0537328302716,-0.403545306882577,
-1.45055093379282));
#61934=CARTESIAN_POINT('Ctrl Pts',(-15.9741892030546,1.00208222910077,-1.12373396867525));
#61935=CARTESIAN_POINT('Ctrl Pts',(-15.8946455758375,1.4871171332595,0.235434615552267));
#61936=CARTESIAN_POINT('Ctrl Pts',(-15.8151019486204,0.605967670724726,
1.37831419069479));
#61937=CARTESIAN_POINT('Ctrl Pts',(-15.7355583214034,-0.831872008034821,
1.25496445705936));
#61938=CARTESIAN_POINT('Ctrl Pts',(-15.6560146941863,-1.50548773492844,
-0.0212956853429847));
#61939=CARTESIAN_POINT('Ctrl Pts',(-15.5764710669693,-0.796042395744522,
-1.27799191328095));
#61940=CARTESIAN_POINT('Ctrl Pts',(-15.4969274397522,0.644710956754863,
-1.36062287518416));
#61941=CARTESIAN_POINT('Ctrl Pts',(-15.4173838125351,1.49318142147395,-0.193277181268826));
#61942=CARTESIAN_POINT('Ctrl Pts',(-15.3378401853181,0.969896380839092,
1.1516283413799));
#61943=CARTESIAN_POINT('Ctrl Pts',(-15.2582965581011,-0.444412805224505,
1.43855625012951));
#61944=CARTESIAN_POINT('Ctrl Pts',(-15.178752930884,-1.45044895530648,0.403911691195623));
#61945=CARTESIAN_POINT('Ctrl Pts',(-15.0992093036669,-1.12398705052216,
-1.0017983512128));
#61946=CARTESIAN_POINT('Ctrl Pts',(-15.0196656764499,0.235058974534927,
-1.48717655465811));
#61947=CARTESIAN_POINT('Ctrl Pts',(-14.9401220492328,1.37816108429549,-0.606315802175471));
#61948=CARTESIAN_POINT('Ctrl Pts',(-14.8605784220157,1.25517454102367,0.831554987839188));
#61949=CARTESIAN_POINT('Ctrl Pts',(-14.7810347947987,-0.0209154108947242,
1.50549306601567));
#61950=CARTESIAN_POINT('Ctrl Pts',(-14.7014911675816,-1.27779079877622,
0.796365180552865));
#61951=CARTESIAN_POINT('Ctrl Pts',(-14.6219475403646,-1.36078568044193,
-0.644367254086051));
#61952=CARTESIAN_POINT('Ctrl Pts',(-14.5424039131475,-0.193654340398797,
-1.49313255361971));
#61953=CARTESIAN_POINT('Ctrl Pts',(-14.4628602859304,1.15138331682546,-0.970187241706543));
#61954=CARTESIAN_POINT('Ctrl Pts',(-14.3833166587134,1.43866845924216,0.444049423618571));
#61955=CARTESIAN_POINT('Ctrl Pts',(-14.3037730314963,0.404278049738003,
1.45034688427777));
#61956=CARTESIAN_POINT('Ctrl Pts',(-14.2242294042793,-1.00151440940753,
1.12424006065575));
#61957=CARTESIAN_POINT('Ctrl Pts',(-14.1446857770622,-1.48723588117101,
-0.234683318520279));
#61958=CARTESIAN_POINT('Ctrl Pts',(-14.0651421498451,-0.606663894941661,
-1.37800788996596));
#61959=CARTESIAN_POINT('Ctrl Pts',(-13.9855985226281,0.8312379145882,-1.25538454490456));
#61960=CARTESIAN_POINT('Ctrl Pts',(-13.906054895411,1.50549830104856,0.0205351351119899));
#61961=CARTESIAN_POINT('Ctrl Pts',(-13.8265112681939,0.796687914551029,
1.27758960274516));
#61962=CARTESIAN_POINT('Ctrl Pts',(-13.7469676409769,-0.644023510304975,
1.36094839887803));
#61963=CARTESIAN_POINT('Ctrl Pts',(-13.6674240137598,-1.49308359049973,
0.194031487173097));
#61964=CARTESIAN_POINT('Ctrl Pts',(-13.5878803865428,-0.970478040673556,
-1.15113821880979));
#61965=CARTESIAN_POINT('Ctrl Pts',(-13.5083367593257,0.443686013681124,
-1.43878057656404));
#61966=CARTESIAN_POINT('Ctrl Pts',(-13.4287931321087,1.45024472071316,-0.404644382486428));
#61967=CARTESIAN_POINT('Ctrl Pts',(-13.3492495048916,1.12449299905994,1.00123040370303));
#61968=CARTESIAN_POINT('Ctrl Pts',(-13.2697058776745,-0.234307647532164,
1.4872951127944));
#61969=CARTESIAN_POINT('Ctrl Pts',(-13.1901622504575,-1.37785460771592,
0.607011949001187));
#61970=CARTESIAN_POINT('Ctrl Pts',(-13.1106186232404,-1.25559446868872,
-0.830920788302052));
#61971=CARTESIAN_POINT('Ctrl Pts',(-13.0310749960233,0.020154858019065,
-1.50550344002676));
#61972=CARTESIAN_POINT('Ctrl Pts',(-12.9515313688063,1.27738832520053,-0.797010597718466));
#61973=CARTESIAN_POINT('Ctrl Pts',(-12.8719877415892,1.36111103048212,0.643679725433465));
#61974=CARTESIAN_POINT('Ctrl Pts',(-12.7924441143722,0.194408621567738,
1.49303453211717));
#61975=CARTESIAN_POINT('Ctrl Pts',(-12.7129004871551,-1.15089304734852,
0.970768777721553));
#61976=CARTESIAN_POINT('Ctrl Pts',(-12.6333568599381,-1.43889260208799,
-0.443322575435331));
#61977=CARTESIAN_POINT('Ctrl Pts',(-12.553813232721,-0.405010689417524,
-1.45014246461917));
#61978=CARTESIAN_POINT('Ctrl Pts',(-12.474269605504,1.00094633411743,-1.1247458657186));
#61979=CARTESIAN_POINT('Ctrl Pts',(-12.3947259782869,1.48735424952452,0.233931961594643));
#61980=CARTESIAN_POINT('Ctrl Pts',(-12.3151823510698,0.607359964331746,
1.37770123755521));
#61981=CARTESIAN_POINT('Ctrl Pts',(-12.2356387238528,-0.830603609001021,
1.25580431236267));
#61982=CARTESIAN_POINT('Ctrl Pts',(-12.1560950966357,-1.50550848294994,
-0.0197745796402064));
#61983=CARTESIAN_POINT('Ctrl Pts',(-12.0765514694186,-0.797333230034552,
-1.27718696615524));
#61984=CARTESIAN_POINT('Ctrl Pts',(-11.9970078422016,0.643335899493558,
-1.36127357524379));
#61985=CARTESIAN_POINT('Ctrl Pts',(-11.9174642149845,1.49298537847513,-0.19478574355858));
#61986=CARTESIAN_POINT('Ctrl Pts',(-11.8379205877675,0.971059452831992,
1.15064780245729));
#61987=CARTESIAN_POINT('Ctrl Pts',(-11.7583769605504,-0.442959108904438,
1.43900453580687));
#61988=CARTESIAN_POINT('Ctrl Pts',(-11.6788333333333,-1.45004011600234,
0.405376970507859));
#61989=CARTESIAN_POINT('Ctrl Pts',(-11.5992897061163,-1.12499866061553,
-1.00066220066888));
#61990=CARTESIAN_POINT('Ctrl Pts',(-11.5197460788992,0.233556260731656,
-1.48741329135758));
#61991=CARTESIAN_POINT('Ctrl Pts',(-11.4402024516822,1.37754777949356,-0.607707940911187));
#61992=CARTESIAN_POINT('Ctrl Pts',(-11.3606588244651,1.25601407591308,0.830286376705301));
#61993=CARTESIAN_POINT('Ctrl Pts',(-11.281115197248,-0.0193942999996536,
1.50551342981779));
#61994=CARTESIAN_POINT('Ctrl Pts',(-11.201571570031,-1.27698552562212,0.797655811478712));
#61995=CARTESIAN_POINT('Ctrl Pts',(-11.1220279428139,-1.36143603315269,
-0.642992032507123));
#61996=CARTESIAN_POINT('Ctrl Pts',(-11.0424843155969,-0.195162853121622,
-1.49293612957676));
#61997=CARTESIAN_POINT('Ctrl Pts',(-10.9629406883798,1.15040248415175,-0.971350065986352));
#61998=CARTESIAN_POINT('Ctrl Pts',(-10.8833970611627,1.43911637771354,0.442595614111609));
#61999=CARTESIAN_POINT('Ctrl Pts',(-10.8038534339457,0.405743225734111,
1.44993767486918));
#62000=CARTESIAN_POINT('Ctrl Pts',(-10.7243098067286,-1.00037800337546,
1.12525138373465));
#62001=CARTESIAN_POINT('Ctrl Pts',(-10.6447661795116,-1.48747223828985,
-0.23318054496715));
#62002=CARTESIAN_POINT('Ctrl Pts',(-10.5652225522945,-0.608055878717266,
-1.37739423354083));
#62003=CARTESIAN_POINT('Ctrl Pts',(-10.4856789250774,0.829969091435158,
-1.25622375932652));
#62004=CARTESIAN_POINT('Ctrl Pts',(-10.4061352978604,1.50551828062998,0.0190140191216825));
#62005=CARTESIAN_POINT('Ctrl Pts',(-10.3265916706433,0.797978342030396,
1.27678400361401));
#62006=CARTESIAN_POINT('Ctrl Pts',(-10.2470480434263,-0.642648124496163,
1.36159840419844));
#62007=CARTESIAN_POINT('Ctrl Pts',(-10.1675044162092,-1.4928867854252,0.195539950232733));
#62008=CARTESIAN_POINT('Ctrl Pts',(-10.0879607889921,-0.971640617166035,
-1.15015709244756));
#62009=CARTESIAN_POINT('Ctrl Pts',(-10.0084171617751,0.442232091080033,
-1.43922812780085));
#62010=CARTESIAN_POINT('Ctrl Pts',(-9.92887353455803,1.44983514122626,-0.406109455072875));
#62011=CARTESIAN_POINT('Ctrl Pts',(-9.84932990734096,1.1255040350598,1.00009374225535));
#62012=CARTESIAN_POINT('Ctrl Pts',(-9.76978628012392,-0.232804814325147,
1.48753109031752));
#62013=CARTESIAN_POINT('Ctrl Pts',(-9.69024265290684,-1.37724059970678,
0.608403777727809));
#62014=CARTESIAN_POINT('Ctrl Pts',(-9.61069902568979,-1.25643336258963,
-0.829651753210869));
#62015=CARTESIAN_POINT('Ctrl Pts',(-9.53115539847272,0.0186337370306052,
-1.5055230353862));
#62016=CARTESIAN_POINT('Ctrl Pts',(-9.45161177125567,1.27658240014378,-0.798300821668966));
#62017=CARTESIAN_POINT('Ctrl Pts',(-9.37206814403861,1.36176068837068,0.642304175482586));
#62018=CARTESIAN_POINT('Ctrl Pts',(-9.29252451682155,0.195917034867912,
1.49283734602358));
#62019=CARTESIAN_POINT('Ctrl Pts',(-9.21298088960449,-1.14991162736034,
0.971931106352556));
#62020=CARTESIAN_POINT('Ctrl Pts',(-9.13343726238743,-1.43933978606171,
-0.441868539832883));
#62021=CARTESIAN_POINT('Ctrl Pts',(-9.05389363517037,-0.406475658500802,
-1.44973251508011));
#62022=CARTESIAN_POINT('Ctrl Pts',(-8.97435000795331,0.999809417326651,
-1.12575661457488));
#62023=CARTESIAN_POINT('Ctrl Pts',(-8.89480638073625,1.48758984743686,0.232429068829558));
#62024=CARTESIAN_POINT('Ctrl Pts',(-8.81526275351918,0.608751637920644,
1.37708687800122));
#62025=CARTESIAN_POINT('Ctrl Pts',(-8.73571912630213,-0.829334362052652,
1.25664288568904));
#62026=CARTESIAN_POINT('Ctrl Pts',(-8.65617549908508,-1.50552769408614,
-0.0182534537506204));
#62027=CARTESIAN_POINT('Ctrl Pts',(-8.576631871868,-0.798623250373908,-1.27638071522427));
#62028=CARTESIAN_POINT('Ctrl Pts',(-8.49708824465096,0.641960185488325,
-1.3619228856591));
#62029=CARTESIAN_POINT('Ctrl Pts',(-8.41754461743388,1.49278781137509,-0.196294107003054));
#62030=CARTESIAN_POINT('Ctrl Pts',(-8.33800099021684,0.97222153352733,1.14966608890581));
#62031=CARTESIAN_POINT('Ctrl Pts',(-8.25845736299977,-0.441504960393397,
1.43945135248894));
#62032=CARTESIAN_POINT('Ctrl Pts',(-8.17891373578272,-1.44962979643727,
0.406841835994534));
#62033=CARTESIAN_POINT('Ctrl Pts',(-8.09937010856564,-1.12600912226377,
-0.999525028607551));
#62034=CARTESIAN_POINT('Ctrl Pts',(-8.0198264813486,0.232053308504426,-1.48764850964411));
#62035=CARTESIAN_POINT('Ctrl Pts',(-7.94028285413152,1.37693306843394,-0.609099459273521));
#62036=CARTESIAN_POINT('Ctrl Pts',(-7.86073922691448,1.25685232861138,0.829016917980754));
#62037=CARTESIAN_POINT('Ctrl Pts',(-7.78119559969741,-0.0178731693060422,
1.50553225672953));
#62038=CARTESIAN_POINT('Ctrl Pts',(-7.70165197248036,-1.27617894886838,
0.798945628124588));
#62039=CARTESIAN_POINT('Ctrl Pts',(-7.6221083452633,-1.36208499605328,-0.641616154535358));
#62040=CARTESIAN_POINT('Ctrl Pts',(-7.54256471804624,-0.196671166614124,
-1.49273818148288));
#62041=CARTESIAN_POINT('Ctrl Pts',(-7.46302109082917,1.14942047709957,-0.972511898671863));
#62042=CARTESIAN_POINT('Ctrl Pts',(-7.38347746361211,1.43956282707545,0.441141352784717));
#62043=CARTESIAN_POINT('Ctrl Pts',(-7.30393383639506,0.407207987530731,
1.4495269853043));
#62044=CARTESIAN_POINT('Ctrl Pts',(-7.22439020917799,-0.999240576116165,
1.12626155811037));
#62045=CARTESIAN_POINT('Ctrl Pts',(-7.14484658196094,-1.48770707693553,
-0.231677533373667));
#62046=CARTESIAN_POINT('Ctrl Pts',(-7.06530295474388,-0.609447241764305,
-1.37677917101476));
#62047=CARTESIAN_POINT('Ctrl Pts',(-6.98575932752682,0.828699421015416,
-1.25706169134332));
#62048=CARTESIAN_POINT('Ctrl Pts',(-6.90621570030976,1.50553672331607,0.0174928837211134));
#62049=CARTESIAN_POINT('Ctrl Pts',(-6.8266720730927,0.799267954900482,1.27597710108895));
#62050=CARTESIAN_POINT('Ctrl Pts',(-6.74712844587562,-0.641272082645586,
1.36224701954293));
#62051=CARTESIAN_POINT('Ctrl Pts',(-6.6675848186586,-1.49268845635011,0.197048213677092));
#62052=CARTESIAN_POINT('Ctrl Pts',(-6.5880411914415,-0.972802201767608,
-1.14917479195737));
#62053=CARTESIAN_POINT('Ctrl Pts',(-6.50849756422447,0.440777717030083,
-1.43967420981412));
#62054=CARTESIAN_POINT('Ctrl Pts',(-6.42895393700739,1.44942408168774,-0.407574113086008));
#62055=CARTESIAN_POINT('Ctrl Pts',(-6.34941030979035,1.12651392209859,0.998956059870634));
#62056=CARTESIAN_POINT('Ctrl Pts',(-6.26986668257328,-0.231301743461309,
1.48776554930739));
#62057=CARTESIAN_POINT('Ctrl Pts',(-6.19032305535623,-1.37662518575351,
0.609794985370748));
#62058=CARTESIAN_POINT('Ctrl Pts',(-6.11077942813915,-1.25727097387143,
-0.828381871176925));
#62059=CARTESIAN_POINT('Ctrl Pts',(-6.0312358009221,0.0171125970200911,
-1.50554109384546));
#62060=CARTESIAN_POINT('Ctrl Pts',(-5.95169217370504,1.2757751718989,-0.799590230680999));
#62061=CARTESIAN_POINT('Ctrl Pts',(-5.87214854648798,1.36240895611768,0.64092796984103));
#62062=CARTESIAN_POINT('Ctrl Pts',(-5.79260491927093,0.197425248167845,
1.49263863597994));
#62063=CARTESIAN_POINT('Ctrl Pts',(-5.71306129205386,-1.14892903349483,
0.973092442796056));
#62064=CARTESIAN_POINT('Ctrl Pts',(-5.63351766483681,-1.43978550069785,
-0.440414053152718));
#62065=CARTESIAN_POINT('Ctrl Pts',(-5.55397403761974,-0.407940212636969,
-1.44932108559419));
#62066=CARTESIAN_POINT('Ctrl Pts',(-5.47443041040269,0.998671479889131,
-1.12676621421227));
#62067=CARTESIAN_POINT('Ctrl Pts',(-5.39488678318562,1.48782392675596,0.230925938791301));
#62068=CARTESIAN_POINT('Ctrl Pts',(-5.31534315596856,0.610142690070709,
1.37647111265999));
#62069=CARTESIAN_POINT('Ctrl Pts',(-5.23579952875151,-0.828064268485496,
1.25748017618243));
#62070=CARTESIAN_POINT('Ctrl Pts',(-5.15625590153445,-1.50554536831745,
-0.0167323092272154));
#62071=CARTESIAN_POINT('Ctrl Pts',(-5.07671227431738,-0.799912455445589,
-1.27557316131109));
#62072=CARTESIAN_POINT('Ctrl Pts',(-4.99716864710033,0.64058381614358,-1.36257080576721));
#62073=CARTESIAN_POINT('Ctrl Pts',(-4.91762501988326,1.49258872037557,-0.197802270062393));
#62074=CARTESIAN_POINT('Ctrl Pts',(-4.83808139266621,0.973382621738716,
1.14868320172765));
#62075=CARTESIAN_POINT('Ctrl Pts',(-4.75853776544914,-0.440050361175798,
1.43989669971953));
#62076=CARTESIAN_POINT('Ctrl Pts',(-4.67899413823209,-1.44921799703017,
0.408306286160309));
#62077=CARTESIAN_POINT('Ctrl Pts',(-4.59945051101503,-1.12701843443538,
-0.998386836189773));
#62078=CARTESIAN_POINT('Ctrl Pts',(-4.51990688379797,0.230550119387597,
-1.48788220927752));
#62079=CARTESIAN_POINT('Ctrl Pts',(-4.44036325658091,1.37631695174408,-0.610490355841967));
#62080=CARTESIAN_POINT('Ctrl Pts',(-4.36081962936385,1.25768929826291,0.827746612961421));
#62081=CARTESIAN_POINT('Ctrl Pts',(-4.28127600214679,-0.0163520203667641,
1.50554954673173));
#62082=CARTESIAN_POINT('Ctrl Pts',(-4.20173237492973,-1.27537106933841,
0.800234629173721));
#62083=CARTESIAN_POINT('Ctrl Pts',(-4.12218874771268,-1.36273256848119,
-0.640239621575252));
#62084=CARTESIAN_POINT('Ctrl Pts',(-4.04264512049561,-0.198179279336608,
-1.49253870954017));
#62085=CARTESIAN_POINT('Ctrl Pts',(-3.96310149327855,1.1484372966715,-0.973672738577014));
#62086=CARTESIAN_POINT('Ctrl Pts',(-3.88355786606149,1.44000780687209,0.439686641122523));
#62087=CARTESIAN_POINT('Ctrl Pts',(-3.80401423884443,0.408672333632629,
1.44911481600231));
#62088=CARTESIAN_POINT('Ctrl Pts',(-3.72447061162738,-0.998102128790777,
1.12727058275177));
#62089=CARTESIAN_POINT('Ctrl Pts',(-3.64492698441031,-1.48794039686834,
-0.230174285274219));
#62090=CARTESIAN_POINT('Ctrl Pts',(-3.56538335719326,-0.610837982662363,
-1.37616270301558));
#62091=CARTESIAN_POINT('Ctrl Pts',(-3.48583972997619,0.827428904625004,
-1.25789834009956));
#62092=CARTESIAN_POINT('Ctrl Pts',(-3.40629610275914,1.50555362908805,0.0159717304630367));
#62093=CARTESIAN_POINT('Ctrl Pts',(-3.32675247554207,0.800556751844799,
1.27516889599378));
#62094=CARTESIAN_POINT('Ctrl Pts',(-3.24720884832502,-0.639895386158011,
1.36289424424926));
#62095=CARTESIAN_POINT('Ctrl Pts',(-3.16766522110796,-1.49248860347686,
0.198556275966578));
#62096=CARTESIAN_POINT('Ctrl Pts',(-3.08812159389089,-0.973962793292614,
-1.14819131834222));
#62097=CARTESIAN_POINT('Ctrl Pts',(-3.00857796667384,0.439322893016301,
-1.44011882214814));
#62098=CARTESIAN_POINT('Ctrl Pts',(-2.92903433945677,1.44901154251677,-0.409038355031158));
#62099=CARTESIAN_POINT('Ctrl Pts',(-2.84949071223972,1.12752265914617,0.997817357711321));
#62100=CARTESIAN_POINT('Ctrl Pts',(-2.76994708502266,-0.229798436476582,
1.48799848952268));
#62101=CARTESIAN_POINT('Ctrl Pts',(-2.6904034578056,-1.37600836648151,0.611185570513587));
#62102=CARTESIAN_POINT('Ctrl Pts',(-2.61085983058853,-1.2581073016844,-0.827111143503776));
#62103=CARTESIAN_POINT('Ctrl Pts',(-2.53131620337148,0.0155914395504356,
-1.50555761537229));
#62104=CARTESIAN_POINT('Ctrl Pts',(-2.45177257615442,1.27496664127071,-0.800878823464588));
#62105=CARTESIAN_POINT('Ctrl Pts',(-2.37222894893736,1.3630558330979,0.639551109963632));
#62106=CARTESIAN_POINT('Ctrl Pts',(-2.2926853217203,0.198933259858434,1.49243840209429));
#62107=CARTESIAN_POINT('Ctrl Pts',(-2.21314169450324,-1.14794526662311,
0.974252786046452));
#62108=CARTESIAN_POINT('Ctrl Pts',(-2.13359806728618,-1.44022974579189,
-0.438959117221064));
#62109=CARTESIAN_POINT('Ctrl Pts',(-2.05405444006912,-0.409404349855524,
-1.4489081759335));
#62110=CARTESIAN_POINT('Ctrl Pts',(-1.97451081285206,0.997532522064249,
-1.12777466482976));
#62111=CARTESIAN_POINT('Ctrl Pts',(-1.894967185635,1.48805648895523,0.229422575348086));
#62112=CARTESIAN_POINT('Ctrl Pts',(-1.81542355841794,0.611533116111903,
1.37585393773064));
#62113=CARTESIAN_POINT('Ctrl Pts',(-1.73587993120088,-0.826793323427721,
1.25831619139526));
#62114=CARTESIAN_POINT('Ctrl Pts',(-1.65633630398382,-1.50556151733331,
-0.0152111635795861));
#62115=CARTESIAN_POINT('Ctrl Pts',(-1.57679267676677,-0.801200821712858,
-1.2747642749542));
#62116=CARTESIAN_POINT('Ctrl Pts',(-1.4972490495497,0.639206750689721,-1.36321739238898));
#62117=CARTESIAN_POINT('Ctrl Pts',(-1.41770542233265,1.49238818572684,-0.199310122096324));
#62118=CARTESIAN_POINT('Ctrl Pts',(-1.33816179511559,0.97454256435248,1.1476989348545));
#62119=CARTESIAN_POINT('Ctrl Pts',(-1.25861816789852,-0.438595024378369,
1.44034097006356));
#62120=CARTESIAN_POINT('Ctrl Pts',(-1.17907454068146,-1.44880526550185,
0.409769573563957));
#62121=CARTESIAN_POINT('Ctrl Pts',(-1.0995309134644,-1.12802555733051,-0.997246208780835));
#62122=CARTESIAN_POINT('Ctrl Pts',(-1.01998728624735,0.22904472334399,-1.48811707718389));
#62123=CARTESIAN_POINT('Ctrl Pts',(-0.940443659030285,1.37570317207231,
-0.611875528990654));
#62124=CARTESIAN_POINT('Ctrl Pts',(-0.860900031813226,1.25851788170227,
0.826465782811734));
#62125=CARTESIAN_POINT('Ctrl Pts',(-0.781356404596167,-0.0148173746002297,
1.50558367261418));
#62126=CARTESIAN_POINT('Ctrl Pts',(-0.701812777379109,-1.27458747328757,
0.801487941651361));
#62127=CARTESIAN_POINT('Ctrl Pts',(-0.622269150162049,-1.36333018639518,
-0.638796246547649));
#62128=CARTESIAN_POINT('Ctrl Pts',(-0.542725522944984,-0.199779384003955,
-1.49246336007472));
#62129=CARTESIAN_POINT('Ctrl Pts',(-0.463181895727926,1.14762810985679,
-0.974593930371403));
#62130=CARTESIAN_POINT('Ctrl Pts',(-0.383638268510868,1.44011730997828,
0.437777000149017));
#62131=CARTESIAN_POINT('Ctrl Pts',(-0.304094641293808,0.41078325908372,
1.44957660963075));
#62132=CARTESIAN_POINT('Ctrl Pts',(-0.224551014076749,-0.998300100086838,
1.12650835861515));
#62133=CARTESIAN_POINT('Ctrl Pts',(-0.171521929265376,-1.32265134589549,
0.225893933992271));
#62134=CARTESIAN_POINT('Ctrl Pts',(-0.145007386859689,-1.2582325722701,
-0.193338547834049));
#62135=CARTESIAN_POINT('Ctrl Pts',(-34.6914926131403,-0.592743564845966,
1.23319225136785));
#62136=CARTESIAN_POINT('Ctrl Pts',(-34.6649780707346,-1.00363282292421,
1.03569509444031));
#62137=CARTESIAN_POINT('Ctrl Pts',(-34.6119489859233,-1.60527835398769,
0.20107823259307));
#62138=CARTESIAN_POINT('Ctrl Pts',(-34.5324053587062,-1.03595602557903,
-1.24467622864298));
#62139=CARTESIAN_POINT('Ctrl Pts',(-34.4528617314891,0.486450185413046,
-1.54294323461826));
#62140=CARTESIAN_POINT('Ctrl Pts',(-34.3733181042721,1.56125942409536,-0.425764039114321));
#62141=CARTESIAN_POINT('Ctrl Pts',(-34.293774477055,1.20214066618724,1.08361093293141));
#62142=CARTESIAN_POINT('Ctrl Pts',(-34.214230849838,-0.261554730735344,
1.59694004015695));
#62143=CARTESIAN_POINT('Ctrl Pts',(-34.1346872226209,-1.4848627155046,0.643484672649936));
#62144=CARTESIAN_POINT('Ctrl Pts',(-34.0551435954039,-1.34411136080804,
-0.901280832617842));
#62145=CARTESIAN_POINT('Ctrl Pts',(-33.9755999681868,0.0314762749515779,
-1.61797686836768));
#62146=CARTESIAN_POINT('Ctrl Pts',(-33.8960563409697,1.37813232185068,-0.848313047507812));
#62147=CARTESIAN_POINT('Ctrl Pts',(-33.8165127137527,1.45873402811122,0.70070127041307));
#62148=CARTESIAN_POINT('Ctrl Pts',(-33.7369690865356,0.199222194592942,
1.60598368203102));
#62149=CARTESIAN_POINT('Ctrl Pts',(-33.6574254593185,-1.24330884096325,
1.03588768266065));
#62150=CARTESIAN_POINT('Ctrl Pts',(-33.5778818321015,-1.54363839982021,
-0.485860623633696));
#62151=CARTESIAN_POINT('Ctrl Pts',(-33.4983382048844,-0.425858042155266,
-1.56125688982344));
#62152=CARTESIAN_POINT('Ctrl Pts',(-33.4187945776674,1.08314914646654,-1.2023590110968));
#62153=CARTESIAN_POINT('Ctrl Pts',(-33.3392509504503,1.59708933824868,0.261122200705366));
#62154=CARTESIAN_POINT('Ctrl Pts',(-33.2597073232333,0.643815838820516,
1.48471548608867));
#62155=CARTESIAN_POINT('Ctrl Pts',(-33.1801636960162,-0.900918174839821,
1.34433088293534));
#62156=CARTESIAN_POINT('Ctrl Pts',(-33.1006200687992,-1.61799694742729,
-0.0310633233745565));
#62157=CARTESIAN_POINT('Ctrl Pts',(-33.021076441582,-0.848654707954505,
-1.37792024706712));
#62158=CARTESIAN_POINT('Ctrl Pts',(-32.941532814365,0.700329402766152,-1.45890978954474));
#62159=CARTESIAN_POINT('Ctrl Pts',(-32.8619891871479,1.60593509034306,-0.19962846994738));
#62160=CARTESIAN_POINT('Ctrl Pts',(-32.7824455599309,1.03620076057325,1.24304747312922));
#62161=CARTESIAN_POINT('Ctrl Pts',(-32.7029019327138,-0.485470203305545,
1.54376090187762));
#62162=CARTESIAN_POINT('Ctrl Pts',(-32.6233583054968,-1.5611495323407,0.426252480357849));
#62163=CARTESIAN_POINT('Ctrl Pts',(-32.5438146782797,-1.20263242999344,
-1.08284545400225));
#62164=CARTESIAN_POINT('Ctrl Pts',(-32.4642710510626,0.260718708470727,
-1.59715521929662));
#62165=CARTESIAN_POINT('Ctrl Pts',(-32.3847274238456,1.48455285426756,-0.644190858489808));
#62166=CARTESIAN_POINT('Ctrl Pts',(-32.3051837966285,1.34455838446256,0.900578586247502));
#62167=CARTESIAN_POINT('Ctrl Pts',(-32.2256401694115,-0.0306546191383235,
1.61800473844763));
#62168=CARTESIAN_POINT('Ctrl Pts',(-32.1460965421944,-1.37770584551247,
0.849002734107022));
#62169=CARTESIAN_POINT('Ctrl Pts',(-32.0665529149774,-1.45908663749064,
-0.699960872887939));
#62170=CARTESIAN_POINT('Ctrl Pts',(-31.9870092877603,-0.200034111067518,
-1.60588461406724));
#62171=CARTESIAN_POINT('Ctrl Pts',(-31.9074656605433,1.2427856985348,-1.03651471132854));
#62172=CARTESIAN_POINT('Ctrl Pts',(-31.8279220333262,1.54388347796431,0.485080246713917));
#62173=CARTESIAN_POINT('Ctrl Pts',(-31.7483784061091,0.426646800465404,
1.56104181460244));
#62174=CARTESIAN_POINT('Ctrl Pts',(-31.6688347788921,-1.0825416445573,1.20290590948875));
#62175=CARTESIAN_POINT('Ctrl Pts',(-31.589291151675,-1.59722102367513,-0.260315271956998));
#62176=CARTESIAN_POINT('Ctrl Pts',(-31.509747524458,-0.644565823763341,
-1.48439008960595));
#62177=CARTESIAN_POINT('Ctrl Pts',(-31.4302038972409,0.900238933191302,
-1.34478582028906));
#62178=CARTESIAN_POINT('Ctrl Pts',(-31.3506602700238,1.61801242992563,0.0302459235288119));
#62179=CARTESIAN_POINT('Ctrl Pts',(-31.2711166428068,0.84935070414651,1.37749135048094));
#62180=CARTESIAN_POINT('Ctrl Pts',(-31.1915730155897,-0.699592297325916,
1.45926339528072));
#62181=CARTESIAN_POINT('Ctrl Pts',(-31.1120293883726,-1.60583403587161,
0.200439737877182));
#62182=CARTESIAN_POINT('Ctrl Pts',(-31.0324857611556,-1.03682859566712,
-1.24252384383195));
#62183=CARTESIAN_POINT('Ctrl Pts',(-30.9529421339385,0.484690259023074,
-1.54400595597689));
#62184=CARTESIAN_POINT('Ctrl Pts',(-30.8733985067214,1.56093399734461,-0.427041093125412));
#62185=CARTESIAN_POINT('Ctrl Pts',(-30.7938548795045,1.20317931219395,1.08223776592412));
#62186=CARTESIAN_POINT('Ctrl Pts',(-30.7143112522873,-0.259911818812566,
1.59728672620964));
#62187=CARTESIAN_POINT('Ctrl Pts',(-30.6347676250703,-1.48422723024795,
0.644940747878795));
#62188=CARTESIAN_POINT('Ctrl Pts',(-30.5552239978532,-1.34501317030866,
-0.89989922268008));
#62189=CARTESIAN_POINT('Ctrl Pts',(-30.4756803706362,0.0298372259863291,
-1.61802001817944));
#62190=CARTESIAN_POINT('Ctrl Pts',(-30.3961367434191,1.37727676756359,-0.849698619990381));
#62191=CARTESIAN_POINT('Ctrl Pts',(-30.3165931162021,1.45944005996512,0.699223677125539));
#62192=CARTESIAN_POINT('Ctrl Pts',(-30.237049488985,0.200845351898754,1.60578335522094));
#62193=CARTESIAN_POINT('Ctrl Pts',(-30.1575058617679,-1.2422619098531,1.03714241385265));
#62194=CARTESIAN_POINT('Ctrl Pts',(-30.0779622345509,-1.54412833547777,
-0.484300240407358));
#62195=CARTESIAN_POINT('Ctrl Pts',(-29.9984186073338,-0.427435358539164,
-1.56082608049534));
#62196=CARTESIAN_POINT('Ctrl Pts',(-29.9188749801167,1.08193381824142,-1.2034526381331));
#62197=CARTESIAN_POINT('Ctrl Pts',(-29.8393313528997,1.5973523268331,0.259508349085033));
#62198=CARTESIAN_POINT('Ctrl Pts',(-29.7597877256826,0.64531563084537,1.48406427619244));
#62199=CARTESIAN_POINT('Ctrl Pts',(-29.6802440984655,-0.899559454752963,
1.34524043451292));
#62200=CARTESIAN_POINT('Ctrl Pts',(-29.6007004712485,-1.61802750319939,
-0.0294285265401461));
#62201=CARTESIAN_POINT('Ctrl Pts',(-29.5211568440314,-0.85004648162128,
-1.37706209677242));
#62202=CARTESIAN_POINT('Ctrl Pts',(-29.4416132168144,0.698855012312891,
-1.45961663153347));
#62203=CARTESIAN_POINT('Ctrl Pts',(-29.3620695895973,1.60573257211715,-0.201250953105849));
#62204=CARTESIAN_POINT('Ctrl Pts',(-29.2825259623803,1.0374561658658,1.24199989661473));
#62205=CARTESIAN_POINT('Ctrl Pts',(-29.2029823351632,-0.483910190892033,
1.54425061645926));
#62206=CARTESIAN_POINT('Ctrl Pts',(-29.1234387079461,-1.56071806406133,
0.427829596681443));
#62207=CARTESIAN_POINT('Ctrl Pts',(-29.0438950807291,-1.20372588728886,
-1.08162980152852));
#62208=CARTESIAN_POINT('Ctrl Pts',(-28.964351453512,0.259104862800183,-1.59741782554135));
#62209=CARTESIAN_POINT('Ctrl Pts',(-28.884807826295,1.48390122744979,-0.645690472639149));
#62210=CARTESIAN_POINT('Ctrl Pts',(-28.8052641990779,1.34546761288737,0.899219629431616));
#62211=CARTESIAN_POINT('Ctrl Pts',(-28.7257205718609,-0.0290198252163337,
1.61803488498499));
#62212=CARTESIAN_POINT('Ctrl Pts',(-28.6461769446438,-1.37684733812111,
0.850394289017024));
#62213=CARTESIAN_POINT('Ctrl Pts',(-28.5666333174267,-1.4597931099745,-0.698486302911472));
#62214=CARTESIAN_POINT('Ctrl Pts',(-28.4870896902097,-0.201656541472631,
-1.60568168656345));
#62215=CARTESIAN_POINT('Ctrl Pts',(-28.4075460629926,1.24173780413355,-1.03776985168656));
#62216=CARTESIAN_POINT('Ctrl Pts',(-28.3280024357755,1.54437279891356,0.48352011050198));
#62217=CARTESIAN_POINT('Ctrl Pts',(-28.2484588085585,0.428223807527087,
1.56060994804947));
#62218=CARTESIAN_POINT('Ctrl Pts',(-28.1689151813414,-1.08132571580484,
1.20399905964379));
#62219=CARTESIAN_POINT('Ctrl Pts',(-28.0893715541244,-1.59748322233021,
-0.258701359983772));
#62220=CARTESIAN_POINT('Ctrl Pts',(-28.0098279269073,-0.646065273236205,
-1.4837380840304));
#62221=CARTESIAN_POINT('Ctrl Pts',(-27.9302842996902,0.898879746737731,
-1.34569470541749));
#62222=CARTESIAN_POINT('Ctrl Pts',(-27.8507406724732,1.61804216353577,0.0286111220409825));
#62223=CARTESIAN_POINT('Ctrl Pts',(-27.7711970452561,0.850742042155411,
1.37663249162338));
#62224=CARTESIAN_POINT('Ctrl Pts',(-27.6916534180391,-0.698117548944819,
1.45996949527695));
#62225=CARTESIAN_POINT('Ctrl Pts',(-27.612109790822,-1.60563069856312,0.202062116973198));
#62226=CARTESIAN_POINT('Ctrl Pts',(-27.532566163605,-1.03808347129492,-1.24147563242629));
#62227=CARTESIAN_POINT('Ctrl Pts',(-27.4530225363878,0.483129999262114,
-1.54449488283288));
#62228=CARTESIAN_POINT('Ctrl Pts',(-27.3734789091709,1.56050173246666,-0.42861799105092));
#62229=CARTESIAN_POINT('Ctrl Pts',(-27.2939352819538,1.20427215518044,1.08102156108979));
#62230=CARTESIAN_POINT('Ctrl Pts',(-27.2143916547367,-0.258297840661568,
1.5975485171955));
#62231=CARTESIAN_POINT('Ctrl Pts',(-27.1348480275197,-1.48357484594468,
0.6464400326126));
#62232=CARTESIAN_POINT('Ctrl Pts',(-27.0553044003026,-1.3459217120888,-0.898539806693006));
#62233=CARTESIAN_POINT('Ctrl Pts',(-26.9757607730855,0.0282024170401897,
-1.61804933885128));
#62234=CARTESIAN_POINT('Ctrl Pts',(-26.8962171458685,1.37641755729295,-0.851089741014233));
#62235=CARTESIAN_POINT('Ctrl Pts',(-26.8166735186514,1.46014578742956,0.697748750436479));
#62236=CARTESIAN_POINT('Ctrl Pts',(-26.7371298914343,0.202467679581668,
1.60557960811938));
#62237=CARTESIAN_POINT('Ctrl Pts',(-26.6575862642173,-1.24121338150966,
1.03839702467087));
#62238=CARTESIAN_POINT('Ctrl Pts',(-26.5780426370002,-1.54461686820943,
-0.482739857197281));
#62239=CARTESIAN_POINT('Ctrl Pts',(-26.4984990097832,-0.429012147227839,
-1.56039341731979));
#62240=CARTESIAN_POINT('Ctrl Pts',(-26.4189553825661,1.08071733740276,-1.20454517388143));
#62241=CARTESIAN_POINT('Ctrl Pts',(-26.3394117553491,1.59761371013306,0.257894304859269));
#62242=CARTESIAN_POINT('Ctrl Pts',(-26.259868128132,0.646814750744472,1.48341151320304));
#62243=CARTESIAN_POINT('Ctrl Pts',(-26.1803245009149,-0.898199809319099,
1.34614863288684));
#62244=CARTESIAN_POINT('Ctrl Pts',(-26.1007808736979,-1.61805641093105,
-0.0277937102399868));
#62245=CARTESIAN_POINT('Ctrl Pts',(-26.0212372464808,-0.851437385571346,
-1.3762025351435));
#62246=CARTESIAN_POINT('Ctrl Pts',(-25.9416936192638,0.697379907409941,
-1.4603219864211));
#62247=CARTESIAN_POINT('Ctrl Pts',(-25.8621499920467,1.60552841523551,-0.202873229272194));
#62248=CARTESIAN_POINT('Ctrl Pts',(-25.7826063648297,1.0387105117944,1.24095105140041));
#62249=CARTESIAN_POINT('Ctrl Pts',(-25.7030627376125,-0.482349684332396,
1.54473875503543));
#62250=CARTESIAN_POINT('Ctrl Pts',(-25.6235191103955,-1.56028500261578,
0.429406276032671));
#62251=CARTESIAN_POINT('Ctrl Pts',(-25.5439754831784,-1.20481811572932,
-1.08041304476317));
#62252=CARTESIAN_POINT('Ctrl Pts',(-25.4644318559614,0.257490752602664,
-1.59767880113873));
#62253=CARTESIAN_POINT('Ctrl Pts',(-25.3848882287443,1.48324808581591,-0.647189427607864));
#62254=CARTESIAN_POINT('Ctrl Pts',(-25.3053446015273,1.34637546779709,0.897859754637735));
#62255=CARTESIAN_POINT('Ctrl Pts',(-25.2258009743102,-0.0273850016665038,
1.61806337977463));
#62256=CARTESIAN_POINT('Ctrl Pts',(-25.1462573470932,-1.37598742518878,
0.851784975804522));
#62257=CARTESIAN_POINT('Ctrl Pts',(-25.0667137198762,-1.4604980922403,-0.697011019888793));
#62258=CARTESIAN_POINT('Ctrl Pts',(-24.987170092659,-0.20327876601885,-1.60547711991477));
#62259=CARTESIAN_POINT('Ctrl Pts',(-24.907626465442,1.24068864211528,-1.03902393264549));
#62260=CARTESIAN_POINT('Ctrl Pts',(-24.828082838225,1.54486054330308,0.481959480692382));
#62261=CARTESIAN_POINT('Ctrl Pts',(-24.7485392110078,0.429800377440236,
1.56017648836156));
#62262=CARTESIAN_POINT('Ctrl Pts',(-24.6689955837908,-1.08010868319043,
1.20509098070668));
#62263=CARTESIAN_POINT('Ctrl Pts',(-24.5894519565737,-1.59774379020835,
-0.257087183917484));
#62264=CARTESIAN_POINT('Ctrl Pts',(-24.5099083293567,-0.64756406317891,
-1.48308456379371));
#62265=CARTESIAN_POINT('Ctrl Pts',(-24.4303647021396,0.89751964267059,-1.3466022168051));
#62266=CARTESIAN_POINT('Ctrl Pts',(-24.3508210749226,1.61807024538158,0.0269762913457571));
#62267=CARTESIAN_POINT('Ctrl Pts',(-24.2712774477055,0.852132511691634,
1.37577222744249));
#62268=CARTESIAN_POINT('Ctrl Pts',(-24.1917338204884,-0.6966420878965,1.46067410487595));
#62269=CARTESIAN_POINT('Ctrl Pts',(-24.1121901932714,-1.60542572216043,
0.20368428979582));
#62270=CARTESIAN_POINT('Ctrl Pts',(-24.0326465660543,-1.03933728720419,
-1.24042615367099));
#62271=CARTESIAN_POINT('Ctrl Pts',(-23.9531029388373,0.481569246302081,
-1.54498223300464));
#62272=CARTESIAN_POINT('Ctrl Pts',(-23.8735593116202,1.56006787456402,-0.430194451425465));
#62273=CARTESIAN_POINT('Ctrl Pts',(-23.7940156844032,1.20536376879613,1.07980425270396));
#62274=CARTESIAN_POINT('Ctrl Pts',(-23.7144720571861,-0.256683598829453,
1.59780867733779));
#62275=CARTESIAN_POINT('Ctrl Pts',(-23.6349284299691,-1.48292094714688,
0.647938657433694));
#62276=CARTESIAN_POINT('Ctrl Pts',(-23.555384802752,-1.34682887989642,-0.89717947343935));
#62277=CARTESIAN_POINT('Ctrl Pts',(-23.4758411755349,0.0265675793038584,
-1.61807700775145));
#62278=CARTESIAN_POINT('Ctrl Pts',(-23.3962975483179,1.37555694191836,-0.852479993210494));
#62279=CARTESIAN_POINT('Ctrl Pts',(-23.3167539211008,1.46085002431682,0.696273111456646));
#62280=CARTESIAN_POINT('Ctrl Pts',(-23.2372102938837,0.204089800577218,
1.60537422197577));
#62281=CARTESIAN_POINT('Ctrl Pts',(-23.1576666666667,-1.2401635860843,1.03965057545047));
#62282=CARTESIAN_POINT('Ctrl Pts',(-23.0781230394496,-1.54510382413234,
-0.481178981186404));
#62283=CARTESIAN_POINT('Ctrl Pts',(-22.9985794122325,-0.430588497963164,
-1.55995916123012));
#62284=CARTESIAN_POINT('Ctrl Pts',(-22.9190357850155,1.07949975332317,-1.20563647998025));
#62285=CARTESIAN_POINT('Ctrl Pts',(-22.8394921577984,1.59787346252289,0.256279997364353));
#62286=CARTESIAN_POINT('Ctrl Pts',(-22.7599485305814,0.648313210348325,
1.48275723588584));
#62287=CARTESIAN_POINT('Ctrl Pts',(-22.6804049033644,-0.896839246965747,
1.34705545705657));
#62288=CARTESIAN_POINT('Ctrl Pts',(-22.6008612761472,-1.61808366688383,
-0.0261588655668692));
#62289=CARTESIAN_POINT('Ctrl Pts',(-22.5213176489302,-0.852827420338917,
-1.37534156863015));
#62290=CARTESIAN_POINT('Ctrl Pts',(-22.4417740217131,0.695904090592774,
-1.46102585055167));
#62291=CARTESIAN_POINT('Ctrl Pts',(-22.3622303944961,1.60532261936409,-0.204495298337127));
#62292=CARTESIAN_POINT('Ctrl Pts',(-22.282686767279,1.03996379736434,1.23990093937197));
#62293=CARTESIAN_POINT('Ctrl Pts',(-22.203143140062,-0.48078868537029,1.5452253166784));
#62294=CARTESIAN_POINT('Ctrl Pts',(-22.1235995128449,-1.5598503483668,0.430982517028184));
#62295=CARTESIAN_POINT('Ctrl Pts',(-22.0440558856279,-1.20590911424163,
-1.07919518506752));
#62296=CARTESIAN_POINT('Ctrl Pts',(-21.9645122584108,0.255876379547943,
-1.59793814575953));
#62297=CARTESIAN_POINT('Ctrl Pts',(-21.8849686311937,1.48259343002106,-0.648687721898869));
#62298=CARTESIAN_POINT('Ctrl Pts',(-21.8054250039767,1.34728194827107,0.896498963271491));
#62299=CARTESIAN_POINT('Ctrl Pts',(-21.7258813767596,-0.0257501501609023,
1.61809022277828));
#62300=CARTESIAN_POINT('Ctrl Pts',(-21.6463377495426,-1.37512610759159,
0.853174793054725));
#62301=CARTESIAN_POINT('Ctrl Pts',(-21.5667941223255,-1.46120158356928,
-0.695535025328411));
#62302=CARTESIAN_POINT('Ctrl Pts',(-21.4872504951084,-0.204900783049728,
-1.60527091432866));
#62303=CARTESIAN_POINT('Ctrl Pts',(-21.4077068678914,1.23963821355074,-1.04027695292585));
#62304=CARTESIAN_POINT('Ctrl Pts',(-21.3281632406743,1.5453467106351,0.480398358878597));
#62305=CARTESIAN_POINT('Ctrl Pts',(-21.2486196134573,0.431376508595433,
1.55974143598097));
#62306=CARTESIAN_POINT('Ctrl Pts',(-21.1690759862402,-1.07889054795642,
1.2061816715629));
#62307=CARTESIAN_POINT('Ctrl Pts',(-21.0895323590231,-1.59800272704358,
-0.25547274540593));
#62308=CARTESIAN_POINT('Ctrl Pts',(-21.0099887318061,-0.649062192061473,
-1.48242952956298));
#62309=CARTESIAN_POINT('Ctrl Pts',(-20.930445104589,0.896158622378259,-1.34750835352552));
#62310=CARTESIAN_POINT('Ctrl Pts',(-20.850901477372,1.61809667543438,0.0253414331119925));
#62311=CARTESIAN_POINT('Ctrl Pts',(-20.7713578501549,0.853522111335798,
1.37491055881641));
#62312=CARTESIAN_POINT('Ctrl Pts',(-20.6918142229379,-0.695165915687114,
1.46137722335845));
#62313=CARTESIAN_POINT('Ctrl Pts',(-20.6122705957208,-1.60521910687279,
0.205306254689137));
#62314=CARTESIAN_POINT('Ctrl Pts',(-20.5327269685037,-1.040590042115,-1.23937540863738));
#62315=CARTESIAN_POINT('Ctrl Pts',(-20.4531833412867,0.480008001736251,
-1.54546800599468));
#62316=CARTESIAN_POINT('Ctrl Pts',(-20.3736397140696,1.55963242407961,-0.431770472639713));
#62317=CARTESIAN_POINT('Ctrl Pts',(-20.2940960868525,1.20645415192664,1.07858584200931));
#62318=CARTESIAN_POINT('Ctrl Pts',(-20.2145524596354,-0.255069094964123,
1.59806720637092));
#62319=CARTESIAN_POINT('Ctrl Pts',(-20.1350088324184,-1.48226553452206,
0.64943662081221));
#62320=CARTESIAN_POINT('Ctrl Pts',(-20.0554652052013,-1.34773467280543,
-0.895818224307807));
#62321=CARTESIAN_POINT('Ctrl Pts',(-19.9759215779843,0.024932714446255,
-1.61810302485173));
#62322=CARTESIAN_POINT('Ctrl Pts',(-19.8963779507672,1.37469492231839,-0.853869375159925));
#62323=CARTESIAN_POINT('Ctrl Pts',(-19.8168343235502,1.46155276990797,0.694796761692446));
#62324=CARTESIAN_POINT('Ctrl Pts',(-19.7372906963331,0.205711713229446,
1.60516719699979));
#62325=CARTESIAN_POINT('Ctrl Pts',(-19.6577470691161,-1.23911252464868,
1.04090306491178));
#62326=CARTESIAN_POINT('Ctrl Pts',(-19.578203441899,-1.54558920274938,-0.479617613968146));
#62327=CARTESIAN_POINT('Ctrl Pts',(-19.4986598146819,-0.432164409135939,
-1.55952331266966));
#62328=CARTESIAN_POINT('Ctrl Pts',(-19.4191161874649,1.07828106724562,-1.2067265553155));
#62329=CARTESIAN_POINT('Ctrl Pts',(-19.3395725602478,1.59813158373743,0.254665428248228));
#62330=CARTESIAN_POINT('Ctrl Pts',(-19.2600289330308,0.649811008127239,
1.48210144490876));
#62331=CARTESIAN_POINT('Ctrl Pts',(-19.1804853058137,-0.895477769081822,
1.34796090609639));
#62332=CARTESIAN_POINT('Ctrl Pts',(-19.1009416785966,-1.61810927102991,
-0.0245239941897118));
#62333=CARTESIAN_POINT('Ctrl Pts',(-19.0213980513796,-0.854216584504992,
-1.37447919811127));
#62334=CARTESIAN_POINT('Ctrl Pts',(-18.9418544241625,0.694427563367922,
-1.46172822320664));
#62335=CARTESIAN_POINT('Ctrl Pts',(-18.8623107969455,1.60511518471297,-0.206117158644834));
#62336=CARTESIAN_POINT('Ctrl Pts',(-18.7827671697284,1.04121602129628,1.23884956160137));
#62337=CARTESIAN_POINT('Ctrl Pts',(-18.7032235425113,-0.479227195599194,
1.5457103008915));
#62338=CARTESIAN_POINT('Ctrl Pts',(-18.6236799152943,-1.55941410175808,
0.432558318058966));
#62339=CARTESIAN_POINT('Ctrl Pts',(-18.5441362880772,-1.20699888171208,
-1.0779762236848));
#62340=CARTESIAN_POINT('Ctrl Pts',(-18.4645926608602,0.254261745284025,
-1.59819585913902));
#62341=CARTESIAN_POINT('Ctrl Pts',(-18.3850490336431,1.48193726073355,-0.650185353982615));
#62342=CARTESIAN_POINT('Ctrl Pts',(-18.3055054064261,1.34818705338395,0.895137256722049));
#62343=CARTESIAN_POINT('Ctrl Pts',(-18.225961779209,-0.0241152723685061,
1.61811541396853));
#62344=CARTESIAN_POINT('Ctrl Pts',(-18.1464181519919,-1.37426338620882,
0.854563739348813));
#62345=CARTESIAN_POINT('Ctrl Pts',(-18.0668745247748,-1.46190358324326,
-0.694058320737146));
#62346=CARTESIAN_POINT('Ctrl Pts',(-17.9873308975578,-0.206522590909396,
-1.60506307001564));
#62347=CARTESIAN_POINT('Ctrl Pts',(-17.9077872703407,1.23858651951227,-1.04152891124848));
#62348=CARTESIAN_POINT('Ctrl Pts',(-17.8282436431237,1.5458313004133,0.478836746654323));
#62349=CARTESIAN_POINT('Ctrl Pts',(-17.7487000159066,0.432952199383627,
1.55930479135185));
#62350=CARTESIAN_POINT('Ctrl Pts',(-17.6691563886895,-1.07767131134634,
1.20727113109899));
#62351=CARTESIAN_POINT('Ctrl Pts',(-17.5896127614725,-1.59826003257156,
-0.253858046097263));
#62352=CARTESIAN_POINT('Ctrl Pts',(-17.5100691342554,-0.6505596583545,-1.48177298200691));
#62353=CARTESIAN_POINT('Ctrl Pts',(-17.4305255070384,0.89479668725018,-1.34841311465369));
#62354=CARTESIAN_POINT('Ctrl Pts',(-17.3509818798213,1.6181214536672,0.0237065490086662));
#62355=CARTESIAN_POINT('Ctrl Pts',(-17.2714382526043,0.854910839669279,
1.3740474866248));
#62356=CARTESIAN_POINT('Ctrl Pts',(-17.1918946253872,-0.693689033823637,
1.46207885000666));
#62357=CARTESIAN_POINT('Ctrl Pts',(-17.1123509981702,-1.60501085291113,
0.20692800999731));
#62358=CARTESIAN_POINT('Ctrl Pts',(-17.0328073709531,-1.04184173474845,
-1.23832339839813));
#62359=CARTESIAN_POINT('Ctrl Pts',(-16.953263743736,0.4784462671584,-1.54595220130706));
#62360=CARTESIAN_POINT('Ctrl Pts',(-16.873720116519,1.55919538145794,-0.433346053084831));
#62361=CARTESIAN_POINT('Ctrl Pts',(-16.7941764893019,1.2075433034589,1.07736633024962));
#62362=CARTESIAN_POINT('Ctrl Pts',(-16.7146328620849,-0.253454330713697,
1.59832410403098));
#62363=CARTESIAN_POINT('Ctrl Pts',(-16.6350892348678,-1.4816086087393,0.650933921219002));
#62364=CARTESIAN_POINT('Ctrl Pts',(-16.5555456076507,-1.34863908989118,
-0.894456060687972));
#62365=CARTESIAN_POINT('Ctrl Pts',(-16.4760019804337,0.0232978241362747,
-1.61812739012554));
#62366=CARTESIAN_POINT('Ctrl Pts',(-16.3964583532166,1.373831499373,-0.855257885444212));
#62367=CARTESIAN_POINT('Ctrl Pts',(-16.3169147259995,1.46225402348564,0.693319702650978));
#62368=CARTESIAN_POINT('Ctrl Pts',(-16.2373710987825,0.207333415882653,
1.60495853340278));
#62369=CARTESIAN_POINT('Ctrl Pts',(-16.1578274715654,-1.23806019827577,
1.04215449177621));
#62370=CARTESIAN_POINT('Ctrl Pts',(-16.0782838443484,-1.54607300356507,
-0.478055757136395));
#62371=CARTESIAN_POINT('Ctrl Pts',(-15.9987402171313,-0.43373987913742,
-1.55908587208332));
#62372=CARTESIAN_POINT('Ctrl Pts',(-15.9191965899143,1.07706128041417,-1.20781539877439));
#62373=CARTESIAN_POINT('Ctrl Pts',(-15.8396529626972,1.59838807351318,0.253050599159107));
#62374=CARTESIAN_POINT('Ctrl Pts',(-15.7601093354801,0.65130814255221,1.48144414094125));
#62375=CARTESIAN_POINT('Ctrl Pts',(-15.6805657082631,-0.894115377057167,
1.348864979082));
#62376=CARTESIAN_POINT('Ctrl Pts',(-15.601022081046,-1.61813322334315,-0.0228890977774511));
#62377=CARTESIAN_POINT('Ctrl Pts',(-15.521478453829,-0.85560487665146,-1.3736154244672));
#62378=CARTESIAN_POINT('Ctrl Pts',(-15.4419348266119,0.692950327242719,
-1.46242910366902));
#62379=CARTESIAN_POINT('Ctrl Pts',(-15.3623911993948,1.60490611149391,-0.207738808539605));
#62380=CARTESIAN_POINT('Ctrl Pts',(-15.2828475721778,1.04246718231184,1.23779691916194));
#62381=CARTESIAN_POINT('Ctrl Pts',(-15.2033039449607,-0.477665216613179,
1.54619370717962));
#62382=CARTESIAN_POINT('Ctrl Pts',(-15.1237603177437,-1.55897626323499,
0.434133677516307));
#62383=CARTESIAN_POINT('Ctrl Pts',(-15.0442166905266,-1.20808741702816,
-1.07675616185941));
#62384=CARTESIAN_POINT('Ctrl Pts',(-14.9646730633095,0.252646851459204,
-1.59845194101409));
#62385=CARTESIAN_POINT('Ctrl Pts',(-14.8851294360925,1.48127957862323,-0.65168232233028));
#62386=CARTESIAN_POINT('Ctrl Pts',(-14.8055858088754,1.34909078221174,0.893774636379497));
#62387=CARTESIAN_POINT('Ctrl Pts',(-14.7260421816584,-0.0224803699582582,
1.61813895331967));
#62388=CARTESIAN_POINT('Ctrl Pts',(-14.6464985544413,-1.37339926192116,
0.855951813268913));
#62389=CARTESIAN_POINT('Ctrl Pts',(-14.5669549272242,-1.46260409054564,
-0.692580907622451));
#62390=CARTESIAN_POINT('Ctrl Pts',(-14.4874113000072,-0.208144187942263,
-1.60485358718789));
#62391=CARTESIAN_POINT('Ctrl Pts',(-14.4078676727901,1.23753356107348,-1.04277980633532));
#62392=CARTESIAN_POINT('Ctrl Pts',(-14.3283240455731,1.546314312143,0.477274645613715));
#62393=CARTESIAN_POINT('Ctrl Pts',(-14.248780418356,0.434527448196287,1.55886655491996));
#62394=CARTESIAN_POINT('Ctrl Pts',(-14.1692367911389,-1.07645097460485,
1.20835935820277));
#62395=CARTESIAN_POINT('Ctrl Pts',(-14.0896931639219,-1.59851570652962,
-0.252243087639847));
#62396=CARTESIAN_POINT('Ctrl Pts',(-14.0101495367048,-0.652056460529289,
-1.48111492179574));
#62397=CARTESIAN_POINT('Ctrl Pts',(-13.9306059094878,0.893433838676696,
-1.34931649926596));
#62398=CARTESIAN_POINT('Ctrl Pts',(-13.8510622822707,1.61814458005474,0.0220716407047407));
#62399=CARTESIAN_POINT('Ctrl Pts',(-13.7715186550536,0.8562986952744,1.37318301174874));
#62400=CARTESIAN_POINT('Ctrl Pts',(-13.6919750278366,-0.692211443813764,
1.46277898410431));
#62401=CARTESIAN_POINT('Ctrl Pts',(-13.6124314006195,-1.60480096048804,
0.208549554064757));
#62402=CARTESIAN_POINT('Ctrl Pts',(-13.5328877734025,-1.04309236382677,
-1.23727012402718));
#62403=CARTESIAN_POINT('Ctrl Pts',(-13.4533441461854,0.47688404416288,-1.54643481844753));
#62404=CARTESIAN_POINT('Ctrl Pts',(-13.3738005189684,1.55875674714518,-0.434921191152319));
#62405=CARTESIAN_POINT('Ctrl Pts',(-13.2942568917513,1.20863122228096,1.07614571866991));
#62406=CARTESIAN_POINT('Ctrl Pts',(-13.2147132645342,-0.251839307726659,
1.59857937005571));
#62407=CARTESIAN_POINT('Ctrl Pts',(-13.1351696373171,-1.48095017046926,
0.652430557125475));
#62408=CARTESIAN_POINT('Ctrl Pts',(-13.0556260101001,-1.34954213023036,
-0.893092983970473));
#62409=CARTESIAN_POINT('Ctrl Pts',(-12.976082382883,0.0216629100430018,
-1.618150103548));
#62410=CARTESIAN_POINT('Ctrl Pts',(-12.896538755666,1.37296667396363,-0.856645522645844));
#62411=CARTESIAN_POINT('Ctrl Pts',(-12.8169951284489,1.46295378433393,0.691841935840126));
#62412=CARTESIAN_POINT('Ctrl Pts',(-12.7374515012319,0.208954906881307,
1.60474823139775));
#62413=CARTESIAN_POINT('Ctrl Pts',(-12.6579078740148,-1.23700660803984,
1.04340485476622));
#62414=CARTESIAN_POINT('Ctrl Pts',(-12.5783642467977,-1.5465552260855,-0.476493412285577));
#62415=CARTESIAN_POINT('Ctrl Pts',(-12.4988206195807,-0.43531490635929,
-1.55864683991769));
#62416=CARTESIAN_POINT('Ctrl Pts',(-12.4192769923636,1.07584039407407,-1.20890300924538));
#62417=CARTESIAN_POINT('Ctrl Pts',(-12.3397333651465,1.59864293158829,0.251435511745501));
#62418=CARTESIAN_POINT('Ctrl Pts',(-12.2601897379295,0.652804612094871,
1.48078532465434));
#62419=CARTESIAN_POINT('Ctrl Pts',(-12.1806461107124,-0.892752072282623,
1.34976767509045));
#62420=CARTESIAN_POINT('Ctrl Pts',(-12.1011024834954,-1.61815552379909,
-0.0212541779991121));
#62421=CARTESIAN_POINT('Ctrl Pts',(-12.0215588562783,-0.856992295361072,
-1.37275024857972));
#62422=CARTESIAN_POINT('Ctrl Pts',(-11.9420152290613,0.691472383725218,
-1.4631284912233));
#62423=CARTESIAN_POINT('Ctrl Pts',(-11.8624716018442,1.60469539992036,-0.209360246365963));
#62424=CARTESIAN_POINT('Ctrl Pts',(-11.7829279746271,1.04371727913374,1.23674301312827));
#62425=CARTESIAN_POINT('Ctrl Pts',(-11.7033843474101,-0.476102750006793,
1.54667553504926));
#62426=CARTESIAN_POINT('Ctrl Pts',(-11.623840720193,-1.55853683324449,0.435708593792007));
#62427=CARTESIAN_POINT('Ctrl Pts',(-11.544297092976,-1.20917471907862,-1.07553500083685));
#62428=CARTESIAN_POINT('Ctrl Pts',(-11.4647534657589,0.251031699722106,
-1.59870639112332));
#62429=CARTESIAN_POINT('Ctrl Pts',(-11.3852098385419,1.48062038436146,-0.65317862541366));
#62430=CARTESIAN_POINT('Ctrl Pts',(-11.3056662113248,1.34999313383188,0.892411103634845));
#62431=CARTESIAN_POINT('Ctrl Pts',(-11.2261225841077,-0.0208454445991207,
1.61816084080769));
#62432=CARTESIAN_POINT('Ctrl Pts',(-11.1465789568907,-1.3725337356108,0.85733901339797));
#62433=CARTESIAN_POINT('Ctrl Pts',(-11.0670353296736,-1.46330310476127,
-0.691102787492547));
#62434=CARTESIAN_POINT('Ctrl Pts',(-10.9874917024566,-0.209765572492934,
-1.60464246605925));
#62435=CARTESIAN_POINT('Ctrl Pts',(-10.9079480752395,1.23647933930929,-1.04402963690943));
#62436=CARTESIAN_POINT('Ctrl Pts',(-10.8284044480224,1.54679574533111,0.475712057351421));
#62437=CARTESIAN_POINT('Ctrl Pts',(-10.7488608208054,0.43610225342541,1.5584267271326));
#62438=CARTESIAN_POINT('Ctrl Pts',(-10.6693171935883,-1.07522953897768,
1.20944635176342));
#62439=CARTESIAN_POINT('Ctrl Pts',(-10.5897735663712,-1.59876974865677,
-0.250627871682214));
#62440=CARTESIAN_POINT('Ctrl Pts',(-10.5102299391542,-0.65355259705794,
-1.48045534960118));
#62441=CARTESIAN_POINT('Ctrl Pts',(-10.4306863119371,0.892070078048929,
-1.35021850644024));
#62442=CARTESIAN_POINT('Ctrl Pts',(-10.3511426847201,1.61816605457342,0.0204367098691262));
#62443=CARTESIAN_POINT('Ctrl Pts',(-10.271599057503,0.857685676734452,1.37231713507066));
#62444=CARTESIAN_POINT('Ctrl Pts',(-10.1920554302859,-0.690733147165762,
1.46347762493672));
#62445=CARTESIAN_POINT('Ctrl Pts',(-10.1125118030689,-1.60458942981779,
0.210170885236279));
#62446=CARTESIAN_POINT('Ctrl Pts',(-10.0329681758518,-1.0443419280733,-1.23621558659974));
#62447=CARTESIAN_POINT('Ctrl Pts',(-9.95342454863478,0.475321334344385,
-1.54691585692338));
#62448=CARTESIAN_POINT('Ctrl Pts',(-9.87388092141771,1.55831652158906,-0.436495885234337));
#62449=CARTESIAN_POINT('Ctrl Pts',(-9.79433729420066,1.20971790728238,1.07492400851611));
#62450=CARTESIAN_POINT('Ctrl Pts',(-9.7147936669836,-0.250224027651638,
1.59883300418455));
#62451=CARTESIAN_POINT('Ctrl Pts',(-9.63525003976653,-1.48029022038403,
0.653926527003873));
#62452=CARTESIAN_POINT('Ctrl Pts',(-9.55570641254947,-1.35044379290116,
-0.891728995546662));
#62453=CARTESIAN_POINT('Ctrl Pts',(-9.47616278533242,0.020027973835256,
-1.61817116509597));
#62454=CARTESIAN_POINT('Ctrl Pts',(-9.39661915811536,1.37210044697314,-0.858032285348334));
#62455=CARTESIAN_POINT('Ctrl Pts',(-9.3170755308983,1.46365205173851,0.690363462768413));
#62456=CARTESIAN_POINT('Ctrl Pts',(-9.23753190368124,0.210576184570202,
1.60453629119936));
#62457=CARTESIAN_POINT('Ctrl Pts',(-9.15798827646418,-1.23595175501641,
1.04465415260547));
#62458=CARTESIAN_POINT('Ctrl Pts',(-9.07844464924712,-1.54703586981845,
-0.474930581010598));
#62459=CARTESIAN_POINT('Ctrl Pts',(-8.99890102203006,-0.436889489193695,
-1.5582062166209));
#62460=CARTESIAN_POINT('Ctrl Pts',(-8.919357394813,1.07461840947157,-1.20998938561821));
#62461=CARTESIAN_POINT('Ctrl Pts',(-8.83981376759594,1.59889615770264,0.249820167656086));
#62462=CARTESIAN_POINT('Ctrl Pts',(-8.76027014037887,0.654300415227634,
1.48012499672052));
#62463=CARTESIAN_POINT('Ctrl Pts',(-8.68072651316183,-0.891387856149781,
1.35066899320027));
#62464=CARTESIAN_POINT('Ctrl Pts',(-8.60118288594476,-1.61817617237499,
-0.0196192365235215));
#62465=CARTESIAN_POINT('Ctrl Pts',(-8.5216392587277,-0.858378839217572,
-1.37188367133204));
#62466=CARTESIAN_POINT('Ctrl Pts',(-8.44209563151065,0.689993734324072,
-1.46382638515553));
#62467=CARTESIAN_POINT('Ctrl Pts',(-8.36255200429358,1.60448305020737,-0.210981470468792));
#62468=CARTESIAN_POINT('Ctrl Pts',(-8.28300837707653,1.04496631048598,1.23568784457617));
#62469=CARTESIAN_POINT('Ctrl Pts',(-8.20346474985946,-0.47453979737503,
1.5471557840086));
#62470=CARTESIAN_POINT('Ctrl Pts',(-8.12392112264241,-1.55809581223514,
0.437283065278374));
#62471=CARTESIAN_POINT('Ctrl Pts',(-8.04437749542533,-1.21026078675358,
-1.07431274186363));
#62472=CARTESIAN_POINT('Ctrl Pts',(-7.96483386820829,0.249416291721394,
-1.59895920920702));
#62473=CARTESIAN_POINT('Ctrl Pts',(-7.88529024099122,1.47995967862121,-0.654674261705304));
#62474=CARTESIAN_POINT('Ctrl Pts',(-7.80574661377416,1.3508941073232,0.891046659880044));
#62475=CARTESIAN_POINT('Ctrl Pts',(-7.72620298655711,-0.0192104979600539,
1.6181810764102));
#62476=CARTESIAN_POINT('Ctrl Pts',(-7.64665935934005,-1.37166680816123,
0.858725338319981));
#62477=CARTESIAN_POINT('Ctrl Pts',(-7.56711573212298,-1.46400062517662,
-0.689623961856359));
#62478=CARTESIAN_POINT('Ctrl Pts',(-7.48757210490593,-0.211386742906221,
-1.60442970684522));
#62479=CARTESIAN_POINT('Ctrl Pts',(-7.40802847768886,1.23542385529583,-1.04527840169494));
#62480=CARTESIAN_POINT('Ctrl Pts',(-7.32848485047181,1.54727559948621,0.47414898346256));
#62481=CARTESIAN_POINT('Ctrl Pts',(-7.24894122325474,0.437676613463291,
1.55798530843885));
#62482=CARTESIAN_POINT('Ctrl Pts',(-7.16939759603769,-1.07400700571175,
1.21053211067118));
#62483=CARTESIAN_POINT('Ctrl Pts',(-7.08985396882063,-1.59902215869365,
-0.24901239987327));
#62484=CARTESIAN_POINT('Ctrl Pts',(-7.01031034160357,-0.655048066413094,
-1.47979426609663));
#62485=CARTESIAN_POINT('Ctrl Pts',(-6.93076671438651,0.89070540675921,-1.35111913525562));
#62486=CARTESIAN_POINT('Ctrl Pts',(-6.85122308716945,1.61818587720126,0.0188017581709107));
#62487=CARTESIAN_POINT('Ctrl Pts',(-6.77167945995239,0.859071782633506,
1.3714498574745));
#62488=CARTESIAN_POINT('Ctrl Pts',(-6.69213583273532,-0.689254145388818,
1.46417477179069));
#62489=CARTESIAN_POINT('Ctrl Pts',(-6.61259220551828,-1.60437626111631,
0.211792001856658));
#62490=CARTESIAN_POINT('Ctrl Pts',(-6.5330485783012,-1.04559042621242,-1.23515978719228));
#62491=CARTESIAN_POINT('Ctrl Pts',(-6.45350495108415,0.473758139298161,
-1.54739531624361));
#62492=CARTESIAN_POINT('Ctrl Pts',(-6.37396132386709,1.55787470523904,-0.438070133723317));
#62493=CARTESIAN_POINT('Ctrl Pts',(-6.29441769665004,1.21080335735372,1.07370120103544));
#62494=CARTESIAN_POINT('Ctrl Pts',(-6.21487406943297,-0.24860849213754,
1.59908500615853));
#62495=CARTESIAN_POINT('Ctrl Pts',(-6.13533044221592,-1.47962875915735,
0.655421829327089));
#62496=CARTESIAN_POINT('Ctrl Pts',(-6.05578681499884,-1.35134407698311,
-0.89036409680908));
#62497=CARTESIAN_POINT('Ctrl Pts',(-5.9762431877818,0.0183930171821651,
-1.61819057474788));
#62498=CARTESIAN_POINT('Ctrl Pts',(-5.89669956056472,1.37123281928574,-0.859418172136015));
#62499=CARTESIAN_POINT('Ctrl Pts',(-5.81715593334767,1.4643488249866,0.688884284945115));
#62500=CARTESIAN_POINT('Ctrl Pts',(-5.73761230613061,0.212197247294186,
1.60432271302402));
#62501=CARTESIAN_POINT('Ctrl Pts',(-5.65806867891356,-1.23489564028233,
1.04590238401853));
#62502=CARTESIAN_POINT('Ctrl Pts',(-5.57852505169649,-1.5475149342732,-0.4733672649068));
#62503=CARTESIAN_POINT('Ctrl Pts',(-5.49898142447944,-0.438463626033293,
-1.5577640026428));
#62504=CARTESIAN_POINT('Ctrl Pts',(-5.41943779726238,1.07339532785422,-1.21107452678385));
#62505=CARTESIAN_POINT('Ctrl Pts',(-5.3398941700453,1.59914775159766,0.248204568539948));
#62506=CARTESIAN_POINT('Ctrl Pts',(-5.26035054282826,0.655795550423491,
1.4794631578139));
#62507=CARTESIAN_POINT('Ctrl Pts',(-5.18080691561119,-0.890022730051382,
1.35156893249138));
#62508=CARTESIAN_POINT('Ctrl Pts',(-5.10126328839414,-1.61819516904976,
-0.0179842750198703));
#62509=CARTESIAN_POINT('Ctrl Pts',(-5.02171966117707,-0.859764506805417,
-1.37101569360878));
#62510=CARTESIAN_POINT('Ctrl Pts',(-4.94217603396002,0.688514380548778,
-1.46452278475327));
#62511=CARTESIAN_POINT('Ctrl Pts',(-4.86263240674296,1.60426906257179,-0.212602479193019));
#62512=CARTESIAN_POINT('Ctrl Pts',(-4.7830887795259,1.04621427509339,1.23463141458283));
#62513=CARTESIAN_POINT('Ctrl Pts',(-4.70354515230884,-0.472976360313382,
1.54763445356733));
#62514=CARTESIAN_POINT('Ctrl Pts',(-4.62400152509178,-1.55765320065716,
0.438857090368179));
#62515=CARTESIAN_POINT('Ctrl Pts',(-4.54445789787472,-1.21134561894431,
-1.07308938618757));
#62516=CARTESIAN_POINT('Ctrl Pts',(-4.46491427065766,0.247800629106233,
-1.59921039500703));
#62517=CARTESIAN_POINT('Ctrl Pts',(-4.3853706434406,1.4792974620769,-0.656169229678419));
#62518=CARTESIAN_POINT('Ctrl Pts',(-4.30582701622354,1.35179370176602,0.88968130650793));
#62519=CARTESIAN_POINT('Ctrl Pts',(-4.22628338900648,-0.0175755317101194,
1.61819966010659));
#62520=CARTESIAN_POINT('Ctrl Pts',(-4.14673976178942,-1.37079848045747,
0.860110786619649));
#62521=CARTESIAN_POINT('Ctrl Pts',(-4.06719613457236,-1.46469665107959,
-0.688144432223473));
#62522=CARTESIAN_POINT('Ctrl Pts',(-3.9876525073553,-0.213007697527226,
-1.60421530976304));
#62523=CARTESIAN_POINT('Ctrl Pts',(-3.90810888013824,1.23436711011067,-1.04652609941703));
#62524=CARTESIAN_POINT('Ctrl Pts',(-3.82856525292118,1.54775387411837,0.472585425542845));
#62525=CARTESIAN_POINT('Ctrl Pts',(-3.74902162570412,0.439250526702823,
1.55754229928924));
#62526=CARTESIAN_POINT('Ctrl Pts',(-3.66947799848706,-1.07278337605506,
1.21161663381776));
#62527=CARTESIAN_POINT('Ctrl Pts',(-3.58993437127001,-1.59927293638262,
-0.247396673862219));
#62528=CARTESIAN_POINT('Ctrl Pts',(-3.51039074405294,-0.656542867068056,
-1.4791316719569));
#62529=CARTESIAN_POINT('Ctrl Pts',(-3.43084711683588,0.889339826200543,
-1.35201838479272));
#62530=CARTESIAN_POINT('Ctrl Pts',(-3.35130348961882,1.61820404791809,0.017166787279032));
#62531=CARTESIAN_POINT('Ctrl Pts',(-3.27175986240176,0.860457011556571,
1.37058117984569));
#62532=CARTESIAN_POINT('Ctrl Pts',(-3.1922162351847,-0.687774439992805,
1.46487042395443));
#62533=CARTESIAN_POINT('Ctrl Pts',(-3.11267260796765,-1.60416145460112,
0.213412902271105));
#62534=CARTESIAN_POINT('Ctrl Pts',(-3.03312898075058,-1.04683785696976,
-1.23410272688283));
#62535=CARTESIAN_POINT('Ctrl Pts',(-2.95358535353353,0.472194460620347,
-1.54787319591841));
#62536=CARTESIAN_POINT('Ctrl Pts',(-2.87404172631646,1.55743129854565,-0.439643935012751));
#62537=CARTESIAN_POINT('Ctrl Pts',(-2.79449809909941,1.21188757138778,1.07247729747732));
#62538=CARTESIAN_POINT('Ctrl Pts',(-2.71495447188235,-0.246992702835222,
1.59933537571829));
#62539=CARTESIAN_POINT('Ctrl Pts',(-2.63541084466529,-1.47896578746142,
0.656916462572719));
#62540=CARTESIAN_POINT('Ctrl Pts',(-2.55586721744822,-1.35224298156292,
-0.888998289158813));
#62541=CARTESIAN_POINT('Ctrl Pts',(-2.47632359023117,0.0167580417635838,
-1.61820833246908));
#62542=CARTESIAN_POINT('Ctrl Pts',(-2.39677996301411,1.37036379176648,-0.860803181622379));
#62543=CARTESIAN_POINT('Ctrl Pts',(-2.31723633579705,1.46504410340623,0.687404403933919));
#62544=CARTESIAN_POINT('Ctrl Pts',(-2.23769270857999,0.21381809332376,1.60410749698785));
#62545=CARTESIAN_POINT('Ctrl Pts',(-2.15814908136293,-1.2338382647739,1.04714954792454));
#62546=CARTESIAN_POINT('Ctrl Pts',(-2.07860545414587,-1.54799241922993,
-0.471803465937055));
#62547=CARTESIAN_POINT('Ctrl Pts',(-1.99906182692881,-0.440037314760149,
-1.55732019773846));
#62548=CARTESIAN_POINT('Ctrl Pts',(-1.91951819971175,1.07217114950081,-1.21215843295618));
#62549=CARTESIAN_POINT('Ctrl Pts',(-1.83997457249469,1.59939771485701,0.246588718554731));
#62550=CARTESIAN_POINT('Ctrl Pts',(-1.76043094527763,0.657290012662976,
1.47879980384918));
#62551=CARTESIAN_POINT('Ctrl Pts',(-1.68088731806057,-0.888656688751067,
1.35246750108129));
#62552=CARTESIAN_POINT('Ctrl Pts',(-1.60134369084351,-1.61821252638751,
-0.016349312307876));
#62553=CARTESIAN_POINT('Ctrl Pts',(-1.52180006362645,-0.861149272826775,
-1.37014628374404));
#62554=CARTESIAN_POINT('Ctrl Pts',(-1.44225643640939,0.687034278579223,
-1.46521775108889));
#62555=CARTESIAN_POINT('Ctrl Pts',(-1.36271280919233,1.60405352326847,-0.214223153619904));
#62556=CARTESIAN_POINT('Ctrl Pts',(-1.28316918197528,1.04746100838583,1.23357350166125));
#62557=CARTESIAN_POINT('Ctrl Pts',(-1.20362555475821,-0.47141213048378,
1.54811196566333));
#62558=CARTESIAN_POINT('Ctrl Pts',(-1.12408192754115,-1.55720958721362,
0.440429865694213));
#62559=CARTESIAN_POINT('Ctrl Pts',(-1.04453830032409,-1.21242809804978,
-1.07186341332639));
#62560=CARTESIAN_POINT('Ctrl Pts',(-0.964994673107033,0.246182594434854,
-1.59946283649398));
#62561=CARTESIAN_POINT('Ctrl Pts',(-0.885451045889976,1.47863775741399,
-0.657658045986899));
#62562=CARTESIAN_POINT('Ctrl Pts',(-0.805907418672914,1.352684282513,0.888304640480979));
#62563=CARTESIAN_POINT('Ctrl Pts',(-0.726363791455857,-0.0159260587564186,
1.61823633939855));
#62564=CARTESIAN_POINT('Ctrl Pts',(-0.646820164238798,-1.36995625320173,
0.861457876012838));
#62565=CARTESIAN_POINT('Ctrl Pts',(-0.567276537021739,-1.46533898470946,
-0.686593059182217));
#62566=CARTESIAN_POINT('Ctrl Pts',(-0.487732909804673,-0.214727527229581,
-1.60413432240554));
#62567=CARTESIAN_POINT('Ctrl Pts',(-0.408189282587616,1.23349737730688,
-1.04751621777734));
#62568=CARTESIAN_POINT('Ctrl Pts',(-0.328645655370557,1.54787157060309,
0.470532899021241));
#62569=CARTESIAN_POINT('Ctrl Pts',(-0.249102028153498,0.441519398461233,
1.55803864581879));
#62570=CARTESIAN_POINT('Ctrl Pts',(-0.169558400936438,-1.07299616020733,
1.21079737759236));
#62571=CARTESIAN_POINT('Ctrl Pts',(-0.116529316125065,-1.42161642106954,
0.242796052776739));
#62572=CARTESIAN_POINT('Ctrl Pts',(-0.0900147737193787,-1.35237762530129,
-0.207804766751035));
#62573=CARTESIAN_POINT('Ctrl Pts',(-34.6365,-0.63400709457496,1.31904027763697));
#62574=CARTESIAN_POINT('Ctrl Pts',(-34.6099854575943,-1.07350019101018,
1.10779446059807));
#62575=CARTESIAN_POINT('Ctrl Pts',(-34.5569563727829,-1.71702895747196,
0.215076187392512));
#62576=CARTESIAN_POINT('Ctrl Pts',(-34.4774127455659,-1.10807355631996,
-1.33132370591566));
#62577=CARTESIAN_POINT('Ctrl Pts',(-34.3978691183488,0.520314157757823,
-1.65035441174038));
#62578=CARTESIAN_POINT('Ctrl Pts',(-34.3183254911318,1.66994567305946,-0.45540337748486));
#62579=CARTESIAN_POINT('Ctrl Pts',(-34.2387818639147,1.28582705277904,1.1590459348403));
#62580=CARTESIAN_POINT('Ctrl Pts',(-34.1592382366976,-0.279762724963516,
1.70811017633449));
#62581=CARTESIAN_POINT('Ctrl Pts',(-34.0796946094806,-1.58823064801099,
0.688280517758478));
#62582=CARTESIAN_POINT('Ctrl Pts',(-34.0001509822635,-1.43768096220901,
-0.964023021038801));
#62583=CARTESIAN_POINT('Ctrl Pts',(-33.9206073550465,0.0336674791827454,
-1.73061147221349));
#62584=CARTESIAN_POINT('Ctrl Pts',(-33.8410637278294,1.47407027445902,-0.907367911586003));
#62585=CARTESIAN_POINT('Ctrl Pts',(-33.7615201006124,1.56028302586567,0.749480218709788));
#62586=CARTESIAN_POINT('Ctrl Pts',(-33.6819764733952,0.213090942288775,
1.71778338655393));
#62587=CARTESIAN_POINT('Ctrl Pts',(-33.6024328461783,-1.32986112826589,
1.10800045574547));
#62588=CARTESIAN_POINT('Ctrl Pts',(-33.5228892189612,-1.65109797050015,
-0.519683553947057));
#62589=CARTESIAN_POINT('Ctrl Pts',(-33.4433455917441,-0.455503924497776,
-1.66994296236554));
#62590=CARTESIAN_POINT('Ctrl Pts',(-33.3638019645271,1.15855200135494,-1.28606059765399));
#62591=CARTESIAN_POINT('Ctrl Pts',(-33.28425833731,1.70826986773391,0.27930008458429));
#62592=CARTESIAN_POINT('Ctrl Pts',(-33.2047147100929,0.688634737886851,
1.58807316929715));
#62593=CARTESIAN_POINT('Ctrl Pts',(-33.1251710828759,-0.963635117031397,
1.43791576625308));
#62594=CARTESIAN_POINT('Ctrl Pts',(-33.0456274556588,-1.73063294906621,
-0.0332257802001231));
#62595=CARTESIAN_POINT('Ctrl Pts',(-32.9660838284418,-0.907733356543969,
-1.47384343620158));
#62596=CARTESIAN_POINT('Ctrl Pts',(-32.8865402012247,0.749082463693335,
-1.56047102283841));
#62597=CARTESIAN_POINT('Ctrl Pts',(-32.8069965740076,1.71773141218131,-0.213525500287109));
#62598=CARTESIAN_POINT('Ctrl Pts',(-32.7274529467906,1.10833532841135,1.32958156544835));
#62599=CARTESIAN_POINT('Ctrl Pts',(-32.6479093195735,-0.519265954714281,
1.65122900047349));
#62600=CARTESIAN_POINT('Ctrl Pts',(-32.5683656923565,-1.66982813124843,
0.45592582130719));
#62601=CARTESIAN_POINT('Ctrl Pts',(-32.4888220651394,-1.28635305046249,
-1.15822716750039));
#62602=CARTESIAN_POINT('Ctrl Pts',(-32.4092784379224,0.27886850345117,-1.70834033505615));
#62603=CARTESIAN_POINT('Ctrl Pts',(-32.3297348107052,1.58789921594784,-0.689035864352048));
#62604=CARTESIAN_POINT('Ctrl Pts',(-32.2501911834882,1.43815910517878,0.963271888158851));
#62605=CARTESIAN_POINT('Ctrl Pts',(-32.1706475562711,-0.0327886242346749,
1.7306412824543));
#62606=CARTESIAN_POINT('Ctrl Pts',(-32.0911039290542,-1.47361410919611,
0.908105610353001));
#62607=CARTESIAN_POINT('Ctrl Pts',(-32.011560301837,-1.56066018196052,-0.748688278802587));
#62608=CARTESIAN_POINT('Ctrl Pts',(-31.93201667462,-0.213959379899255,-1.71767742202626));
#62609=CARTESIAN_POINT('Ctrl Pts',(-31.8524730474029,1.32930156755401,-1.1086711346824));
#62610=CARTESIAN_POINT('Ctrl Pts',(-31.7729294201859,1.65136010962961,0.518848851500797));
#62611=CARTESIAN_POINT('Ctrl Pts',(-31.6933857929688,0.456347591800452,
1.66971291479679));
#62612=CARTESIAN_POINT('Ctrl Pts',(-31.6138421657518,-1.15790220852164,
1.2866455680882));
#62613=CARTESIAN_POINT('Ctrl Pts',(-31.5342985385347,-1.70841072037166,
-0.27843698191794));
#62614=CARTESIAN_POINT('Ctrl Pts',(-31.4547549113176,-0.689436932634756,
-1.58772512051041));
#62615=CARTESIAN_POINT('Ctrl Pts',(-31.3752112841006,0.962908590334806,
-1.43840237383004));
#62616=CARTESIAN_POINT('Ctrl Pts',(-31.2956676568835,1.73064950937048,0.0323514774964916));
#62617=CARTESIAN_POINT('Ctrl Pts',(-31.2161240296665,0.908477804142727,
1.47338468220642));
#62618=CARTESIAN_POINT('Ctrl Pts',(-31.1365804024494,-0.748294045047776,
1.56084924465066));
#62619=CARTESIAN_POINT('Ctrl Pts',(-31.0570367752323,-1.71762332285629,
0.214393244204715));
#62620=CARTESIAN_POINT('Ctrl Pts',(-30.9774931480153,-1.10900686991318,
-1.32902148397453));
#62621=CARTESIAN_POINT('Ctrl Pts',(-30.8979495207982,0.518431715023144,
-1.65149111388425));
#62622=CARTESIAN_POINT('Ctrl Pts',(-30.8184058935812,1.66959759189759,-0.456769332935423));
#62623=CARTESIAN_POINT('Ctrl Pts',(-30.7388622663641,1.28693800357811,1.15757717553815));
#62624=CARTESIAN_POINT('Ctrl Pts',(-30.659318639147,-0.278005442596269,
1.70848099675336));
#62625=CARTESIAN_POINT('Ctrl Pts',(-30.57977501193,-1.58755092378435,0.689837956894189));
#62626=CARTESIAN_POINT('Ctrl Pts',(-30.5002313847129,-1.43864555070099,
-0.96254523105604));
#62627=CARTESIAN_POINT('Ctrl Pts',(-30.4206877574959,0.0319143286907724,
-1.73065762587657));
#62628=CARTESIAN_POINT('Ctrl Pts',(-30.3411441302788,1.47315516121278,-0.908849939964034));
#62629=CARTESIAN_POINT('Ctrl Pts',(-30.2616005030618,1.56103820775362,0.747899763547134));
#62630=CARTESIAN_POINT('Ctrl Pts',(-30.1820568758447,0.214827094831843,
1.71756911409893));
#62631=CARTESIAN_POINT('Ctrl Pts',(-30.1025132486276,-1.3287413156003,1.1093425343857));
#62632=CARTESIAN_POINT('Ctrl Pts',(-30.0229696214106,-1.65162201276936,
-0.5180145454678));
#62633=CARTESIAN_POINT('Ctrl Pts',(-29.9434259941935,-0.457191044927401,
-1.66948216247395));
#62634=CARTESIAN_POINT('Ctrl Pts',(-29.8638823669764,1.15725206869828,-1.28723035695793));
#62635=CARTESIAN_POINT('Ctrl Pts',(-29.7843387397594,1.70855116412952,0.277573885537073));
#62636=CARTESIAN_POINT('Ctrl Pts',(-29.7047951125423,0.690238937140185,
1.58737662576847));
#62637=CARTESIAN_POINT('Ctrl Pts',(-29.6252514853252,-0.962181810364402,
1.43888863578262));
#62638=CARTESIAN_POINT('Ctrl Pts',(-29.5457078581082,-1.73066563196221,
-0.0314771778488288));
#62639=CARTESIAN_POINT('Ctrl Pts',(-29.4661642308911,-0.909222017798363,
-1.47292554622804));
#62640=CARTESIAN_POINT('Ctrl Pts',(-29.3866206036741,0.747505434328563,
-1.5612270712583));
#62641=CARTESIAN_POINT('Ctrl Pts',(-29.307076976457,1.71751479575623,-0.215260931752423));
#62642=CARTESIAN_POINT('Ctrl Pts',(-29.2275333492399,1.10967812807928,1.32846106244894));
#62643=CARTESIAN_POINT('Ctrl Pts',(-29.1479897220229,-0.517597342861786,
1.65175280627669));
#62644=CARTESIAN_POINT('Ctrl Pts',(-29.0684460948058,-1.66936662653302,
0.457612727749417));
#62645=CARTESIAN_POINT('Ctrl Pts',(-28.9889024675888,-1.28752262820913,
-1.15692688802273));
#62646=CARTESIAN_POINT('Ctrl Pts',(-28.9093588403717,0.277142310767931,
-1.7086212224957));
#62647=CARTESIAN_POINT('Ctrl Pts',(-28.8298152131547,1.58720222647384,-0.69063987334716));
#62648=CARTESIAN_POINT('Ctrl Pts',(-28.7502715859376,1.43913162905944,0.961818328283063));
#62649=CARTESIAN_POINT('Ctrl Pts',(-28.6707279587206,-0.0310400249985448,
1.73067352762691));
#62650=CARTESIAN_POINT('Ctrl Pts',(-28.5911843315035,-1.47269583726682,
0.909594037621987));
#62651=CARTESIAN_POINT('Ctrl Pts',(-28.5116407042864,-1.56141583515265,
-0.747111057417198));
#62652=CARTESIAN_POINT('Ctrl Pts',(-28.4320970770693,-0.215694754938821,
-1.71746036783163));
#62653=CARTESIAN_POINT('Ctrl Pts',(-28.3525534498523,1.32818072453831,-1.11001365097253));
#62654=CARTESIAN_POINT('Ctrl Pts',(-28.2730098226352,1.65188349439792,0.517180107231717));
#62655=CARTESIAN_POINT('Ctrl Pts',(-28.1934661954182,0.45803438137456,1.66925098408218));
#62656=CARTESIAN_POINT('Ctrl Pts',(-28.1139225682011,-1.15660163353224,
1.28781481731305));
#62657=CARTESIAN_POINT('Ctrl Pts',(-28.0343789409841,-1.70869117184742,
-0.276710718316393));
#62658=CARTESIAN_POINT('Ctrl Pts',(-27.954835313767,-0.691040765489525,
-1.5870277259116));
#62659=CARTESIAN_POINT('Ctrl Pts',(-27.87529168655,0.961454784835226,-1.43937453051593));
#62660=CARTESIAN_POINT('Ctrl Pts',(-27.7957480593328,1.73068131287016,0.0306028701678309));
#62661=CARTESIAN_POINT('Ctrl Pts',(-27.7162044321159,0.909965999411154,
1.4724660343438));
#62662=CARTESIAN_POINT('Ctrl Pts',(-27.6366608048987,-0.746716632838211,
1.56160449942463));
#62663=CARTESIAN_POINT('Ctrl Pts',(-27.5571171776817,-1.71740583032862,
0.216128564363326));
#62664=CARTESIAN_POINT('Ctrl Pts',(-27.4775735504647,-1.11034910304403,
-1.32790030188634));
#62665=CARTESIAN_POINT('Ctrl Pts',(-27.3980299232476,0.516762838604242,
-1.6520140771247));
#62666=CARTESIAN_POINT('Ctrl Pts',(-27.3184862960305,1.66913523512881,-0.458456005775898));
#62667=CARTESIAN_POINT('Ctrl Pts',(-27.2389426688135,1.28810692425103,1.1562763052476));
#62668=CARTESIAN_POINT('Ctrl Pts',(-27.1593990415964,-0.276279108210019,
1.70876101218022));
#62669=CARTESIAN_POINT('Ctrl Pts',(-27.0798554143793,-1.58685312409289,
0.691441613541677));
#62670=CARTESIAN_POINT('Ctrl Pts',(-27.0003117871623,-1.43961734013658,
-0.961091180044105));
#62671=CARTESIAN_POINT('Ctrl Pts',(-26.9207681599452,0.0301657133845961,
-1.73068898769146));
#62672=CARTESIAN_POINT('Ctrl Pts',(-26.8412245327282,1.47223613747364,-0.910337903142115));
#62673=CARTESIAN_POINT('Ctrl Pts',(-26.7616809055111,1.56179306406219,0.746322160616793));
#62674=CARTESIAN_POINT('Ctrl Pts',(-26.6821372782941,0.216562359998259,
1.71735118325067));
#62675=CARTESIAN_POINT('Ctrl Pts',(-26.602593651077,-1.32761979451087,1.11068448427239));
#62676=CARTESIAN_POINT('Ctrl Pts',(-26.52305002386,-1.65214455444872,-0.516345537005934));
#62677=CARTESIAN_POINT('Ctrl Pts',(-26.4435063966428,-0.458877600926578,
-1.66901937968028));
#62678=CARTESIAN_POINT('Ctrl Pts',(-26.3639627694258,1.15595090318951,-1.28839894900448));
#62679=CARTESIAN_POINT('Ctrl Pts',(-26.2844191422087,1.70883074348965,0.275847480476298));
#62680=CARTESIAN_POINT('Ctrl Pts',(-26.2048755149917,0.691842417478086,
1.58667842102884));
#62681=CARTESIAN_POINT('Ctrl Pts',(-26.1253318877746,-0.960727513932856,
1.43986005790594));
#62682=CARTESIAN_POINT('Ctrl Pts',(-26.0457882605576,-1.73069655209032,
-0.0297285546766869));
#62683=CARTESIAN_POINT('Ctrl Pts',(-25.9662446333405,-0.910709748791179,
-1.472006146671));
#62684=CARTESIAN_POINT('Ctrl Pts',(-25.8867010061235,0.745927640778065,
-1.56198152905332));
#62685=CARTESIAN_POINT('Ctrl Pts',(-25.8071573789064,1.71729642660127,-0.21699614181597));
#62686=CARTESIAN_POINT('Ctrl Pts',(-25.7276137516893,1.1110197946362,1.32733920242982));
#62687=CARTESIAN_POINT('Ctrl Pts',(-25.6480701244723,-0.515928202463446,
1.65227492636163));
#62688=CARTESIAN_POINT('Ctrl Pts',(-25.5685264972552,-1.668903417744,0.459299166799682));
#62689=CARTESIAN_POINT('Ctrl Pts',(-25.4889828700381,-1.28869089155473,
-1.15562542737878));
#62690=CARTESIAN_POINT('Ctrl Pts',(-25.4094392428211,0.275415835142812,
-1.70890036577125));
#62691=CARTESIAN_POINT('Ctrl Pts',(-25.329895615604,1.5865036167306,-0.692243177273134));
#62692=CARTESIAN_POINT('Ctrl Pts',(-25.250351988387,1.44010268380848,0.960363786524726));
#62693=CARTESIAN_POINT('Ctrl Pts',(-25.1708083611699,-0.0292913940720509,
1.73070400606627));
#62694=CARTESIAN_POINT('Ctrl Pts',(-25.0912647339529,-1.47177606195057,
0.911081536334578));
#62695=CARTESIAN_POINT('Ctrl Pts',(-25.0117211067358,-1.56216989438597,
-0.745533073347261));
#62696=CARTESIAN_POINT('Ctrl Pts',(-24.9321774795187,-0.217429909788733,
-1.71724156038391));
#62697=CARTESIAN_POINT('Ctrl Pts',(-24.8526338523017,1.32705852566112,-1.11135503411405));
#62698=CARTESIAN_POINT('Ctrl Pts',(-24.7730902250846,1.65240519285512,0.515510835003435));
#62699=CARTESIAN_POINT('Ctrl Pts',(-24.6935465978676,0.45972070336827,1.66878734932737));
#62700=CARTESIAN_POINT('Ctrl Pts',(-24.6140029706505,-1.15529987783615,
1.28898275188315));
#62701=CARTESIAN_POINT('Ctrl Pts',(-24.5344593434335,-1.70896987902057,
-0.274984172237085));
#62702=CARTESIAN_POINT('Ctrl Pts',(-24.4549157162164,-0.692643892901292,
-1.58632871120933));
#62703=CARTESIAN_POINT('Ctrl Pts',(-24.3753720889993,0.959999997842893,
-1.44034521782875));
#62704=CARTESIAN_POINT('Ctrl Pts',(-24.2958284617823,1.73071134961881,0.028854231598518));
#62705=CARTESIAN_POINT('Ctrl Pts',(-24.2162848345652,0.91145326574864,1.471545883327));
#62706=CARTESIAN_POINT('Ctrl Pts',(-24.1367412073482,-0.745138458349476,
1.56235816004816));
#62707=CARTESIAN_POINT('Ctrl Pts',(-24.0571975801311,-1.71718658460209,
0.217863663888931));
#62708=CARTESIAN_POINT('Ctrl Pts',(-23.977653952914,-1.1116902026846,-1.32677776422261));
#62709=CARTESIAN_POINT('Ctrl Pts',(-23.8981103256969,0.515093434652472,
-1.65253535392088));
#62710=CARTESIAN_POINT('Ctrl Pts',(-23.8185666984799,1.66867117443778,-0.460142210605531));
#62711=CARTESIAN_POINT('Ctrl Pts',(-23.7390230712628,1.28927452997115,1.1549742545824));
#62712=CARTESIAN_POINT('Ctrl Pts',(-23.6594794440458,-0.27455249178663,
1.7090392832332));
#62713=CARTESIAN_POINT('Ctrl Pts',(-23.5799358168287,-1.58615370447617,
0.693044564336977));
#62714=CARTESIAN_POINT('Ctrl Pts',(-23.5003921896117,-1.44058765995127,
-0.959636147910556));
#62715=CARTESIAN_POINT('Ctrl Pts',(-23.4208485623946,0.0284170672840143,
-1.73071858274749));
#62716=CARTESIAN_POINT('Ctrl Pts',(-23.3413049351776,1.47131561081499,-0.91182493700963));
#62717=CARTESIAN_POINT('Ctrl Pts',(-23.2617613079605,1.56254632602784,0.744743795809934));
#62718=CARTESIAN_POINT('Ctrl Pts',(-23.1822176807434,0.218297404088875,
1.71713149925932));
#62719=CARTESIAN_POINT('Ctrl Pts',(-23.1026740535264,-1.32649691813226,
1.11202530032643));
#62720=CARTESIAN_POINT('Ctrl Pts',(-23.0231304263093,-1.65266540955062,
-0.514676001437202));
#62721=CARTESIAN_POINT('Ctrl Pts',(-22.9435867990922,-0.460563688484515,
-1.66855489308264));
#62722=CARTESIAN_POINT('Ctrl Pts',(-22.8640431718752,1.15464855763828,-1.28956622580011));
#62723=CARTESIAN_POINT('Ctrl Pts',(-22.7844995446581,1.7091085784047,0.274120793819028));
#62724=CARTESIAN_POINT('Ctrl Pts',(-22.7049559174411,0.693445191554635,
1.58597859654229));
#62725=CARTESIAN_POINT('Ctrl Pts',(-22.625412290224,-0.959272236750958,
1.44083001016057));
#62726=CARTESIAN_POINT('Ctrl Pts',(-22.5458686630069,-1.73072570545184,
-0.0279799011564179));
#62727=CARTESIAN_POINT('Ctrl Pts',(-22.4663250357899,-0.912196550093822,
-1.47108524442924));
#62728=CARTESIAN_POINT('Ctrl Pts',(-22.3867814085729,0.74434908575382,-1.56273439231303));
#62729=CARTESIAN_POINT('Ctrl Pts',(-22.3072377813557,1.71707630435912,-0.218731130360849));
#62730=CARTESIAN_POINT('Ctrl Pts',(-22.2276941541387,1.11236032701816,1.32621598740799));
#62731=CARTESIAN_POINT('Ctrl Pts',(-22.1481505269216,-0.5142585353843,1.65279535973601));
#62732=CARTESIAN_POINT('Ctrl Pts',(-22.0686068997046,-1.66843850526939,
0.460985136978328));
#62733=CARTESIAN_POINT('Ctrl Pts',(-21.9890632724875,-1.28985783935138,
-1.15432278702462));
#62734=CARTESIAN_POINT('Ctrl Pts',(-21.9095196452705,0.273689078361827,
-1.70917776453064));
#62735=CARTESIAN_POINT('Ctrl Pts',(-21.8299760180534,1.58580338741888,-0.693845774528669));
#62736=CARTESIAN_POINT('Ctrl Pts',(-21.7504323908364,1.44107226844117,0.958908264387324));
#62737=CARTESIAN_POINT('Ctrl Pts',(-21.6708887636193,-0.0275427332436607,
1.73073271773141));
#62738=CARTESIAN_POINT('Ctrl Pts',(-21.5913451364023,-1.47085478418445,
0.912568104977495));
#62739=CARTESIAN_POINT('Ctrl Pts',(-21.5118015091852,-1.5629223588917,-0.7439543282063));
#62740=CARTESIAN_POINT('Ctrl Pts',(-21.4322578819681,-0.219164842677231,
-1.717020999905));
#62741=CARTESIAN_POINT('Ctrl Pts',(-21.352714254751,1.32593497206768,-1.11269528273844));
#62742=CARTESIAN_POINT('Ctrl Pts',(-21.273170627534,1.65292520446879,0.513841036520355));
#62743=CARTESIAN_POINT('Ctrl Pts',(-21.1936270003169,0.461406556060124,
1.66832201100544));
#62744=CARTESIAN_POINT('Ctrl Pts',(-21.1140833730999,-1.15399694276216,
1.29014937060639));
#62745=CARTESIAN_POINT('Ctrl Pts',(-21.0345397458828,-1.70924684160662,
-0.273257345442523));
#62746=CARTESIAN_POINT('Ctrl Pts',(-20.9549961186657,-0.694246313233563,
-1.58562807711711));
#62747=CARTESIAN_POINT('Ctrl Pts',(-20.8754524914487,0.958544230842836,
-1.44131443477765));
#62748=CARTESIAN_POINT('Ctrl Pts',(-20.7959088642316,1.73073961958576,0.0271055635735854));
#62749=CARTESIAN_POINT('Ctrl Pts',(-20.7163652370146,0.912939601636987,
1.4706242300953));
#62750=CARTESIAN_POINT('Ctrl Pts',(-20.6368216097975,-0.743559523192568,
1.56311022575189));
#62751=CARTESIAN_POINT('Ctrl Pts',(-20.5572779825805,-1.71696558590049,
0.219598541010339));
#62752=CARTESIAN_POINT('Ctrl Pts',(-20.4777343553634,-1.11303016746587,
-1.3256538721293));
#62753=CARTESIAN_POINT('Ctrl Pts',(-20.3981907281463,0.513423504872026,
-1.65305494374066));
#62754=CARTESIAN_POINT('Ctrl Pts',(-20.3186471009293,1.66820541029823,-0.461827945702956));
#62755=CARTESIAN_POINT('Ctrl Pts',(-20.2391034737122,1.29044081954653,1.15367102487173));
#62756=CARTESIAN_POINT('Ctrl Pts',(-20.1595598464952,-0.272825595088725,
1.70931580962822));
#62757=CARTESIAN_POINT('Ctrl Pts',(-20.0800162192781,-1.58545266564817,
0.694646807643726));
#62758=CARTESIAN_POINT('Ctrl Pts',(-20.0004725920611,-1.44155650915452,
-0.958180136140769));
#62759=CARTESIAN_POINT('Ctrl Pts',(-19.9209289648439,0.0266683921741259,
-1.73074641101443));
#62760=CARTESIAN_POINT('Ctrl Pts',(-19.841385337627,1.47039358217654,-0.913311040048543));
#62761=CARTESIAN_POINT('Ctrl Pts',(-19.7618417104098,1.5632979928816,0.743164670737831));
#62762=CARTESIAN_POINT('Ctrl Pts',(-19.6822980831928,0.220032225332462,
1.71691006234914));
#62763=CARTESIAN_POINT('Ctrl Pts',(-19.6027544559757,-1.32537268761077,
1.11336498117908));
#62764=CARTESIAN_POINT('Ctrl Pts',(-19.5232108287587,-1.65318457754334,
-0.513005940465945));
#62765=CARTESIAN_POINT('Ctrl Pts',(-19.4436672015416,-0.462249305879991,
-1.66808870315519));
#62766=CARTESIAN_POINT('Ctrl Pts',(-19.3641235743246,1.15334503337407,-1.29073218615321));
#62767=CARTESIAN_POINT('Ctrl Pts',(-19.2845799471075,1.70938466859105,0.272393827327927));
#62768=CARTESIAN_POINT('Ctrl Pts',(-19.2050363198905,0.695047257733653,
1.58527715302323));
#62769=CARTESIAN_POINT('Ctrl Pts',(-19.1254926926734,-0.957815980304312,
1.44179849155635));
#62770=CARTESIAN_POINT('Ctrl Pts',(-19.0459490654563,-1.73075309201701,
-0.0262312190731219));
#62771=CARTESIAN_POINT('Ctrl Pts',(-18.9664054382393,-0.913682420188505,
-1.47016284044285));
#62772=CARTESIAN_POINT('Ctrl Pts',(-18.8868618110222,0.742769770867235,
-1.56348566026885));
#62773=CARTESIAN_POINT('Ctrl Pts',(-18.8073181838051,1.71685442925448,-0.220465895615978));
#62774=CARTESIAN_POINT('Ctrl Pts',(-18.7277745565881,1.11369972385674,1.32509141853002));
#62775=CARTESIAN_POINT('Ctrl Pts',(-18.648230929371,-0.512588343328754,
1.65331410586857));
#62776=CARTESIAN_POINT('Ctrl Pts',(-18.568687302154,-1.66797188958377,0.462670636564333));
#62777=CARTESIAN_POINT('Ctrl Pts',(-18.4891436749369,-1.29102347040784,
-1.15301896829003));
#62778=CARTESIAN_POINT('Ctrl Pts',(-18.4096000477198,0.271962042187704,
-1.70945341849072));
#62779=CARTESIAN_POINT('Ctrl Pts',(-18.3300564205028,1.58510153925351,-0.695447663477738));
#62780=CARTESIAN_POINT('Ctrl Pts',(-18.2505127932857,1.44204038196771,0.957451763356733));
#62781=CARTESIAN_POINT('Ctrl Pts',(-18.1709691660687,-0.0257940442985307,
1.73075966259305));
#62782=CARTESIAN_POINT('Ctrl Pts',(-18.0914255388516,-1.46993200490897,
0.914053742033148));
#62783=CARTESIAN_POINT('Ctrl Pts',(-18.0118819116345,-1.56367322790166,
-0.742374823606033));
#62784=CARTESIAN_POINT('Ctrl Pts',(-17.9323382844175,-0.220899551833179,
-1.71679868662007));
#62785=CARTESIAN_POINT('Ctrl Pts',(-17.8527946572004,1.32481006490503,-1.11403439547746));
#62786=CARTESIAN_POINT('Ctrl Pts',(-17.7732510299834,1.65344352870807,0.51217071348712));
#62787=CARTESIAN_POINT('Ctrl Pts',(-17.6937074027663,0.46309193772906,1.66785496959143));
#62788=CARTESIAN_POINT('Ctrl Pts',(-17.6141637755492,-1.1526928296404,1.29131467229181));
#62789=CARTESIAN_POINT('Ctrl Pts',(-17.5346201483322,-1.70952205932282,
-0.271530239695595));
#62790=CARTESIAN_POINT('Ctrl Pts',(-17.4550765211151,-0.695848024850479,
-1.58492582435021));
#62791=CARTESIAN_POINT('Ctrl Pts',(-17.3755328938981,0.957087485321226,
-1.44228218037317));
#62792=CARTESIAN_POINT('Ctrl Pts',(-17.295989266681,1.73076612274215,0.025356867878193));
#62793=CARTESIAN_POINT('Ctrl Pts',(-17.216445639464,0.914425005558822,1.46970107558961));
#62794=CARTESIAN_POINT('Ctrl Pts',(-17.1369020122469,-0.741979828979377,
1.56386069576808));
#62795=CARTESIAN_POINT('Ctrl Pts',(-17.0573583850298,-1.71674283444945,
0.221333193956447));
#62796=CARTESIAN_POINT('Ctrl Pts',(-16.9778147578128,-1.11436899601991,
-1.32452862675371));
#62797=CARTESIAN_POINT('Ctrl Pts',(-16.8982711305957,0.511753050967637,
-1.6535728460536));
#62798=CARTESIAN_POINT('Ctrl Pts',(-16.8187275033786,1.66773794318562,-0.463513209347343));
#62799=CARTESIAN_POINT('Ctrl Pts',(-16.7391838761616,1.29160579178658,1.15236661744596));
#62800=CARTESIAN_POINT('Ctrl Pts',(-16.6596402489446,-0.271098419879153,
1.709590591083));
#62801=CARTESIAN_POINT('Ctrl Pts',(-16.5800966217275,-1.58475000832453,
0.696248341826323));
#62802=CARTESIAN_POINT('Ctrl Pts',(-16.5005529945104,-1.44252388675729,
-0.956723146221068));
#62803=CARTESIAN_POINT('Ctrl Pts',(-16.4210093672934,0.0249196898400101,
-1.73077247246389));
#62804=CARTESIAN_POINT('Ctrl Pts',(-16.3414657400763,1.46947005249952,-0.914796210741802));
#62805=CARTESIAN_POINT('Ctrl Pts',(-16.2619221128592,1.56404806385614,0.741584787012495));
#62806=CARTESIAN_POINT('Ctrl Pts',(-16.1823784856422,0.221766821958055,
1.7166868727462));
#62807=CARTESIAN_POINT('Ctrl Pts',(-16.1028348584251,-1.32424710409405,
1.11470352546272));
#62808=CARTESIAN_POINT('Ctrl Pts',(-16.0232912312081,-1.6537020578969,-0.511335355797014));
#62809=CARTESIAN_POINT('Ctrl Pts',(-15.943747603991,-0.463934451392264,
-1.66762081037383));
#62810=CARTESIAN_POINT('Ctrl Pts',(-15.8642039767739,1.15204033172758,-1.29189682887354));
#62811=CARTESIAN_POINT('Ctrl Pts',(-15.7846603495569,1.70965901376687,0.270666582765945));
#62812=CARTESIAN_POINT('Ctrl Pts',(-15.7051167223398,0.696648614379695,
1.58457409118771));
#62813=CARTESIAN_POINT('Ctrl Pts',(-15.6255730951228,-0.956358746079515,
1.44276550110464));
#62814=CARTESIAN_POINT('Ctrl Pts',(-15.5460294679057,-1.73077871175787,
-0.0244825102119152));
#62815=CARTESIAN_POINT('Ctrl Pts',(-15.4664858406887,-0.915167357558401,
-1.46923893565345));
#62816=CARTESIAN_POINT('Ctrl Pts',(-15.3869422134716,0.741189697730577,
-1.56423533215388));
#62817=CARTESIAN_POINT('Ctrl Pts',(-15.3073985862545,1.71663080151387,-0.222200435810386));
#62818=CARTESIAN_POINT('Ctrl Pts',(-15.2278549590375,1.11503798378458,1.32396549694398));
#62819=CARTESIAN_POINT('Ctrl Pts',(-15.1483113318204,-0.510917628001855,
1.65383116422973));
#62820=CARTESIAN_POINT('Ctrl Pts',(-15.0687677046033,-1.66750357116349,
0.464355663836996));
#62821=CARTESIAN_POINT('Ctrl Pts',(-14.9892240773863,-1.29218778353415,
-1.15171397250602));
#62822=CARTESIAN_POINT('Ctrl Pts',(-14.9096804501692,0.270234728383482,
-1.70972732737007));
#62823=CARTESIAN_POINT('Ctrl Pts',(-14.8301368229522,1.58439807295096,-0.697048842485089));
#62824=CARTESIAN_POINT('Ctrl Pts',(-14.7505931957351,1.44300702339981,0.955994284919805));
#62825=CARTESIAN_POINT('Ctrl Pts',(-14.671049568518,-0.0240453290217912,
1.73078484062367));
#62826=CARTESIAN_POINT('Ctrl Pts',(-14.591505941301,-1.46900772506611,0.91553844598496));
#62827=CARTESIAN_POINT('Ctrl Pts',(-14.5119623140839,-1.56442250064936,
-0.740794561158851));
#62828=CARTESIAN_POINT('Ctrl Pts',(-14.4324186868669,-0.222634035485727,
-1.71657462075608));
#62829=CARTESIAN_POINT('Ctrl Pts',(-14.3528750596498,1.3236838053215,-1.11537237096409));
#62830=CARTESIAN_POINT('Ctrl Pts',(-14.2733314324328,1.65396016504384,0.510499867608859));
#62831=CARTESIAN_POINT('Ctrl Pts',(-14.1937878052157,0.46477684665457,1.66738622556214));
#62832=CARTESIAN_POINT('Ctrl Pts',(-14.1142441779986,-1.15138753980216,
1.29247865574979));
#62833=CARTESIAN_POINT('Ctrl Pts',(-14.0347005507816,-1.70979553188824,
-0.269802856759417));
#62834=CARTESIAN_POINT('Ctrl Pts',(-13.9551569235645,-0.697449026116917,
-1.58422195362553));
#62835=CARTESIAN_POINT('Ctrl Pts',(-13.8756132963474,0.955629762765192,
-1.44324845362737));
#62836=CARTESIAN_POINT('Ctrl Pts',(-13.7960696691304,1.73079085906093,0.0236081462974931));
#62837=CARTESIAN_POINT('Ctrl Pts',(-13.7165260419133,0.915909475997773,
1.46877642075232));
#62838=CARTESIAN_POINT('Ctrl Pts',(-13.6369824146963,-0.740399377322555,
1.5646095693306));
#62839=CARTESIAN_POINT('Ctrl Pts',(-13.5574387874792,-1.71651833047635,
0.223067620956417));
#62840=CARTESIAN_POINT('Ctrl Pts',(-13.4778951602621,-1.11570668697998,
-1.32340202924457));
#62841=CARTESIAN_POINT('Ctrl Pts',(-13.3983515330451,0.510082074644636,
-1.65408906033102));
#62842=CARTESIAN_POINT('Ctrl Pts',(-13.318807905828,1.66726877357721,-0.465197999818213));
#62843=CARTESIAN_POINT('Ctrl Pts',(-13.239264278611,1.29276944550198,1.15106103363678));
#62844=CARTESIAN_POINT('Ctrl Pts',(-13.1597206513939,-0.269370967921155,
1.70986362731701));
#62845=CARTESIAN_POINT('Ctrl Pts',(-13.0801770241769,-1.5840457332226,0.697849165249764));
#62846=CARTESIAN_POINT('Ctrl Pts',(-13.0006333969598,-1.44348979177201,
-0.955265179638894));
#62847=CARTESIAN_POINT('Ctrl Pts',(-12.9210897697427,0.023170962066939,
-1.73079676706925));
#62848=CARTESIAN_POINT('Ctrl Pts',(-12.8415461425257,1.46854502272674,-0.916280447573221));
#62849=CARTESIAN_POINT('Ctrl Pts',(-12.7620025153086,1.56479653818574,0.740004146246785));
#62850=CARTESIAN_POINT('Ctrl Pts',(-12.6824588880916,0.223501192194875,
1.71646193067834));
#62851=CARTESIAN_POINT('Ctrl Pts',(-12.6029152608745,-1.32312016873115,
1.11604093181088));
#62852=CARTESIAN_POINT('Ctrl Pts',(-12.5233716336574,-1.65421785008302,
-0.509664249135823));
#62853=CARTESIAN_POINT('Ctrl Pts',(-12.4438280064404,-0.465619123301057,
-1.66715121521621));
#62854=CARTESIAN_POINT('Ctrl Pts',(-12.3642843792233,1.15073445403071,-1.29306015277216));
#62855=CARTESIAN_POINT('Ctrl Pts',(-12.2847407520063,1.70993161365207,0.26893906189636));
#62856=CARTESIAN_POINT('Ctrl Pts',(-12.2051971247892,0.698249259857993,
1.58386941175347));
#62857=CARTESIAN_POINT('Ctrl Pts',(-12.1256534975721,-0.954900535564221,
1.44373103781822));
#62858=CARTESIAN_POINT('Ctrl Pts',(-12.0461098703551,-1.73080256464825,
-0.0227337763580157));
#62859=CARTESIAN_POINT('Ctrl Pts',(-11.966566243138,-0.91665136068759,-1.46831353100421));
#62860=CARTESIAN_POINT('Ctrl Pts',(-11.8870226159209,0.739608867956876,
-1.5649834072028));
#62861=CARTESIAN_POINT('Ctrl Pts',(-11.8074789887039,1.71640542136559,-0.223934749173347));
#62862=CARTESIAN_POINT('Ctrl Pts',(-11.7279353614868,1.11637510543549,1.32283822379925));
#62863=CARTESIAN_POINT('Ctrl Pts',(-11.6483917342698,-0.509246391109146,
1.65434653429165));
#62864=CARTESIAN_POINT('Ctrl Pts',(-11.5688481070527,-1.66703355048665,
0.466040217076157));
#62865=CARTESIAN_POINT('Ctrl Pts',(-11.4893044798357,-1.29335077754172,
-1.15040780100482));
#62866=CARTESIAN_POINT('Ctrl Pts',(-11.4097608526186,0.268507138712558,
-1.70999949088906));
#62867=CARTESIAN_POINT('Ctrl Pts',(-11.3302172254015,1.58369298922935,-0.698649309916132));
#62868=CARTESIAN_POINT('Ctrl Pts',(-11.2506735981845,1.44397219175068,0.954535830564389));
#62869=CARTESIAN_POINT('Ctrl Pts',(-11.1711299709674,-0.0222965891985885,
1.73080825179759));
#62870=CARTESIAN_POINT('Ctrl Pts',(-11.0915863437504,-1.46808194559948,
0.917022215317227));
#62871=CARTESIAN_POINT('Ctrl Pts',(-11.0120427165333,-1.56517017636985,
-0.73921354247797));
#62872=CARTESIAN_POINT('Ctrl Pts',(-10.9324990893162,-0.224368291864247,
-1.71634880254173));
#62873=CARTESIAN_POINT('Ctrl Pts',(-10.8529554620992,1.32255619446684,-1.11670920783251));
#62874=CARTESIAN_POINT('Ctrl Pts',(-10.7734118348821,1.65447511294868,0.508828500591231));
#62875=CARTESIAN_POINT('Ctrl Pts',(-10.6938682076651,0.46646128111671,1.66691577939602));
#62876=CARTESIAN_POINT('Ctrl Pts',(-10.614324580448,-1.1500810745799,1.29364131979218));
#62877=CARTESIAN_POINT('Ctrl Pts',(-10.5347809532309,-1.71006725902369,
-0.268075198397277));
#62878=CARTESIAN_POINT('Ctrl Pts',(-10.4552373260139,-0.699049315398613,
-1.58351646566153));
#62879=CARTESIAN_POINT('Ctrl Pts',(-10.3756936987968,0.954171064662698,
-1.44421325355396));
#62880=CARTESIAN_POINT('Ctrl Pts',(-10.2961500715798,1.73081382851686,0.0218594006165701));
#62881=CARTESIAN_POINT('Ctrl Pts',(-10.2166064443627,0.917393011438508,
1.46785026652732));
#62882=CARTESIAN_POINT('Ctrl Pts',(-10.1370628171456,-0.738818169835363,
1.565356845675));
#62883=CARTESIAN_POINT('Ctrl Pts',(-10.0575191899286,-1.71629207421038,
0.224801820239825));
#62884=CARTESIAN_POINT('Ctrl Pts',(-9.97797556271151,-1.11704323898056,
-1.32227408075192));
#62885=CARTESIAN_POINT('Ctrl Pts',(-9.89843193549448,0.50841057760874,-1.65460358604592));
#62886=CARTESIAN_POINT('Ctrl Pts',(-9.81888830827739,1.66679790195186,-0.466882315395799));
#62887=CARTESIAN_POINT('Ctrl Pts',(-9.73934468106036,1.29393177950496,1.14975427477686));
#62888=CARTESIAN_POINT('Ctrl Pts',(-9.65980105384328,-0.26764324097813,
1.71013491805157));
#62889=CARTESIAN_POINT('Ctrl Pts',(-9.58025742662623,-1.58333984106127,
0.699449276279938));
#62890=CARTESIAN_POINT('Ctrl Pts',(-9.50071379940916,-1.44445422321269,
-0.953806237882455));
#62891=CARTESIAN_POINT('Ctrl Pts',(-9.42117017219211,0.0214222106399076,
-1.73081929480574));
#62892=CARTESIAN_POINT('Ctrl Pts',(-9.34162654497504,1.4676184938025,-0.917763749027703));
#62893=CARTESIAN_POINT('Ctrl Pts',(-9.26208291775799,1.56554341510633,0.73842275005424));
#62894=CARTESIAN_POINT('Ctrl Pts',(-9.18253929054093,0.22523533427249,1.71623523637514));
#62895=CARTESIAN_POINT('Ctrl Pts',(-9.10299566332387,-1.32199188267247,
1.11737719885839));
#62896=CARTESIAN_POINT('Ctrl Pts',(-9.02345203610681,-1.65473195357519,
-0.507992622188313));
#62897=CARTESIAN_POINT('Ctrl Pts',(-8.94390840888974,-0.467303319886586,
-1.66667991816168));
#62898=CARTESIAN_POINT('Ctrl Pts',(-8.86436478167269,1.14942740161649,-1.29422215666154));
#62899=CARTESIAN_POINT('Ctrl Pts',(-8.78482115445563,1.71020246796842,0.267211266482613));
#62900=CARTESIAN_POINT('Ctrl Pts',(-8.70527752723857,0.699849192534625,
1.58316311543983));
#62901=CARTESIAN_POINT('Ctrl Pts',(-8.62573390002151,-0.953441350246909,
1.4446951007115));
#62902=CARTESIAN_POINT('Ctrl Pts',(-8.54619027280445,-1.73082465066384,
-0.0209850192964212));
#62903=CARTESIAN_POINT('Ctrl Pts',(-8.46664664558739,-0.918134428061233,
-1.46738662743981));
#62904=CARTESIAN_POINT('Ctrl Pts',(-8.38710301837034,0.738027283159815,
-1.56572988465197));
#62905=CARTESIAN_POINT('Ctrl Pts',(-8.30755939115327,1.71617828903966,-0.225668833934531));
#62906=CARTESIAN_POINT('Ctrl Pts',(-8.22801576393622,1.11771108744463,1.32170960024654));
#62907=CARTESIAN_POINT('Ctrl Pts',(-8.14847213671915,-0.507574634356665,
1.65486021552826));
#62908=CARTESIAN_POINT('Ctrl Pts',(-8.06892850950209,-1.66656182803301,
0.467724294562213));
#62909=CARTESIAN_POINT('Ctrl Pts',(-7.98938488228503,-1.29451245124338,
-1.1491004551197));
#62910=CARTESIAN_POINT('Ctrl Pts',(-7.90984125506798,0.266779274938363,
-1.71026990876992));
#62911=CARTESIAN_POINT('Ctrl Pts',(-7.83029762785091,1.58298628880849,-0.700249064137086));
#62912=CARTESIAN_POINT('Ctrl Pts',(-7.75075400063385,1.44493588603502,0.953076401779334));
#62913=CARTESIAN_POINT('Ctrl Pts',(-7.6712103734168,-0.020547826614065,
1.73082989609086));
#62914=CARTESIAN_POINT('Ctrl Pts',(-7.59166674619973,-1.46715466745408,
0.918505048515373));
#62915=CARTESIAN_POINT('Ctrl Pts',(-7.51212311898269,-1.56591625429995,
-0.737631769177359));
#62916=CARTESIAN_POINT('Ctrl Pts',(-7.4325794917656,-0.226102319198319,
-1.71612123220756));
#62917=CARTESIAN_POINT('Ctrl Pts',(-7.35303586454856,1.32142723349209,-1.11804490471801));
#62918=CARTESIAN_POINT('Ctrl Pts',(-7.27349223733149,1.65498837189696,0.507156614140401));
#62919=CARTESIAN_POINT('Ctrl Pts',(-7.19394861011444,0.468145239395855,
1.6664436315734));
#62920=CARTESIAN_POINT('Ctrl Pts',(-7.11440498289737,-1.14877343530734,
1.29480266323198));
#62921=CARTESIAN_POINT('Ctrl Pts',(-7.03486135568031,-1.71033724045177,
-0.266347266372873));
#62922=CARTESIAN_POINT('Ctrl Pts',(-6.95531772846326,-0.700648891061883,
-1.5828093611785));
#62923=CARTESIAN_POINT('Ctrl Pts',(-6.87577410124619,0.952711392503003,
-1.44517657916793));
#62924=CARTESIAN_POINT('Ctrl Pts',(-6.79623047402915,1.73083503108646,0.0201106326207077));
#62925=CARTESIAN_POINT('Ctrl Pts',(-6.71668684681207,0.918875610366531,
1.46692261386005));
#62926=CARTESIAN_POINT('Ctrl Pts',(-6.63714321959502,-0.737236208132049,
1.56610252403845));
#62927=CARTESIAN_POINT('Ctrl Pts',(-6.55759959237796,-1.7160640658825,0.226535790036225));
#62928=CARTESIAN_POINT('Ctrl Pts',(-6.47805596516089,-1.11837865065723,
-1.32114478242718));
#62929=CARTESIAN_POINT('Ctrl Pts',(-6.39851233794384,0.506738561566241,
-1.65511642267311));
#62930=CARTESIAN_POINT('Ctrl Pts',(-6.31896871072678,1.66632532879034,-0.468566154360624));
#62931=CARTESIAN_POINT('Ctrl Pts',(-6.23942508350972,1.29509279260886,1.14844634220024));
#62932=CARTESIAN_POINT('Ctrl Pts',(-6.15988145629267,-0.265915240813773,
1.71040446300967));
#62933=CARTESIAN_POINT('Ctrl Pts',(-6.0803378290756,-1.58263233256119,0.70104867328343));
#62934=CARTESIAN_POINT('Ctrl Pts',(-6.00079420185854,-1.44541718009479,
-0.952346322441234));
#62935=CARTESIAN_POINT('Ctrl Pts',(-5.92125057464147,0.0196734373442374,
-1.7308400556503));
#62936=CARTESIAN_POINT('Ctrl Pts',(-5.84170694742443,1.46669046667259,-0.919246113591029));
#62937=CARTESIAN_POINT('Ctrl Pts',(-5.76216332020736,1.56628869385553,0.736840600049199));
#62938=CARTESIAN_POINT('Ctrl Pts',(-5.6826196929903,0.226969246420528,1.7160067900681));
#62939=CARTESIAN_POINT('Ctrl Pts',(-5.60307606577325,-1.32086224706982,
1.118712325241));
#62940=CARTESIAN_POINT('Ctrl Pts',(-5.52353243855618,-1.65524436784856,
-0.506320476660882));
#62941=CARTESIAN_POINT('Ctrl Pts',(-5.44398881133913,-0.468987039429618,
-1.66620691969142));
#62942=CARTESIAN_POINT('Ctrl Pts',(-5.36444518412206,1.1481191758193,-1.29538283935543));
#62943=CARTESIAN_POINT('Ctrl Pts',(-5.284901556905,1.71047157643935,0.265483198288593));
#62944=CARTESIAN_POINT('Ctrl Pts',(-5.20535792968795,0.701448410776275,
1.58245520296781));
#62945=CARTESIAN_POINT('Ctrl Pts',(-5.12581430247088,-0.951981191617268,
1.44565768880032));
#62946=CARTESIAN_POINT('Ctrl Pts',(-5.04627067525383,-1.73084496978208,
-0.019236240812523));
#62947=CARTESIAN_POINT('Ctrl Pts',(-4.96672704803676,-0.919616558165243,
-1.46645822590648));
#62948=CARTESIAN_POINT('Ctrl Pts',(-4.88718342081971,0.736444944953975,
-1.56647476373933));
#62949=CARTESIAN_POINT('Ctrl Pts',(-4.80763979360264,1.71594940476801,-0.227402688323648));
#62950=CARTESIAN_POINT('Ctrl Pts',(-4.7280961663856,1.11904592844805,1.32057962743803));
#62951=CARTESIAN_POINT('Ctrl Pts',(-4.64855253916852,-0.505902359450965,
1.65537220741512));
#62952=CARTESIAN_POINT('Ctrl Pts',(-4.56900891195147,-1.66608840428416,
0.46940789457605));
#62953=CARTESIAN_POINT('Ctrl Pts',(-4.4894652847344,-1.29567280345324,-1.14779193618536));
#62954=CARTESIAN_POINT('Ctrl Pts',(-4.40992165751735,0.265051138824868,
-1.71053858073654));
#62955=CARTESIAN_POINT('Ctrl Pts',(-4.33037803030029,1.58227797240973,-0.701848103514873));
#62956=CARTESIAN_POINT('Ctrl Pts',(-4.25083440308323,1.44589810526913,0.951616000054438));
#62957=CARTESIAN_POINT('Ctrl Pts',(-4.17129077586617,-0.0187990430534725,
1.73084977348145));
#62958=CARTESIAN_POINT('Ctrl Pts',(-4.09174714864911,-1.46622589157654,
0.919986944065575));
#62959=CARTESIAN_POINT('Ctrl Pts',(-4.01220352143205,-1.56666073367799,
-0.736049242871692));
#62960=CARTESIAN_POINT('Ctrl Pts',(-3.93265989421499,-0.227836115717847,
-1.71589190998592));
#62961=CARTESIAN_POINT('Ctrl Pts',(-3.85311626699793,1.32029692354984,-1.11937946025705));
#62962=CARTESIAN_POINT('Ctrl Pts',(-3.77357263978087,1.65549994136465,0.505484209963166));
#62963=CARTESIAN_POINT('Ctrl Pts',(-3.69402901256381,0.469828719773019,
1.66596978257618));
#62964=CARTESIAN_POINT('Ctrl Pts',(-3.61448538534676,-1.14746462331935,
1.29596268488375));
#62965=CARTESIAN_POINT('Ctrl Pts',(-3.53494175812969,-1.71060547589691,
-0.264619062450219));
#62966=CARTESIAN_POINT('Ctrl Pts',(-3.45539813091264,-0.702247751473749,
-1.58210064089821));
#62967=CARTESIAN_POINT('Ctrl Pts',(-3.37585450369557,0.951250747776082,
-1.44613842948588));
#62968=CARTESIAN_POINT('Ctrl Pts',(-3.29631087647852,1.73085446674812,0.0183618440950245));
#62969=CARTESIAN_POINT('Ctrl Pts',(-3.21676724926145,0.920357271268342,
1.46599346369761));
#62970=CARTESIAN_POINT('Ctrl Pts',(-3.13722362204439,-0.735653493827597,
1.5668466036596));
#62971=CARTESIAN_POINT('Ctrl Pts',(-3.05767999482733,-1.71583430572539,
0.22826952857563));
#62972=CARTESIAN_POINT('Ctrl Pts',(-2.97813636761028,-1.1197129206469,-1.32001413542344));
#62973=CARTESIAN_POINT('Ctrl Pts',(-2.89859274039322,0.505066028224394,
-1.65562756968869));
#62974=CARTESIAN_POINT('Ctrl Pts',(-2.81904911317615,1.66585105457453,-0.470249514994343));
#62975=CARTESIAN_POINT('Ctrl Pts',(-2.7395054859591,1.29625248362939,1.14713723724332));
#62976=CARTESIAN_POINT('Ctrl Pts',(-2.65996185874204,-0.264186969193862,
1.7106722619139));
#62977=CARTESIAN_POINT('Ctrl Pts',(-2.58041823152498,-1.58192320844134,
0.702647354631853));
#62978=CARTESIAN_POINT('Ctrl Pts',(-2.50087460430791,-1.44637866144143,
-0.950885434813853));
#62979=CARTESIAN_POINT('Ctrl Pts',(-2.42133097709086,0.0179246439767291,
-1.73085904956586));
#62980=CARTESIAN_POINT('Ctrl Pts',(-2.3417873498738,1.46576094226225,-0.920727539780172));
#62981=CARTESIAN_POINT('Ctrl Pts',(-2.26224372265674,1.56703237371457,0.735257697904209));
#62982=CARTESIAN_POINT('Ctrl Pts',(-2.18270009543968,0.228702926789087,
1.71577659188141));
#62983=CARTESIAN_POINT('Ctrl Pts',(-2.10315646822262,-1.31973126292469,
1.12004630980263));
#62984=CARTESIAN_POINT('Ctrl Pts',(-2.02361284100556,-1.65575509266798,
-0.504647814653044));
#62985=CARTESIAN_POINT('Ctrl Pts',(-1.9440692137885,-0.470670279664775,
-1.66573221954342));
#62986=CARTESIAN_POINT('Ctrl Pts',(-1.86452558657144,1.14680977693736,-1.2965422010826));
#62987=CARTESIAN_POINT('Ctrl Pts',(-1.78498195935438,1.71073894075879,0.263754861761375));
#62988=CARTESIAN_POINT('Ctrl Pts',(-1.70543833213732,0.70304690921405,1.58174566996773));
#62989=CARTESIAN_POINT('Ctrl Pts',(-1.62589470492026,-0.950520054074415,
1.44661881076732));
#62990=CARTESIAN_POINT('Ctrl Pts',(-1.5463510777032,-1.73086353544171,-0.017487461036164));
#62991=CARTESIAN_POINT('Ctrl Pts',(-1.46680745048614,-0.921097723940694,
-1.46552829253389));
#62992=CARTESIAN_POINT('Ctrl Pts',(-1.38726382326908,0.734861806468727,
-1.5672181097888));
#62993=CARTESIAN_POINT('Ctrl Pts',(-1.30772019605202,1.71571886081011,-0.229136185143489));
#62994=CARTESIAN_POINT('Ctrl Pts',(-1.22817656883497,1.12037945241918,1.319448068468));
#62995=CARTESIAN_POINT('Ctrl Pts',(-1.1486329416179,-0.504229236589193,
1.6558829612631));
#62996=CARTESIAN_POINT('Ctrl Pts',(-1.06908931440084,-1.6656139089254,0.471090157824471));
#62997=CARTESIAN_POINT('Ctrl Pts',(-0.98954568718378,-1.29683063876905,
-1.14648061787195));
#62998=CARTESIAN_POINT('Ctrl Pts',(-0.910002059966725,0.263320465525717,
-1.71080859580406));
#62999=CARTESIAN_POINT('Ctrl Pts',(-0.830458432749663,1.58157234275566,
-0.703440562983143));
#63000=CARTESIAN_POINT('Ctrl Pts',(-0.750914805532606,1.44685068332373,
0.950143498150224));
#63001=CARTESIAN_POINT('Ctrl Pts',(-0.671371178315544,-0.0170347429126065,
1.73088900618291));
#63002=CARTESIAN_POINT('Ctrl Pts',(-0.591827551098487,-1.46532503311589,
0.921427810374316));
#63003=CARTESIAN_POINT('Ctrl Pts',(-0.512283923881428,-1.56734778302374,
-0.734389871816786));
#63004=CARTESIAN_POINT('Ctrl Pts',(-0.432740296664362,-0.229675670455208,
-1.71580528473636));
#63005=CARTESIAN_POINT('Ctrl Pts',(-0.353196669447305,1.31936664475697,
-1.12043850518328));
#63006=CARTESIAN_POINT('Ctrl Pts',(-0.273653042230246,1.65562583122791,
0.503288797893469));
#63007=CARTESIAN_POINT('Ctrl Pts',(-0.194109415013187,0.472255537838747,
1.66650068200683));
#63008=CARTESIAN_POINT('Ctrl Pts',(-0.114565787796127,-1.14769222032782,
1.29508639656957));
#63009=CARTESIAN_POINT('Ctrl Pts',(-0.0615367029847541,-1.5205814962436,
0.259698171561206));
#63010=CARTESIAN_POINT('Ctrl Pts',(-0.0350221605790679,-1.44652267833248,
-0.222270985668021));
#63011=CARTESIAN_POINT('Ctrl Pts',(-0.547155045842891,-1.46121426462895,
-0.000470658046818673));
#63012=CARTESIAN_POINT('Ctrl Pts',(-0.535531338522404,-1.46184924216179,
-0.215008973536607));
#63013=CARTESIAN_POINT('Ctrl Pts',(-0.523907631201916,-1.41768133724367,
-0.429300105994831));
#63014=CARTESIAN_POINT('Ctrl Pts',(-0.512283923881429,-1.32739863927768,
-0.621989493604839));
#63015=CARTESIAN_POINT('Ctrl Pts',(-0.485769381475741,-1.12145707883424,
-1.06152834278995));
#63016=CARTESIAN_POINT('Ctrl Pts',(-0.459254839070054,-0.675566374644769,
-1.38866681376314));
#63017=CARTESIAN_POINT('Ctrl Pts',(-0.432740296664367,-0.194447303347988,
-1.45300825265757));
#63018=CARTESIAN_POINT('Ctrl Pts',(-0.40622575425868,0.286671767948793,
-1.51734969155201));
#63019=CARTESIAN_POINT('Ctrl Pts',(-0.379711211852995,0.80301920635284,
-1.31889409836768));
#63020=CARTESIAN_POINT('Ctrl Pts',(-0.353196669447309,1.11723612330005,
-0.949045084596062));
#63021=CARTESIAN_POINT('Ctrl Pts',(-0.326682127041623,1.43145304024725,
-0.579196070824442));
#63022=CARTESIAN_POINT('Ctrl Pts',(-0.300167584635933,1.5435394357376,-0.037953636465458));
#63023=CARTESIAN_POINT('Ctrl Pts',(-0.273653042230246,1.40235425125123,
0.426536228066234));
#63024=CARTESIAN_POINT('Ctrl Pts',(-0.249102028153501,1.27162450307314,
0.856628402697813));
#63025=CARTESIAN_POINT('Ctrl Pts',(-0.224551014076758,0.923746142995881,
1.22091487580054));
#63026=CARTESIAN_POINT('Ctrl Pts',(-0.200000000000013,0.502021735097343,
1.37727613462784));
#63027=CARTESIAN_POINT('',(-34.6365,-0.684664424539681,-0.958295198918239));
#63028=CARTESIAN_POINT('Ctrl Pts',(-34.6365,-0.686154072602779,-0.9596222324959));
#63029=CARTESIAN_POINT('Ctrl Pts',(-34.6365,-0.7119101001333,-0.945613082101837));
#63030=CARTESIAN_POINT('Ctrl Pts',(-34.6365,-0.737057208054438,-0.930606615436407));
#63031=CARTESIAN_POINT('Ctrl Pts',(-34.6365,-0.761530234615434,-0.914615833182014));
#63032=CARTESIAN_POINT('Ctrl Pts',(-34.6365,-0.801891049947194,-0.888243900475965));
#63033=CARTESIAN_POINT('Ctrl Pts',(-34.6365,-0.840419847997269,-0.859197627341817));
#63034=CARTESIAN_POINT('Ctrl Pts',(-34.6365,-0.877044577847601,-0.827775063525897));
#63035=CARTESIAN_POINT('Ctrl Pts',(-34.6365,-0.891050333973354,-0.815758680949148));
#63036=CARTESIAN_POINT('Ctrl Pts',(-34.6365,-0.904777454305529,-0.803394278639855));
#63037=CARTESIAN_POINT('Ctrl Pts',(-34.6365,-0.918221120557909,-0.790696745740664));
#63038=CARTESIAN_POINT('Ctrl Pts',(-34.6365,-0.926551929996928,-0.782828302345611));
#63039=CARTESIAN_POINT('Ctrl Pts',(-34.6365,-0.934775354469558,-0.774830435851512));
#63040=CARTESIAN_POINT('Ctrl Pts',(-34.6365,-0.942885419604258,-0.766711271506816));
#63041=CARTESIAN_POINT('Ctrl Pts',(-34.6365,-0.978536944636376,-0.731019746708046));
#63042=CARTESIAN_POINT('Ctrl Pts',(-34.6365,-1.01191327669552,-0.693076341324169));
#63043=CARTESIAN_POINT('Ctrl Pts',(-34.6365,-1.04293679416646,-0.653208812595354));
#63044=CARTESIAN_POINT('Ctrl Pts',(-34.6365,-1.06541205389432,-0.624326431230085));
#63045=CARTESIAN_POINT('Ctrl Pts',(-34.6365,-1.08665213278273,-0.594432978370132));
#63046=CARTESIAN_POINT('Ctrl Pts',(-34.6365,-1.10661916861093,-0.563638328343162));
#63047=CARTESIAN_POINT('Ctrl Pts',(-34.6365,-1.11501890060192,-0.550683635958747));
#63048=CARTESIAN_POINT('Ctrl Pts',(-34.6365,-1.12319324208052,-0.537569324701878));
#63049=CARTESIAN_POINT('Ctrl Pts',(-34.6365,-1.13113891356507,-0.524303043918853));
#63050=CARTESIAN_POINT('Ctrl Pts',(-34.6365,-1.1380110222127,-0.51282920900531));
#63051=CARTESIAN_POINT('Ctrl Pts',(-34.6365,-1.14471355135492,-0.50123871631513));
#63052=CARTESIAN_POINT('Ctrl Pts',(-34.6365,-1.15123207412817,-0.48955905836601));
#63053=CARTESIAN_POINT('Ctrl Pts',(-34.6365,-1.17683516242865,-0.443684352670734));
#63054=CARTESIAN_POINT('Ctrl Pts',(-34.6365,-1.19964285363905,-0.396372122447951));
#63055=CARTESIAN_POINT('Ctrl Pts',(-34.6365,-1.21956940907531,-0.347951651152172));
#63056=CARTESIAN_POINT('Ctrl Pts',(-34.6365,-1.23986899619782,-0.298624732672669));
#63057=CARTESIAN_POINT('Ctrl Pts',(-34.6365,-1.2571793448604,-0.248146802693327));
#63058=CARTESIAN_POINT('Ctrl Pts',(-34.6365,-1.27137376561068,-0.196827051143323));
#63059=CARTESIAN_POINT('Ctrl Pts',(-34.6365,-1.27949212467089,-0.167475225007287));
#63060=CARTESIAN_POINT('Ctrl Pts',(-34.6365,-1.28659049471938,-0.137847386060878));
#63061=CARTESIAN_POINT('Ctrl Pts',(-34.6365,-1.29263849229147,-0.10799760567475));
#63062=CARTESIAN_POINT('Ctrl Pts',(-34.6365,-1.29646959968636,-0.0890892458399302));
#63063=CARTESIAN_POINT('Ctrl Pts',(-34.6365,-1.2998791327864,-0.0700917822900422));
#63064=CARTESIAN_POINT('Ctrl Pts',(-34.6365,-1.3028582061524,-0.0510186173543007));
#63065=CARTESIAN_POINT('Ctrl Pts',(-34.6365,-1.30433493626761,-0.0415640274223254));
#63066=CARTESIAN_POINT('Ctrl Pts',(-34.6365,-1.30570555790757,-0.0320922880145657));
#63067=CARTESIAN_POINT('Ctrl Pts',(-34.6365,-1.30696764581746,-0.0226173109335764));
#63068=CARTESIAN_POINT('Ctrl Pts',(-34.6365,-1.31420352572401,0.0317052095011377));
#63069=CARTESIAN_POINT('Ctrl Pts',(-34.6365,-1.31789275479354,0.0862397373277177));
#63070=CARTESIAN_POINT('Ctrl Pts',(-34.6365,-1.31791881756557,0.140657257014611));
#63071=CARTESIAN_POINT('Ctrl Pts',(-34.6365,-1.31792247004294,0.148283412776851));
#63072=CARTESIAN_POINT('Ctrl Pts',(-34.6365,-1.31785410762944,0.155907313822103));
#63073=CARTESIAN_POINT('Ctrl Pts',(-34.6365,-1.31771333721581,0.163528092935519));
#63074=CARTESIAN_POINT('Ctrl Pts',(-34.6365,-1.31674443923682,0.21598057418652));
#63075=CARTESIAN_POINT('Ctrl Pts',(-34.6365,-1.3123496251762,0.268284454830481));
#63076=CARTESIAN_POINT('Ctrl Pts',(-34.6365,-1.30473184284742,0.320221776691518));
#63077=CARTESIAN_POINT('Ctrl Pts',(-34.6365,-1.3006747321352,0.347882775101802));
#63078=CARTESIAN_POINT('Ctrl Pts',(-34.6365,-1.29570254950683,0.375439959013181));
#63079=CARTESIAN_POINT('Ctrl Pts',(-34.6365,-1.28984013681239,0.402860769972335));
#63080=CARTESIAN_POINT('Ctrl Pts',(-34.6365,-1.28632199418306,0.419316507395516));
#63081=CARTESIAN_POINT('Ctrl Pts',(-34.6365,-1.28248316633568,0.435723131009655));
#63082=CARTESIAN_POINT('Ctrl Pts',(-34.6365,-1.27832836254595,0.452073542754125));
#63083=CARTESIAN_POINT('Ctrl Pts',(-34.6365,-1.27547249914963,0.463312230494656));
#63084=CARTESIAN_POINT('Ctrl Pts',(-34.6365,-1.27246679788216,0.474525738156413));
#63085=CARTESIAN_POINT('Ctrl Pts',(-34.6365,-1.26931881447351,0.485691489535342));
#63086=CARTESIAN_POINT('Ctrl Pts',(-34.6365,-1.25443545775983,0.538482066605106));
#63087=CARTESIAN_POINT('Ctrl Pts',(-34.6365,-1.23635097763686,0.590308106442404));
#63088=CARTESIAN_POINT('Ctrl Pts',(-34.6365,-1.21530442574023,0.640933424389205));
#63089=CARTESIAN_POINT('Ctrl Pts',(-34.6365,-1.19380245740259,0.692654199788485));
#63090=CARTESIAN_POINT('Ctrl Pts',(-34.6365,-1.16920862107615,0.743122685571138));
#63091=CARTESIAN_POINT('Ctrl Pts',(-34.6365,-1.14172291998422,0.792087274667335));
#63092=CARTESIAN_POINT('Ctrl Pts',(-34.6365,-1.12633431912328,0.819501402304143));
#63093=CARTESIAN_POINT('Ctrl Pts',(-34.6365,-1.11003826917362,0.846444039154066));
#63094=CARTESIAN_POINT('Ctrl Pts',(-34.6365,-1.09286303313459,0.872869290765076));
#63095=CARTESIAN_POINT('Ctrl Pts',(-34.6365,-1.08109837366658,0.89097000774234));
#63096=CARTESIAN_POINT('Ctrl Pts',(-34.6365,-1.06892110442247,0.908827940355749));
#63097=CARTESIAN_POINT('Ctrl Pts',(-34.6365,-1.05633909029096,0.92642773863922));
#63098=CARTESIAN_POINT('Ctrl Pts',(-34.6365,-1.04773945000675,0.938456968040044));
#63099=CARTESIAN_POINT('Ctrl Pts',(-34.6365,-1.03894684652451,0.950370403618958));
#63100=CARTESIAN_POINT('Ctrl Pts',(-34.6365,-1.0299848727059,0.962135775346617));
#63101=CARTESIAN_POINT('Ctrl Pts',(-34.6365,-0.994691270463756,1.00846958064347));
#63102=CARTESIAN_POINT('Ctrl Pts',(-34.6365,-0.956729926976582,1.05257580844336));
#63103=CARTESIAN_POINT('Ctrl Pts',(-34.6365,-0.916323904549539,1.09419408100751));
#63104=CARTESIAN_POINT('Ctrl Pts',(-34.6365,-0.874305894879269,1.13747270320345));
#63105=CARTESIAN_POINT('Ctrl Pts',(-34.6365,-0.829644031989242,1.1780622586008));
#63106=CARTESIAN_POINT('Ctrl Pts',(-34.6365,-0.782534111930377,1.21564789997407));
#63107=CARTESIAN_POINT('Ctrl Pts',(-34.6365,-0.738322170255781,1.25092145132208));
#63108=CARTESIAN_POINT('Ctrl Pts',(-34.6365,-0.691953185744718,1.28355000577543));
#63109=CARTESIAN_POINT('Ctrl Pts',(-34.6365,-0.643551181830037,1.31323998384329));
#63110=CARTESIAN_POINT('Ctrl Pts',(-34.6365,-0.640378555707157,1.31518608508678));
#63111=CARTESIAN_POINT('Ctrl Pts',(-34.6365,-0.637197183227053,1.31711954607524));
#63112=CARTESIAN_POINT('Ctrl Pts',(-34.6365,-0.634007094575281,1.31904027763682));
#63113=CARTESIAN_POINT('Ctrl Pts',(-34.6365,-0.686154072602774,-0.959622232495904));
#63114=CARTESIAN_POINT('Ctrl Pts',(-34.6119489859232,-0.390562334310552,
-1.1685227208061));
#63115=CARTESIAN_POINT('Ctrl Pts',(-34.5608834294408,0.441559859931502,
-1.30438298146528));
#63116=CARTESIAN_POINT('Ctrl Pts',(-34.4833033305527,1.34388692616717,-0.366485362373245));
#63117=CARTESIAN_POINT('Ctrl Pts',(-34.4037597033356,1.03476789300364,0.932740929113639));
#63118=CARTESIAN_POINT('Ctrl Pts',(-34.3242160761186,-0.225138742279001,
1.37459976780186));
#63119=CARTESIAN_POINT('Ctrl Pts',(-34.2603404700946,-1.07071564015608,
0.715550826767906));
#63120=CARTESIAN_POINT('Ctrl Pts',(-34.2229794064764,-1.17675281276781,
0.161639855406849));
#63121=CARTESIAN_POINT('Ctrl Pts',(-34.2121328852638,-1.17605840265479,
0.000574308414346206));
#63122=CARTESIAN_POINT('Origin',(-34.6365,-3.28582941601228E-17,0.));
#63123=CARTESIAN_POINT('',(-34.6365,-1.4635,-1.79227059055215E-16));
#63124=CARTESIAN_POINT('Origin',(-34.6365,0.,0.));
#63125=CARTESIAN_POINT('Origin',(-34.6365,0.,0.));
#63126=CARTESIAN_POINT('',(-34.6365,0.6846644245395,-0.958295198918368));
#63127=CARTESIAN_POINT('Ctrl Pts',(-34.6365,0.635548045752339,1.32098221395624));
#63128=CARTESIAN_POINT('Ctrl Pts',(-34.6365,0.666498491669791,1.30253980504351));
#63129=CARTESIAN_POINT('Ctrl Pts',(-34.6365,0.696670008128909,1.28290514074601));
#63130=CARTESIAN_POINT('Ctrl Pts',(-34.6365,0.725984184660265,1.26207365955444));
#63131=CARTESIAN_POINT('Ctrl Pts',(-34.6365,0.773073530585445,1.22861064131428));
#63132=CARTESIAN_POINT('Ctrl Pts',(-34.6365,0.817952842411402,1.19206056398115));
#63133=CARTESIAN_POINT('Ctrl Pts',(-34.6365,0.860470315479712,1.15273759731246));
#63134=CARTESIAN_POINT('Ctrl Pts',(-34.6365,0.882577900258638,1.13229104306898));
#63135=CARTESIAN_POINT('Ctrl Pts',(-34.6365,0.904046247749025,1.1110942774146));
#63136=CARTESIAN_POINT('Ctrl Pts',(-34.6365,0.924849238970118,1.08918893459142));
#63137=CARTESIAN_POINT('Ctrl Pts',(-34.6365,0.933737523857988,1.07982965901852));
#63138=CARTESIAN_POINT('Ctrl Pts',(-34.6365,0.942504822960868,1.07034025158081));
#63139=CARTESIAN_POINT('Ctrl Pts',(-34.6365,0.951138112600303,1.06073646803148));
#63140=CARTESIAN_POINT('Ctrl Pts',(-34.6365,0.989630872686237,1.01791662165531));
#63141=CARTESIAN_POINT('Ctrl Pts',(-34.6365,1.02551732004391,0.972769428249441));
#63142=CARTESIAN_POINT('Ctrl Pts',(-34.6365,1.05864549743232,0.925607080115083));
#63143=CARTESIAN_POINT('Ctrl Pts',(-34.6365,1.0806661582941,0.894257752878159));
#63144=CARTESIAN_POINT('Ctrl Pts',(-34.6365,1.10146719775831,0.862017405404437));
#63145=CARTESIAN_POINT('Ctrl Pts',(-34.6365,1.12099192934309,0.828973605276758));
#63146=CARTESIAN_POINT('Ctrl Pts',(-34.6365,1.12904366504594,0.815346788227294));
#63147=CARTESIAN_POINT('Ctrl Pts',(-34.6365,1.13687822907506,0.801583312066227));
#63148=CARTESIAN_POINT('Ctrl Pts',(-34.6365,1.14449112932449,0.787689263461989));
#63149=CARTESIAN_POINT('Ctrl Pts',(-34.6365,1.15119354448111,0.775456910626577));
#63150=CARTESIAN_POINT('Ctrl Pts',(-34.6365,1.15772571146099,0.763119959343411));
#63151=CARTESIAN_POINT('Ctrl Pts',(-34.6365,1.16407270727518,0.750706322535687));
#63152=CARTESIAN_POINT('Ctrl Pts',(-34.6365,1.18968499603057,0.700613072164659));
#63153=CARTESIAN_POINT('Ctrl Pts',(-34.6365,1.21232701568682,0.649200916818433));
#63154=CARTESIAN_POINT('Ctrl Pts',(-34.6365,1.23185338093466,0.596758023613943));
#63155=CARTESIAN_POINT('Ctrl Pts',(-34.6365,1.25088764177288,0.545636798762549));
#63156=CARTESIAN_POINT('Ctrl Pts',(-34.6365,1.26696143620811,0.493535096364606));
#63157=CARTESIAN_POINT('Ctrl Pts',(-34.6365,1.27989180385019,0.440714302555275));
#63158=CARTESIAN_POINT('Ctrl Pts',(-34.6365,1.28743198375341,0.409912526536342));
#63159=CARTESIAN_POINT('Ctrl Pts',(-34.6365,1.29390232703675,0.378866200024003));
#63160=CARTESIAN_POINT('Ctrl Pts',(-34.6365,1.29925840715535,0.347628297483629));
#63161=CARTESIAN_POINT('Ctrl Pts',(-34.6365,1.30273792407846,0.327334947099519));
#63162=CARTESIAN_POINT('Ctrl Pts',(-34.6365,1.30574706385875,0.306960769457363));
#63163=CARTESIAN_POINT('Ctrl Pts',(-34.6365,1.30827220879121,0.286520718592337));
#63164=CARTESIAN_POINT('Ctrl Pts',(-34.6365,1.30983744822857,0.273850723573731));
#63165=CARTESIAN_POINT('Ctrl Pts',(-34.6365,1.31121690877827,0.261151572677647));
#63166=CARTESIAN_POINT('Ctrl Pts',(-34.6365,1.31240507505011,0.248453673487265));
#63167=CARTESIAN_POINT('Ctrl Pts',(-34.6365,1.31731668013685,0.195963489467908));
#63168=CARTESIAN_POINT('Ctrl Pts',(-34.6365,1.3189760904167,0.143408381037281));
#63169=CARTESIAN_POINT('Ctrl Pts',(-34.6365,1.31722292331031,0.0910320624908964));
#63170=CARTESIAN_POINT('Ctrl Pts',(-34.6365,1.31692479917861,0.0821255273229491));
#63171=CARTESIAN_POINT('Ctrl Pts',(-34.6365,1.31652787382802,0.0732241778386358));
#63172=CARTESIAN_POINT('Ctrl Pts',(-34.6365,1.31603120806162,0.0643292382201927));
#63173=CARTESIAN_POINT('Ctrl Pts',(-34.6365,1.31309184640608,0.0116873083521665));
#63174=CARTESIAN_POINT('Ctrl Pts',(-34.6365,1.30666269163376,-0.0407318065592056));
#63175=CARTESIAN_POINT('Ctrl Pts',(-34.6365,1.29689813812491,-0.0926593050314029));
#63176=CARTESIAN_POINT('Ctrl Pts',(-34.6365,1.29219527731605,-0.117668927565173));
#63177=CARTESIAN_POINT('Ctrl Pts',(-34.6365,1.28671806309696,-0.142564201344602));
#63178=CARTESIAN_POINT('Ctrl Pts',(-34.6365,1.28048041312089,-0.167312876218102));
#63179=CARTESIAN_POINT('Ctrl Pts',(-34.6365,1.27563401943483,-0.186541563641289));
#63180=CARTESIAN_POINT('Ctrl Pts',(-34.6365,1.27032853396833,-0.205681726868499));
#63181=CARTESIAN_POINT('Ctrl Pts',(-34.6365,1.26456972207496,-0.224717452852664));
#63182=CARTESIAN_POINT('Ctrl Pts',(-34.6365,1.26182301144504,-0.23379669209109));
#63183=CARTESIAN_POINT('Ctrl Pts',(-34.6365,1.25897402305304,-0.242849070418405));
#63184=CARTESIAN_POINT('Ctrl Pts',(-34.6365,1.25602686354908,-0.251863406655858));
#63185=CARTESIAN_POINT('Ctrl Pts',(-34.6365,1.23970756016791,-0.30177848171073));
#63186=CARTESIAN_POINT('Ctrl Pts',(-34.6365,1.22035602282228,-0.350615852547003));
#63187=CARTESIAN_POINT('Ctrl Pts',(-34.6365,1.19814539365861,-0.398117840475043));
#63188=CARTESIAN_POINT('Ctrl Pts',(-34.6365,1.17602990897011,-0.445416342419949));
#63189=CARTESIAN_POINT('Ctrl Pts',(-34.6365,1.15107898465775,-0.491391780007035));
#63190=CARTESIAN_POINT('Ctrl Pts',(-34.6365,1.12342395860753,-0.53575743875993));
#63191=CARTESIAN_POINT('Ctrl Pts',(-34.6365,1.10893424546816,-0.559002604662186));
#63192=CARTESIAN_POINT('Ctrl Pts',(-34.6365,1.09370162121455,-0.581805236030971));
#63193=CARTESIAN_POINT('Ctrl Pts',(-34.6365,1.07774169884391,-0.604119277574196));
#63194=CARTESIAN_POINT('Ctrl Pts',(-34.6365,1.06683927858885,-0.619362275180545));
#63195=CARTESIAN_POINT('Ctrl Pts',(-34.6365,1.05559742596417,-0.634377204151687));
#63196=CARTESIAN_POINT('Ctrl Pts',(-34.6365,1.04402064985082,-0.649148328629702));
#63197=CARTESIAN_POINT('Ctrl Pts',(-34.6365,1.03779477786861,-0.657092088544632));
#63198=CARTESIAN_POINT('Ctrl Pts',(-34.6365,1.03147122864614,-0.664966126131085));
#63199=CARTESIAN_POINT('Ctrl Pts',(-34.6365,1.02506186124697,-0.672754796849972));
#63200=CARTESIAN_POINT('Ctrl Pts',(-34.6365,0.993012679416858,-0.711700999889751));
#63201=CARTESIAN_POINT('Ctrl Pts',(-34.6365,0.958759462630057,-0.748595252324693));
#63202=CARTESIAN_POINT('Ctrl Pts',(-34.6365,0.922431964225527,-0.783185558398445));
#63203=CARTESIAN_POINT('Ctrl Pts',(-34.6365,0.886691317016434,-0.817217076684392));
#63204=CARTESIAN_POINT('Ctrl Pts',(-34.6365,0.8489421255063,-0.849019106260595));
#63205=CARTESIAN_POINT('Ctrl Pts',(-34.6365,0.809283769251354,-0.878307498888002));
#63206=CARTESIAN_POINT('Ctrl Pts',(-34.6365,0.769625412996408,-0.907595891515409));
#63207=CARTESIAN_POINT('Ctrl Pts',(-34.6365,0.728057253858435,-0.934371344062744));
#63208=CARTESIAN_POINT('Ctrl Pts',(-34.6365,0.684664424539256,-0.958295198918542));
#63209=CARTESIAN_POINT('Origin',(-34.6365,0.,0.));
#63210=CARTESIAN_POINT('Origin',(-35.5608671147362,0.,0.));
#63211=CARTESIAN_POINT('Ctrl Pts',(-34.6365,0.684664424539256,-0.958295198918542));
#63212=CARTESIAN_POINT('Ctrl Pts',(-34.6099854575943,1.00396030307469,-0.7301707867521));
#63213=CARTESIAN_POINT('Ctrl Pts',(-34.556956372783,1.39099115610471,0.0663998364373292));
#63214=CARTESIAN_POINT('Ctrl Pts',(-34.4774127455658,0.694817159188923,
1.20840932237519));
#63215=CARTESIAN_POINT('Ctrl Pts',(-34.3978691183489,-0.640240458638742,
1.23665911837698));
#63216=CARTESIAN_POINT('Ctrl Pts',(-34.3423539080722,-1.16129644075106,
0.464741691095696));
#63217=CARTESIAN_POINT('Ctrl Pts',(-34.3133532402014,-1.17949500306512,
0.0373805274982975));
#63218=CARTESIAN_POINT('Ctrl Pts',(-34.3108671147362,-1.17925499677644,
0.000722179416794018));
#63219=CARTESIAN_POINT('Ctrl Pts',(-34.8014778394209,0.850780204044596,
-1.19080027477568));
#63220=CARTESIAN_POINT('Ctrl Pts',(-34.7749632970152,1.24754481303337,-0.90732748580884));
#63221=CARTESIAN_POINT('Ctrl Pts',(-34.7219342122039,1.72847850304328,0.0825100069000186));
#63222=CARTESIAN_POINT('Ctrl Pts',(-34.6423905849868,0.863396232199179,
1.50159799897799));
#63223=CARTESIAN_POINT('Ctrl Pts',(-34.5628469577697,-0.795577933532765,
1.53670186350626));
#63224=CARTESIAN_POINT('Ctrl Pts',(-34.4833033305527,-1.72329896479418,
0.162331246392712));
#63225=CARTESIAN_POINT('Ctrl Pts',(-34.4037597033356,-1.06805600758911,
-1.36234908588761));
#63226=CARTESIAN_POINT('Ctrl Pts',(-34.3242160761186,0.568491528314387,
-1.63484710452143));
#63227=CARTESIAN_POINT('Ctrl Pts',(-34.2446724489015,1.68272306300853,-0.405770608944271));
#63228=CARTESIAN_POINT('Ctrl Pts',(-34.1651288216845,1.25109966684745,1.19625105692336));
#63229=CARTESIAN_POINT('Ctrl Pts',(-34.0855851944674,-0.329898722146615,
1.69921054064198));
#63230=CARTESIAN_POINT('Ctrl Pts',(-34.0060415672503,-1.60781789259073,
0.641187468103347));
#63231=CARTESIAN_POINT('Ctrl Pts',(-33.9264979400333,-1.40867154360034,
-1.00590667876807));
#63232=CARTESIAN_POINT('Ctrl Pts',(-33.8469543128162,0.0845950055721448,
-1.72888150200373));
#63233=CARTESIAN_POINT('Ctrl Pts',(-33.7674106855992,1.50014467527073,-0.863574913031011));
#63234=CARTESIAN_POINT('Ctrl Pts',(-33.6878670583821,1.53754245201339,0.795084121240462));
#63235=CARTESIAN_POINT('Ctrl Pts',(-33.608323431165,0.162430821126508,1.7233135521795));
#63236=CARTESIAN_POINT('Ctrl Pts',(-33.528779803948,-1.36190254265914,1.06837077475386));
#63237=CARTESIAN_POINT('Ctrl Pts',(-33.4492361767309,-1.63508373563369,
-0.568063115508245));
#63238=CARTESIAN_POINT('Ctrl Pts',(-33.3696925495139,-0.406146596378477,
-1.6826286527699));
#63239=CARTESIAN_POINT('Ctrl Pts',(-33.2901489222968,1.19590916357646,-1.25139750262871));
#63240=CARTESIAN_POINT('Ctrl Pts',(-33.2106052950798,1.69930742894605,0.329467246193458));
#63241=CARTESIAN_POINT('Ctrl Pts',(-33.1310616678627,0.641586397136989,
1.60765707275096));
#63242=CARTESIAN_POINT('Ctrl Pts',(-33.0515180406457,-1.00554704922936,
1.40892495536101));
#63243=CARTESIAN_POINT('Ctrl Pts',(-32.9719744134285,-1.72890480566619,
-0.0841579713322476));
#63244=CARTESIAN_POINT('Ctrl Pts',(-32.8924307862115,-0.863952760758447,
-1.49992666957161));
#63245=CARTESIAN_POINT('Ctrl Pts',(-32.8128871589944,0.794695172738762,
-1.53774314294755));
#63246=CARTESIAN_POINT('Ctrl Pts',(-32.7333435317774,1.72327275966808,-0.162866159028769));
#63247=CARTESIAN_POINT('Ctrl Pts',(-32.6537999045603,1.06871459261237,1.3616326630319));
#63248=CARTESIAN_POINT('Ctrl Pts',(-32.5742562773433,-0.567650007920692,
1.63522715811347));
#63249=CARTESIAN_POINT('Ctrl Pts',(-32.4947126501262,-1.68252605239498,
0.406571608589262));
#63250=CARTESIAN_POINT('Ctrl Pts',(-32.4151690229091,-1.25169951705268,
-1.1955930364733));
#63251=CARTESIAN_POINT('Ctrl Pts',(-32.3356253956921,0.329037992840854,
-1.69939059348022));
#63252=CARTESIAN_POINT('Ctrl Pts',(-32.256081768475,1.60749496826621,-0.641992458602764));
#63253=CARTESIAN_POINT('Ctrl Pts',(-32.176538141258,1.40917890001414,1.00519113488724));
#63254=CARTESIAN_POINT('Ctrl Pts',(-32.0969945140409,-0.0837212598430693,
1.72892600783361));
#63255=CARTESIAN_POINT('Ctrl Pts',(-32.0174508868239,-1.49970839530019,
0.864331602438092));
#63256=CARTESIAN_POINT('Ctrl Pts',(-31.9379072596068,-1.53794382684947,
-0.79430672624796));
#63257=CARTESIAN_POINT('Ctrl Pts',(-31.8583636323897,-0.163301438553533,
-1.72323156600474));
#63258=CARTESIAN_POINT('Ctrl Pts',(-31.7788200051727,1.36136267124702,-1.06905849570687));
#63259=CARTESIAN_POINT('Ctrl Pts',(-31.6992763779556,1.63537048958156,0.567236944947783));
#63260=CARTESIAN_POINT('Ctrl Pts',(-31.6197327507385,0.406996587841936,
1.68242330208339));
#63261=CARTESIAN_POINT('Ctrl Pts',(-31.5401891235215,-1.19527682939084,
1.2520014740524));
#63262=CARTESIAN_POINT('Ctrl Pts',(-31.4606454963044,-1.69947365153686,
-0.32860873031615));
#63263=CARTESIAN_POINT('Ctrl Pts',(-31.3811018690874,-0.642398478081434,
-1.60733275499092));
#63264=CARTESIAN_POINT('Ctrl Pts',(-31.3015582418703,1.0048351558706,-1.40943275803939));
#63265=CARTESIAN_POINT('Ctrl Pts',(-31.2220146146532,1.72894709997597,0.0832845447410718));
#63266=CARTESIAN_POINT('Ctrl Pts',(-31.1424709874362,0.86471038882106,1.49949002443263));
#63267=CARTESIAN_POINT('Ctrl Pts',(-31.0629273602191,-0.793918228999244,
1.5381444131065));
#63268=CARTESIAN_POINT('Ctrl Pts',(-30.9833837330021,-1.72319026243643,
0.163736707406421));
#63269=CARTESIAN_POINT('Ctrl Pts',(-30.903840105785,-1.06940233057072,-1.36109259247046));
#63270=CARTESIAN_POINT('Ctrl Pts',(-30.824296478568,0.566823845772114,-1.63551371677897));
#63271=CARTESIAN_POINT('Ctrl Pts',(-30.7447528513508,1.68232044443492,-0.407421541090209));
#63272=CARTESIAN_POINT('Ctrl Pts',(-30.6652092241339,1.252303351168,1.19496054602713));
#63273=CARTESIAN_POINT('Ctrl Pts',(-30.5856655969168,-0.328179446823656,
1.69955660117295));
#63274=CARTESIAN_POINT('Ctrl Pts',(-30.5061219696997,-1.60717043916454,
0.642804456568018));
#63275=CARTESIAN_POINT('Ctrl Pts',(-30.4265783424826,-1.40968652613872,
-1.00447911274003));
#63276=CARTESIAN_POINT('Ctrl Pts',(-30.3470347152656,0.0828478243250561,
-1.72896808180852));
#63277=CARTESIAN_POINT('Ctrl Pts',(-30.2674910880485,1.49927155789386,-0.865089120032475));
#63278=CARTESIAN_POINT('Ctrl Pts',(-30.1879474608315,1.53834490122586,0.793529681096073));
#63279=CARTESIAN_POINT('Ctrl Pts',(-30.1084038336144,0.164171965812518,
1.72314884892434));
#63280=CARTESIAN_POINT('Ctrl Pts',(-30.0288602063974,-1.36082242685268,
1.06974609720383));
#63281=CARTESIAN_POINT('Ctrl Pts',(-29.9493165791803,-1.63565683962635,
-0.566410710431554));
#63282=CARTESIAN_POINT('Ctrl Pts',(-29.8697729519632,-0.407846468343938,
-1.68221747945009));
#63283=CARTESIAN_POINT('Ctrl Pts',(-29.7902293247462,1.19464418642185,-1.25260514838337));
#63284=CARTESIAN_POINT('Ctrl Pts',(-29.7106856975292,1.69963944237293,0.327750142392453));
#63285=CARTESIAN_POINT('Ctrl Pts',(-29.631142070312,0.643210394042013,1.60700802079652));
#63286=CARTESIAN_POINT('Ctrl Pts',(-29.5515984430951,-1.00412300552109,
1.40994020429639));
#63287=CARTESIAN_POINT('Ctrl Pts',(-29.4720548158779,-1.72898895332844,
-0.0824110986231344));
#63288=CARTESIAN_POINT('Ctrl Pts',(-29.3925111886609,-0.865467796048966,
-1.49905299569768));
#63289=CARTESIAN_POINT('Ctrl Pts',(-29.3129675614438,0.793141082563654,
-1.53854529119483));
#63290=CARTESIAN_POINT('Ctrl Pts',(-29.2334239342268,1.7231073254709,-0.164607213744022));
#63291=CARTESIAN_POINT('Ctrl Pts',(-29.1538803070097,1.07008979558436,1.36055217441091));
#63292=CARTESIAN_POINT('Ctrl Pts',(-29.0743366797926,-0.565997538952522,
1.63579985811459));
#63293=CARTESIAN_POINT('Ctrl Pts',(-28.9947930525756,-1.68211440713543,
0.408271369576005));
#63294=CARTESIAN_POINT('Ctrl Pts',(-28.9152494253585,-1.2529068656793,-1.19432775059517));
#63295=CARTESIAN_POINT('Ctrl Pts',(-28.8357057981415,0.327320817049945,
-1.69972217513151));
#63296=CARTESIAN_POINT('Ctrl Pts',(-28.7561621709244,1.60684549989723,-0.643616290477521));
#63297=CARTESIAN_POINT('Ctrl Pts',(-28.6766185437074,1.41019379249622,1.00376683423649));
#63298=CARTESIAN_POINT('Ctrl Pts',(-28.5970749164902,-0.0819743676631687,
1.72900971453438));
#63299=CARTESIAN_POINT('Ctrl Pts',(-28.5175312892732,-1.49883433785804,
0.865846416846369));
#63300=CARTESIAN_POINT('Ctrl Pts',(-28.4379876620562,-1.53874558300063,
-0.79275243342678));
#63301=CARTESIAN_POINT('Ctrl Pts',(-28.3584440348391,-0.165042451173157,
-1.72306569207874));
#63302=CARTESIAN_POINT('Ctrl Pts',(-28.2789004076221,1.36028183516239,-1.0704334256904));
#63303=CARTESIAN_POINT('Ctrl Pts',(-28.199356780405,1.63594277223457,0.565584331361386));
#63304=CARTESIAN_POINT('Ctrl Pts',(-28.1198131531879,0.408696244759305,
1.68201122749751));
#63305=CARTESIAN_POINT('Ctrl Pts',(-28.0402695259709,-1.19401123856729,
1.25320850303652));
#63306=CARTESIAN_POINT('Ctrl Pts',(-27.9607258987538,-1.69980479944342,
-0.326891470823519));
#63307=CARTESIAN_POINT('Ctrl Pts',(-27.8811822715368,-0.644022145848643,
-1.60668287647704));
#63308=CARTESIAN_POINT('Ctrl Pts',(-27.8016386443197,1.00341059890898,-1.41044729072205));
#63309=CARTESIAN_POINT('Ctrl Pts',(-27.7220950171026,1.72903036542503,0.0815376314730298));
#63310=CARTESIAN_POINT('Ctrl Pts',(-27.6425513898856,0.866224982400531,
1.49861558438888));
#63311=CARTESIAN_POINT('Ctrl Pts',(-27.5630077626685,-0.79236373371025,
1.53894577663048));
#63312=CARTESIAN_POINT('Ctrl Pts',(-27.4834641354515,-1.72302394875053,
0.165477678072159));
#63313=CARTESIAN_POINT('Ctrl Pts',(-27.4039205082344,-1.07077698750001,
-1.36001140912437));
#63314=CARTESIAN_POINT('Ctrl Pts',(-27.3243768810173,0.565171087684503,
-1.63608558197716));
#63315=CARTESIAN_POINT('Ctrl Pts',(-27.2448332538003,1.68190794054292,-0.409121093866723));
#63316=CARTESIAN_POINT('Ctrl Pts',(-27.1652896265832,1.2535100604358,1.19369465035841));
#63317=CARTESIAN_POINT('Ctrl Pts',(-27.0857459993662,-0.326462103740574,
1.69988731530338));
#63318=CARTESIAN_POINT('Ctrl Pts',(-27.0062023721491,-1.60652015054632,
0.644427960129485));
#63319=CARTESIAN_POINT('Ctrl Pts',(-26.926658744932,-1.41070069895768,-1.00305429956127));
#63320=CARTESIAN_POINT('Ctrl Pts',(-26.847115117715,0.0811008900805756,
-1.72905090599906));
#63321=CARTESIAN_POINT('Ctrl Pts',(-26.7675714904979,1.49839673530418,-0.866603492687293));
#63322=CARTESIAN_POINT('Ctrl Pts',(-26.6880278632808,1.5391458720716,0.791974983438858));
#63323=CARTESIAN_POINT('Ctrl Pts',(-26.6084842360638,0.165912894413254,
1.72298209548894));
#63324=CARTESIAN_POINT('Ctrl Pts',(-26.5289406088467,-1.3597408963141,1.07112048099127));
#63325=CARTESIAN_POINT('Ctrl Pts',(-26.4493969816297,-1.63622828733326,
-0.56475780794824));
#63326=CARTESIAN_POINT('Ctrl Pts',(-26.3698533544126,-0.409545916871159,
-1.68180454627825));
#63327=CARTESIAN_POINT('Ctrl Pts',(-26.2903097271955,1.19337798598872,-1.25381153785789));
#63328=CARTESIAN_POINT('Ctrl Pts',(-26.2107660999785,1.69996972270612,0.326032715828498));
#63329=CARTESIAN_POINT('Ctrl Pts',(-26.1312224727614,0.644833733294154,
1.60635732211546));
#63330=CARTESIAN_POINT('Ctrl Pts',(-26.0516788455444,-1.0026979362161,1.41095401718695));
#63331=CARTESIAN_POINT('Ctrl Pts',(-25.9721352183273,-1.72907133625517,
-0.0806641435136772));
#63332=CARTESIAN_POINT('Ctrl Pts',(-25.8925915911103,-0.866981947682513,
-1.49817779061788));
#63333=CARTESIAN_POINT('Ctrl Pts',(-25.8130479638931,0.791586182637417,
-1.53934586931123));
#63334=CARTESIAN_POINT('Ctrl Pts',(-25.7335043366762,1.72294013229662,-0.166348100168679));
#63335=CARTESIAN_POINT('Ctrl Pts',(-25.653960709459,1.07146390614228,1.35947029674884));
#63336=CARTESIAN_POINT('Ctrl Pts',(-25.574417082242,-0.564344492178976,
1.63637088829376));
#63337=CARTESIAN_POINT('Ctrl Pts',(-25.4948734550249,-1.6817010447101,0.409970713745494));
#63338=CARTESIAN_POINT('Ctrl Pts',(-25.4153298278079,-1.25411293528354,
-1.19306124547843));
#63339=CARTESIAN_POINT('Ctrl Pts',(-25.3357862005908,0.325603307114701,
-1.7000520216464));
#63340=CARTESIAN_POINT('Ctrl Pts',(-25.2562425733738,1.60619439119485,-0.645239465316747));
#63341=CARTESIAN_POINT('Ctrl Pts',(-25.1766989461567,1.4112072453937,1.00234150889622));
#63342=CARTESIAN_POINT('Ctrl Pts',(-25.0971553189396,-0.0802273918002108,
1.72909165619205));
#63343=CARTESIAN_POINT('Ctrl Pts',(-25.0176116917226,-1.49795875034397,
0.867360347362028));
#63344=CARTESIAN_POINT('Ctrl Pts',(-24.9380680645055,-1.53954576833661,
-0.791197331330738));
#63345=CARTESIAN_POINT('Ctrl Pts',(-24.8585244372885,-0.166783295310653,
-1.72289805917627));
#63346=CARTESIAN_POINT('Ctrl Pts',(-24.7789808100714,1.35919961044586,-1.0718072629311));
#63347=CARTESIAN_POINT('Ctrl Pts',(-24.6994371828543,1.63651338484955,0.563931140403065));
#63348=CARTESIAN_POINT('Ctrl Pts',(-24.6198935556373,0.41039548446264,1.68159743584507));
#63349=CARTESIAN_POINT('Ctrl Pts',(-24.5403499284202,-1.19274442884774,
1.25441425269356));
#63350=CARTESIAN_POINT('Ctrl Pts',(-24.4608063012032,-1.70013421211895,
-0.325173877626586));
#63351=CARTESIAN_POINT('Ctrl Pts',(-24.3812626739861,-0.645645156171385,
-1.60603135779488));
#63352=CARTESIAN_POINT('Ctrl Pts',(-24.3017190467691,1.00198501762436,-1.41146038356177));
#63353=CARTESIAN_POINT('Ctrl Pts',(-24.222175419552,1.72911186580841,0.0797906349680398));
#63354=CARTESIAN_POINT('Ctrl Pts',(-24.142631792335,0.867738691701698,1.49773961449641));
#63355=CARTESIAN_POINT('Ctrl Pts',(-24.0630881651179,-0.790808429543632,
1.53974556913497));
#63356=CARTESIAN_POINT('Ctrl Pts',(-23.9835445379008,-1.72285587613056,
0.167218479811407));
#63357=CARTESIAN_POINT('Ctrl Pts',(-23.9040009106837,-1.07215055133584,
-1.35892883742244));
#63358=CARTESIAN_POINT('Ctrl Pts',(-23.8244572834667,0.563517752646911,
-1.63665577699155));
#63359=CARTESIAN_POINT('Ctrl Pts',(-23.7449136562497,1.68149371968977,-0.410820228995473));
#63360=CARTESIAN_POINT('Ctrl Pts',(-23.6653700290326,1.25471549006868,1.19242753611687));
#63361=CARTESIAN_POINT('Ctrl Pts',(-23.5858264018155,-0.324744427391516,
1.70021629411854));
#63362=CARTESIAN_POINT('Ctrl Pts',(-23.5062827745985,-1.60586822192594,
0.646050805832219));
#63363=CARTESIAN_POINT('Ctrl Pts',(-23.4267391473814,-1.41171343167502,
-1.00162846242325));
#63364=CARTESIAN_POINT('Ctrl Pts',(-23.3471955201644,0.079353873044988,
-1.72913196510295));
#63365=CARTESIAN_POINT('Ctrl Pts',(-23.2676518929473,1.49752038308919,-0.868116980677408));
#63366=CARTESIAN_POINT('Ctrl Pts',(-23.1881082657303,1.53994527169359,0.790419477300873));
#63367=CARTESIAN_POINT('Ctrl Pts',(-23.1085646385131,0.167653653643207,
1.72281358316218));
#63368=CARTESIAN_POINT('Ctrl Pts',(-23.0290210112961,-1.35865797769581,
1.07249377133462));
#63369=CARTESIAN_POINT('Ctrl Pts',(-22.9494773840791,-1.63679806471068,
-0.563104328936848));
#63370=CARTESIAN_POINT('Ctrl Pts',(-22.869933756862,-0.411244947316943,
-1.68138989625081));
#63371=CARTESIAN_POINT('Ctrl Pts',(-22.7903901296449,1.19211056730603,-1.25501664738972));
#63372=CARTESIAN_POINT('Ctrl Pts',(-22.7108465024279,1.70029826763994,0.324314956436899));
#63373=CARTESIAN_POINT('Ctrl Pts',(-22.6313028752108,0.646456414273326,
1.60570498359846));
#63374=CARTESIAN_POINT('Ctrl Pts',(-22.5517592479938,-1.00127184331565,
1.41196638971731));
#63375=CARTESIAN_POINT('Ctrl Pts',(-22.4722156207767,-1.7291519540744,-0.0789171060589664));
#63376=CARTESIAN_POINT('Ctrl Pts',(-22.3926719935596,-0.868495214265015,
-1.49730105613627));
#63377=CARTESIAN_POINT('Ctrl Pts',(-22.3131283663426,0.790030474627313,
-1.54014487599972));
#63378=CARTESIAN_POINT('Ctrl Pts',(-22.2335847391255,1.72277118027384,-0.168088816778282));
#63379=CARTESIAN_POINT('Ctrl Pts',(-22.1540411119085,1.07283692290551,1.3583870312833));
#63380=CARTESIAN_POINT('Ctrl Pts',(-22.0744974846914,-0.562690869299256,
1.63694024799786));
#63381=CARTESIAN_POINT('Ctrl Pts',(-21.9949538574743,-1.68128596553483,
0.411669639399906));
#63382=CARTESIAN_POINT('Ctrl Pts',(-21.9154102302573,-1.25531772463745,
-1.19179352243544));
#63383=CARTESIAN_POINT('Ctrl Pts',(-21.8358666030402,0.323885464790162,
-1.7003801326779));
#63384=CARTESIAN_POINT('Ctrl Pts',(-21.7563229758232,1.60554164282283,-0.646861981468851));
#63385=CARTESIAN_POINT('Ctrl Pts',(-21.6767793486061,1.41221925767248,1.00091516032431));
#63386=CARTESIAN_POINT('Ctrl Pts',(-21.5972357213891,-0.0784803340378172,
1.72917183272148));
#63387=CARTESIAN_POINT('Ctrl Pts',(-21.517692094172,-1.49708163365169,0.868873392440369));
#63388=CARTESIAN_POINT('Ctrl Pts',(-21.4381484669549,-1.54034438204061,
-0.789641421547753));
#63389=CARTESIAN_POINT('Ctrl Pts',(-21.3586048397378,-0.168523969188844,
-1.72272866746823));
#63390=CARTESIAN_POINT('Ctrl Pts',(-21.2790612125208,1.35811599820218,-1.07318000602664));
#63391=CARTESIAN_POINT('Ctrl Pts',(-21.1995175853037,1.63708232684401,0.562277373760544));
#63392=CARTESIAN_POINT('Ctrl Pts',(-21.1199739580867,0.412094305217296,
1.68118192754845));
#63393=CARTESIAN_POINT('Ctrl Pts',(-21.0404303308696,-1.19147640152535,
1.25561872179266));
#63394=CARTESIAN_POINT('Ctrl Pts',(-20.9608867036526,-1.7004618892272,-0.323455952478681));
#63395=CARTESIAN_POINT('Ctrl Pts',(-20.8813430764355,-0.647267507392897,
-1.6053781996095));
#63396=CARTESIAN_POINT('Ctrl Pts',(-20.8017994492184,1.00055841347199,-1.41247203552441));
#63397=CARTESIAN_POINT('Ctrl Pts',(-20.7222558220014,1.72919160104291,0.0780435570094322));
#63398=CARTESIAN_POINT('Ctrl Pts',(-20.6427121947843,0.869251515179363,
1.49686211564941));
#63399=CARTESIAN_POINT('Ctrl Pts',(-20.5631685675672,-0.789252318087039,
1.54054378980355));
#63400=CARTESIAN_POINT('Ctrl Pts',(-20.4836249403502,-1.72268604474808,
0.168959110847153));
#63401=CARTESIAN_POINT('Ctrl Pts',(-20.4040813131331,-1.0735230206761,-1.35784487846974));
#63402=CARTESIAN_POINT('Ctrl Pts',(-20.3245376859161,0.561863842347068,
-1.63722430124007));
#63403=CARTESIAN_POINT('Ctrl Pts',(-20.244994058699,1.68107778229831,-0.412518944741988));
#63404=CARTESIAN_POINT('Ctrl Pts',(-20.1654504314819,1.25591963883615,1.19115920459598));
#63405=CARTESIAN_POINT('Ctrl Pts',(-20.0859068042649,-0.323026419529885,
1.70054353728264));
#63406=CARTESIAN_POINT('Ctrl Pts',(-20.0063631770479,-1.60521465396887,
0.647672992019612));
#63407=CARTESIAN_POINT('Ctrl Pts',(-19.9268195498308,-1.41272472325696,
-1.00020160278146));
#63408=CARTESIAN_POINT('Ctrl Pts',(-19.8472759226137,0.0776067750016528,
-1.72921125903745));
#63409=CARTESIAN_POINT('Ctrl Pts',(-19.7677322953967,1.49664250214346,-0.869629582457851));
#63410=CARTESIAN_POINT('Ctrl Pts',(-19.6881886681796,1.5407430992758,0.788863164269974));
#63411=CARTESIAN_POINT('Ctrl Pts',(-19.6086450409625,0.16939424172542,1.72264331211609));
#63412=CARTESIAN_POINT('Ctrl Pts',(-19.5291014137455,-1.35757367210328,
1.07386596683201));
#63413=CARTESIAN_POINT('Ctrl Pts',(-19.4495577865284,-1.63736617117698,
-0.561450275085237));
#63414=CARTESIAN_POINT('Ctrl Pts',(-19.3700141593114,-0.412943557946916,
-1.68097352979105));
#63415=CARTESIAN_POINT('Ctrl Pts',(-19.2904705320943,1.19084193166757,-1.2562204757487));
#63416=CARTESIAN_POINT('Ctrl Pts',(-19.2109269048772,1.70062507683899,0.322596865971154));
#63417=CARTESIAN_POINT('Ctrl Pts',(-19.1313832776602,0.648078435323101,
1.6050510059114));
#63418=CARTESIAN_POINT('Ctrl Pts',(-19.0518396504431,-0.999844728275466,
1.41297732085402));
#63419=CARTESIAN_POINT('Ctrl Pts',(-18.9722960232261,-1.72923080670383,
-0.0771699880423723));
#63420=CARTESIAN_POINT('Ctrl Pts',(-18.892752396009,-0.870007594251728,
-1.49642279314783));
#63421=CARTESIAN_POINT('Ctrl Pts',(-18.8132087687919,0.788473960121406,
-1.54094231044465));
#63422=CARTESIAN_POINT('Ctrl Pts',(-18.7336651415749,1.72260046957501,-0.169829361795908));
#63423=CARTESIAN_POINT('Ctrl Pts',(-18.6541215143578,1.07420884447249,1.35730237912011));
#63424=CARTESIAN_POINT('Ctrl Pts',(-18.5745778871408,-0.561036672001411,
1.63750793664569));
#63425=CARTESIAN_POINT('Ctrl Pts',(-18.4950342599237,-1.68086917003333,
0.413368144804963));
#63426=CARTESIAN_POINT('Ctrl Pts',(-18.4154906327066,-1.25652123251115,
-1.19052458276035));
#63427=CARTESIAN_POINT('Ctrl Pts',(-18.3359470054896,0.32216729182992,-1.70070650789106));
#63428=CARTESIAN_POINT('Ctrl Pts',(-18.2564033782725,1.60488725544752,-0.648483837277519));
#63429=CARTESIAN_POINT('Ctrl Pts',(-18.1768597510555,1.41322982829946,0.999487789976802));
#63430=CARTESIAN_POINT('Ctrl Pts',(-18.0973161238384,-0.076733196159435,
1.72925024404081));
#63431=CARTESIAN_POINT('Ctrl Pts',(-18.0177724966213,-1.49620298867657,
0.870385550536859));
#63432=CARTESIAN_POINT('Ctrl Pts',(-17.9382288694043,-1.5411414232974,-0.788084705666147));
#63433=CARTESIAN_POINT('Ctrl Pts',(-17.8586852421872,-0.170264471030831,
-1.72255751712755));
#63434=CARTESIAN_POINT('Ctrl Pts',(-17.7791416149702,1.35703099953753,-1.07455165357568));
#63435=CARTESIAN_POINT('Ctrl Pts',(-17.6995979877531,1.63764959763715,0.560623033122007));
#63436=CARTESIAN_POINT('Ctrl Pts',(-17.6200543605361,0.413792705289065,
1.68076470303181));
#63437=CARTESIAN_POINT('Ctrl Pts',(-17.540510733319,-1.19020715789459,1.25682190910428));
#63438=CARTESIAN_POINT('Ctrl Pts',(-17.460967106102,-1.70078783043366,-0.321737697133566));
#63439=CARTESIAN_POINT('Ctrl Pts',(-17.3814234788849,-0.648889197856976,
-1.60472340258768));
#63440=CARTESIAN_POINT('Ctrl Pts',(-17.3018798516678,0.999130787908217,
-1.41348224557719));
#63441=CARTESIAN_POINT('Ctrl Pts',(-17.2223362244507,1.72926957104715,0.0762963993807335));
#63442=CARTESIAN_POINT('Ctrl Pts',(-17.1427925972337,0.870763451289146,
1.49598308874367));
#63443=CARTESIAN_POINT('Ctrl Pts',(-17.0632489700166,-0.787695400929053,
1.54134043782133));
#63444=CARTESIAN_POINT('Ctrl Pts',(-16.9837053427996,-1.72251445477646,
0.170699569402452));
#63445=CARTESIAN_POINT('Ctrl Pts',(-16.9041617155825,-1.07489439411967,
-1.35675953337286));
#63446=CARTESIAN_POINT('Ctrl Pts',(-16.8246180883654,0.560209358473387,
-1.63779115414233));
#63447=CARTESIAN_POINT('Ctrl Pts',(-16.7450744611484,1.68066012879314,-0.41421723937211));
#63448=CARTESIAN_POINT('Ctrl Pts',(-16.6655308339313,1.25712250550892,1.18988965709052));
#63449=CARTESIAN_POINT('Ctrl Pts',(-16.5859872067143,-0.321308081909528,
1.70086904446158));
#63450=CARTESIAN_POINT('Ctrl Pts',(-16.5064435794972,-1.60455944734232,
0.649294517035638));
#63451=CARTESIAN_POINT('Ctrl Pts',(-16.4268999522802,-1.41373457267109,
-0.998773722092515));
#63452=CARTESIAN_POINT('Ctrl Pts',(-16.3473563250631,0.0758595977341116,
-1.7292887877216));
#63453=CARTESIAN_POINT('Ctrl Pts',(-16.267812697846,1.49576309336319,-0.871141296484464));
#63454=CARTESIAN_POINT('Ctrl Pts',(-16.188269070629,1.54153935400376,0.787306045934945));
#63455=CARTESIAN_POINT('Ctrl Pts',(-16.1087254434119,0.171134656882987,
1.72247128252449));
#63456=CARTESIAN_POINT('Ctrl Pts',(-16.0291818161949,-1.35648798064341,
1.07523706608263));
#63457=CARTESIAN_POINT('Ctrl Pts',(-15.9496381889778,-1.63793260615219,
-0.559795648081974));
#63458=CARTESIAN_POINT('Ctrl Pts',(-15.8700945617607,-0.414641747027034,
-1.68055544732401));
#63459=CARTESIAN_POINT('Ctrl Pts',(-15.7905509345437,1.18957208036842,-1.25742302170589));
#63460=CARTESIAN_POINT('Ctrl Pts',(-15.7110073073266,1.70095014996966,0.320878446185189));
#63461=CARTESIAN_POINT('Ctrl Pts',(-15.6314636801096,0.649699794787615,
1.60439538972193));
#63462=CARTESIAN_POINT('Ctrl Pts',(-15.5519200528925,-0.998416592552452,
1.41398680956506));
#63463=CARTESIAN_POINT('Ctrl Pts',(-15.4723764256755,-1.72930789406296,
-0.0754227912474636));
#63464=CARTESIAN_POINT('Ctrl Pts',(-15.3928327984584,-0.871519086098719,
-1.49554300254914));
#63465=CARTESIAN_POINT('Ctrl Pts',(-15.3132891712414,0.786916640708664,
-1.54173817183197));
#63466=CARTESIAN_POINT('Ctrl Pts',(-15.2337455440242,1.72242800037439,-0.171569733444734));
#63467=CARTESIAN_POINT('Ctrl Pts',(-15.1542019168073,1.07557966944271,1.35621634136652));
#63468=CARTESIAN_POINT('Ctrl Pts',(-15.0746582895901,-0.559381901974127,
1.63807395365773));
#63469=CARTESIAN_POINT('Ctrl Pts',(-14.9951146623731,-1.68045065863108,
0.41506622822674));
#63470=CARTESIAN_POINT('Ctrl Pts',(-14.915571035156,-1.25772345767604,-1.18925442774851));
#63471=CARTESIAN_POINT('Ctrl Pts',(-14.836027407939,0.320448789987955,-1.70103114695273));
#63472=CARTESIAN_POINT('Ctrl Pts',(-14.7564837807219,1.60423122973695,-0.65010503108709));
#63473=CARTESIAN_POINT('Ctrl Pts',(-14.6769401535048,1.41423895624302,0.998059399310818));
#63474=CARTESIAN_POINT('Ctrl Pts',(-14.5973965262878,-0.0749859799485997,
1.72932689006999));
#63475=CARTESIAN_POINT('Ctrl Pts',(-14.5178528990708,-1.49532281631557,
0.871896820107827));
#63476=CARTESIAN_POINT('Ctrl Pts',(-14.4383092718537,-1.54193689129333,
-0.786527185275081));
#63477=CARTESIAN_POINT('Ctrl Pts',(-14.3587656446366,-0.172004799059819,
-1.72238460832893));
#63478=CARTESIAN_POINT('Ctrl Pts',(-14.2792220174195,1.3559446155595,-1.07592220417798));
#63479=CARTESIAN_POINT('Ctrl Pts',(-14.1996783902025,1.6382151966499,0.558968120176268));
#63480=CARTESIAN_POINT('Ctrl Pts',(-14.1201347629854,0.415490682944149,
1.68034576272107));
#63481=CARTESIAN_POINT('Ctrl Pts',(-14.0405911357684,-1.18893669925114,
1.25802381340014));
#63482=CARTESIAN_POINT('Ctrl Pts',(-13.9610475085513,-1.70111203540558,
-0.320019113345276));
#63483=CARTESIAN_POINT('Ctrl Pts',(-13.8815038813343,-0.650510225908176,
-1.60406696739786));
#63484=CARTESIAN_POINT('Ctrl Pts',(-13.8019602541172,0.99770214239043,-1.41449101268888));
#63485=CARTESIAN_POINT('Ctrl Pts',(-13.7224166269001,1.7293457757415,0.0745491638655046));
#63486=CARTESIAN_POINT('Ctrl Pts',(-13.6428729996831,0.872274498487625,
1.49510253467652));
#63487=CARTESIAN_POINT('Ctrl Pts',(-13.563329372466,-0.786137679659009,
1.5421355123751));
#63488=CARTESIAN_POINT('Ctrl Pts',(-13.4837857452489,-1.72234110639089,
0.172439853700588));
#63489=CARTESIAN_POINT('Ctrl Pts',(-13.4042421180319,-1.07626467026662,
-1.35567280323974));
#63490=CARTESIAN_POINT('Ctrl Pts',(-13.3246984908148,0.558554302714798,
-1.63835633511968));
#63491=CARTESIAN_POINT('Ctrl Pts',(-13.2451548635978,1.68024075960064,-0.415915111152186));
#63492=CARTESIAN_POINT('Ctrl Pts',(-13.1656112363807,1.25832408885909,1.18861889489651));
#63493=CARTESIAN_POINT('Ctrl Pts',(-13.0860676091637,-0.319589416284583,
1.70119281532309));
#63494=CARTESIAN_POINT('Ctrl Pts',(-13.0065239819466,-1.60390260271513,
0.650915379225009));
#63495=CARTESIAN_POINT('Ctrl Pts',(-12.9269803547296,-1.41474297888655,
-0.997344821814044));
#63496=CARTESIAN_POINT('Ctrl Pts',(-12.8474367275125,0.074112343025946,
-1.72936455107628));
#63497=CARTESIAN_POINT('Ctrl Pts',(-12.7678931002954,1.4948821576461,-0.872652121214035));
#63498=CARTESIAN_POINT('Ctrl Pts',(-12.6883494730784,1.54233403506462,0.785748123885319));
#63499=CARTESIAN_POINT('Ctrl Pts',(-12.6088058458613,0.172874897339258,
1.72229749456301));
#63500=CARTESIAN_POINT('Ctrl Pts',(-12.5292622186442,-1.35540090442454,
1.07660706768682));
#63501=CARTESIAN_POINT('Ctrl Pts',(-12.4497185914272,-1.63849736905809,
-0.558140449616154));
#63502=CARTESIAN_POINT('Ctrl Pts',(-12.3701749642101,-0.416339512823747,
-1.68013564927648));
#63503=CARTESIAN_POINT('Ctrl Pts',(-12.2906313369931,1.18830101470491,-1.2586242840337));
#63504=CARTESIAN_POINT('Ctrl Pts',(-12.211087709776,1.70127348670011,0.319159698833231));
#63505=CARTESIAN_POINT('Ctrl Pts',(-12.1315440825589,0.651320491011731,
1.60373813569929));
#63506=CARTESIAN_POINT('Ctrl Pts',(-12.0520004553419,-0.996987437604471,
1.41499485481993));
#63507=CARTESIAN_POINT('Ctrl Pts',(-11.9724568281248,-1.72938321607311,
-0.0736755174578175));
#63508=CARTESIAN_POINT('Ctrl Pts',(-11.8929132009078,-0.873029688263015,
-1.49466168523832));
#63509=CARTESIAN_POINT('Ctrl Pts',(-11.8133695736907,0.785358517978902,
-1.54253245934923));
#63510=CARTESIAN_POINT('Ctrl Pts',(-11.7338259464736,1.72225377284807,-0.173309929948049));
#63511=CARTESIAN_POINT('Ctrl Pts',(-11.6542823192566,1.0769493964167,1.35512891913123));
#63512=CARTESIAN_POINT('Ctrl Pts',(-11.5747386920395,-0.557726560906682,
1.63863829845615));
#63513=CARTESIAN_POINT('Ctrl Pts',(-11.4951950648225,-1.68003043175534,
0.41676388793174));
#63514=CARTESIAN_POINT('Ctrl Pts',(-11.4156514376054,-1.25892439890481,
-1.18798305869662));
#63515=CARTESIAN_POINT('Ctrl Pts',(-11.3361078103884,0.31872996101865,-1.70135404953147));
#63516=CARTESIAN_POINT('Ctrl Pts',(-11.2565641831713,1.60357356636082,-0.651725561242555));
#63517=CARTESIAN_POINT('Ctrl Pts',(-11.1770205559542,1.41524664047297,0.996629989784558));
#63518=CARTESIAN_POINT('Ctrl Pts',(-11.0974769287371,-0.073238687189009,
1.7294017707308));
#63519=CARTESIAN_POINT('Ctrl Pts',(-11.0179333015201,-1.49444111746723,
0.873407199610443));
#63520=CARTESIAN_POINT('Ctrl Pts',(-10.938389674303,-1.54273078521631,-0.784968861964558));
#63521=CARTESIAN_POINT('Ctrl Pts',(-10.858846047086,-0.173744951499187,
-1.7222099412489));
#63522=CARTESIAN_POINT('Ctrl Pts',(-10.7793024198689,1.35485684737718,-1.0772916564344));
#63523=CARTESIAN_POINT('Ctrl Pts',(-10.6997587926519,1.63877912330483,0.557312636612794));
#63524=CARTESIAN_POINT('Ctrl Pts',(-10.6202151654348,0.417188236449154,
1.67992510704391));
#63525=CARTESIAN_POINT('Ctrl Pts',(-10.5406715382178,-1.18766502689197,
1.25922443345327));
#63526=CARTESIAN_POINT('Ctrl Pts',(-10.4611279110007,-1.70143450381201,
-0.318300202868278));
#63527=CARTESIAN_POINT('Ctrl Pts',(-10.3815842837836,-0.652130589891605,
-1.60340889471017));
#63528=CARTESIAN_POINT('Ctrl Pts',(-10.3020406565666,0.996272478377053,
-1.41549833582965));
#63529=CARTESIAN_POINT('Ctrl Pts',(-10.2224970293495,1.7294202150482,0.0728018522474178));
#63530=CARTESIAN_POINT('Ctrl Pts',(-10.1429534021325,0.87378465523221,1.49422045434693));
#63531=CARTESIAN_POINT('Ctrl Pts',(-10.0634097749154,-0.784579155867149,
1.54292901265316));
#63532=CARTESIAN_POINT('Ctrl Pts',(-9.98386614769833,-1.7221659997683,0.17417996196498));
#63533=CARTESIAN_POINT('Ctrl Pts',(-9.90432252048128,-1.07763384771809,
-1.35458468917979));
#63534=CARTESIAN_POINT('Ctrl Pts',(-9.82477889326421,0.55689867676092,-1.63891984359515));
#63535=CARTESIAN_POINT('Ctrl Pts',(-9.74523526604717,1.6798196751489,-0.417612558348886));
#63536=CARTESIAN_POINT('Ctrl Pts',(-9.66569163883009,1.25952438765999,1.1873469193112));
#63537=CARTESIAN_POINT('Ctrl Pts',(-9.58614801161304,-0.317870424409565,
1.70151484953664));
#63538=CARTESIAN_POINT('Ctrl Pts',(-9.50660438439598,-1.60324412075788,
0.652535576933021));
#63539=CARTESIAN_POINT('Ctrl Pts',(-9.42706075717891,-1.41574994087386,
-0.995914903404769));
#63540=CARTESIAN_POINT('Ctrl Pts',(-9.34751712996185,0.072365012660848,
-1.72943854902412));
#63541=CARTESIAN_POINT('Ctrl Pts',(-9.26797350274479,1.49399969589152,-0.874162055104235));
#63542=CARTESIAN_POINT('Ctrl Pts',(-9.18842987552774,1.54312714164713,0.784189399711559));
#63543=CARTESIAN_POINT('Ctrl Pts',(-9.10888624831068,0.17461496131765,1.72212194840903));
#63544=CARTESIAN_POINT('Ctrl Pts',(-9.02934262109362,-1.35431244455638,
1.07797597024599));
#63545=CARTESIAN_POINT('Ctrl Pts',(-8.94979899387657,-1.63906045931814,
-0.556484681377506));
#63546=CARTESIAN_POINT('Ctrl Pts',(-8.87025536665949,-0.41803685360384,
-1.67971413607703));
#63547=CARTESIAN_POINT('Ctrl Pts',(-8.79071173944245,1.18702873597461,-1.25982426150579));
#63548=CARTESIAN_POINT('Ctrl Pts',(-8.71116811222537,1.70159508670024,0.317440625669869));
#63549=CARTESIAN_POINT('Ctrl Pts',(-8.63162448500832,0.652940522340951,
1.60307924451448));
#63550=CARTESIAN_POINT('Ctrl Pts',(-8.55208085779126,-0.99555726489053,
1.41600145558954));
#63551=CARTESIAN_POINT('Ctrl Pts',(-8.47253723057421,-1.72945677265738,
-0.0719281684571926));
#63552=CARTESIAN_POINT('Ctrl Pts',(-8.39299360335713,-0.874539399202495,
-1.49377884211506));
#63553=CARTESIAN_POINT('Ctrl Pts',(-8.31344997614009,0.783799593522696,
-1.54332517218559));
#63554=CARTESIAN_POINT('Ctrl Pts',(-8.23390634892302,1.7220777871739,-0.175049949529422));
#63555=CARTESIAN_POINT('Ctrl Pts',(-8.15436272170597,1.07831802399623,1.35404011352432));
#63556=CARTESIAN_POINT('Ctrl Pts',(-8.07481909448889,-0.556070650488905,
1.63920097046485));
#63557=CARTESIAN_POINT('Ctrl Pts',(-7.99527546727185,-1.67960848983507,
0.418461122186932));
#63558=CARTESIAN_POINT('Ctrl Pts',(-7.91573184005478,-1.26012405497151,
-1.1867104769025));
#63559=CARTESIAN_POINT('Ctrl Pts',(-7.83618821283773,0.317010806676624,
-1.70167521529765));
#63560=CARTESIAN_POINT('Ctrl Pts',(-7.75664458562067,1.60291426599049,-0.653345426089623));
#63561=CARTESIAN_POINT('Ctrl Pts',(-7.67710095840361,1.41625287996065,0.9951995628572));
#63562=CARTESIAN_POINT('Ctrl Pts',(-7.59755733118654,-0.0714913196643404,
1.72947488594679));
#63563=CARTESIAN_POINT('Ctrl Pts',(-7.5180137039695,-1.49355789303162,0.874916687502879));
#63564=CARTESIAN_POINT('Ctrl Pts',(-7.43847007675241,-1.54352310425593,
-0.783409737325367));
#63565=CARTESIAN_POINT('Ctrl Pts',(-7.35892644953538,-0.175484926572522,
-1.72203351606577));
#63566=CARTESIAN_POINT('Ctrl Pts',(-7.27938282231829,1.35376769610098,-1.07866000894696));
#63567=CARTESIAN_POINT('Ctrl Pts',(-7.19983919510126,1.63934137702629,0.555656584121541));
#63568=CARTESIAN_POINT('Ctrl Pts',(-7.12029556788418,0.418885364071158,
1.67950273642976));
#63569=CARTESIAN_POINT('Ctrl Pts',(-7.04075194066713,-1.18639214211523,
1.26042376803805));
#63570=CARTESIAN_POINT('Ctrl Pts',(-6.96120831345007,-1.70175523532376,
-0.316580967457275));
#63571=CARTESIAN_POINT('Ctrl Pts',(-6.88166468623301,-0.65375028815317,
-1.6027491851964));
#63572=CARTESIAN_POINT('Ctrl Pts',(-6.80212105901595,0.994841797327544,
-1.4165042139712));
#63573=CARTESIAN_POINT('Ctrl Pts',(-6.72257743179888,1.72949288889124,0.0710544663101945));
#63574=CARTESIAN_POINT('Ctrl Pts',(-6.64303380458183,0.875293919981295,
1.49333684865531));
#63575=CARTESIAN_POINT('Ctrl Pts',(-6.56349017736477,-0.78301983114445,
1.5437209378455));
#63576=CARTESIAN_POINT('Ctrl Pts',(-6.48394655014771,-1.72198913508746,
0.175919892419264));
#63577=CARTESIAN_POINT('Ctrl Pts',(-6.40440292293067,-1.07900192507638,
-1.35349519230379));
#63578=CARTESIAN_POINT('Ctrl Pts',(-6.32485929571358,0.555242482301849,
-1.63948167899348));
#63579=CARTESIAN_POINT('Ctrl Pts',(-6.24531566849655,1.6793968758678,-0.41930957922942));
#63580=CARTESIAN_POINT('Ctrl Pts',(-6.16577204127946,1.26072340068632,1.18607373163306));
#63581=CARTESIAN_POINT('Ctrl Pts',(-6.08622841406243,-0.316151108039277,
1.70183514677349));
#63582=CARTESIAN_POINT('Ctrl Pts',(-6.00668478684534,-1.60258400214274,
0.654155108505738));
#63583=CARTESIAN_POINT('Ctrl Pts',(-5.9271411596283,-1.41675545760511,-0.994483968324387));
#63584=CARTESIAN_POINT('Ctrl Pts',(-5.84759753241123,0.0706176084225559,
-1.72951078148959));
#63585=CARTESIAN_POINT('Ctrl Pts',(-5.76805390519418,1.49311570900028,-0.875671096613672));
#63586=CARTESIAN_POINT('Ctrl Pts',(-5.68851027797711,1.54391867294165,0.782629875004844));
#63587=CARTESIAN_POINT('Ctrl Pts',(-5.60896665076006,0.176354847041871,
1.72194464424177));
#63588=CARTESIAN_POINT('Ctrl Pts',(-5.529423023543,-1.3532226021501,1.07934377236272));
#63589=CARTESIAN_POINT('Ctrl Pts',(-5.44987939632593,-1.63962187635751,
-0.554828345056291));
#63590=CARTESIAN_POINT('Ctrl Pts',(-5.37033576910888,-0.41973376763463,
-1.67929090815595));
#63591=CARTESIAN_POINT('Ctrl Pts',(-5.29079214189181,1.1857552454763,-1.26102295289718));
#63592=CARTESIAN_POINT('Ctrl Pts',(-5.21124851467476,1.70191494964176,0.315721228449992));
#63593=CARTESIAN_POINT('Ctrl Pts',(-5.13170488745769,0.654559887121492,
1.60241871684011));
#63594=CARTESIAN_POINT('Ctrl Pts',(-5.05216126024064,-0.994126075870575,
1.41700661084632));
#63595=CARTESIAN_POINT('Ctrl Pts',(-4.97261763302358,-1.72952856374066,
-0.0701807460293178));
#63596=CARTESIAN_POINT('Ctrl Pts',(-4.89307400580652,-0.876048217376002,
-1.4928944740806));
#63597=CARTESIAN_POINT('Ctrl Pts',(-4.81353037858946,0.78223986893146,-1.5441163095318));
#63598=CARTESIAN_POINT('Ctrl Pts',(-4.7339867513724,1.72190004353153,-0.17678979041257));
#63599=CARTESIAN_POINT('Ctrl Pts',(-4.65444312415534,1.07968555078413,1.35294992565728));
#63600=CARTESIAN_POINT('Ctrl Pts',(-4.57489949693828,-0.554414172411219,
1.63976196910943));
#63601=CARTESIAN_POINT('Ctrl Pts',(-4.49535586972122,-1.67918483330103,
0.420157929259712));
#63602=CARTESIAN_POINT('Ctrl Pts',(-4.41581224250417,-1.26132242465148,
-1.18543668366527));
#63603=CARTESIAN_POINT('Ctrl Pts',(-4.3362686152871,0.315291328716861,-1.70199464392343));
#63604=CARTESIAN_POINT('Ctrl Pts',(-4.25672498807005,1.60225332929902,-0.654964623974668));
#63605=CARTESIAN_POINT('Ctrl Pts',(-4.17718136085298,1.41725767367884,0.993768119988983));
#63606=CARTESIAN_POINT('Ctrl Pts',(-4.09763773363593,-0.0697438791584081,
1.72954623564333));
#63607=CARTESIAN_POINT('Ctrl Pts',(-4.01809410641886,-1.49267314391039,
0.876425282244154));
#63608=CARTESIAN_POINT('Ctrl Pts',(-3.93855047920181,-1.54431384760333,
-0.781849812949146));
#63609=CARTESIAN_POINT('Ctrl Pts',(-3.85900685198474,-0.177224722503594,
-1.72185533295964));
#63610=CARTESIAN_POINT('Ctrl Pts',(-3.77946322476768,1.35267716284278,-1.08002726031877));
#63611=CARTESIAN_POINT('Ctrl Pts',(-3.69991959755063,1.63990195724028,0.553999964393108));
#63612=CARTESIAN_POINT('Ctrl Pts',(-3.62037597033356,0.420582064077634,
1.67907865130977));
#63613=CARTESIAN_POINT('Ctrl Pts',(-3.54083234311651,-1.18511804622036,
1.26162181593013));
#63614=CARTESIAN_POINT('Ctrl Pts',(-3.46128871589944,-1.70207422961342,
-0.314861408867349));
#63615=CARTESIAN_POINT('Ctrl Pts',(-3.38174508868239,-0.655369319039388,
-1.60208783953004));
#63616=CARTESIAN_POINT('Ctrl Pts',(-3.30220146146532,0.99341010070244,-1.4175086460866));
#63617=CARTESIAN_POINT('Ctrl Pts',(-3.22265783424827,1.7295637971964,0.0693070078375217));
#63618=CARTESIAN_POINT('Ctrl Pts',(-3.1431142070312,0.87680229119424,1.49245171850394));
#63619=CARTESIAN_POINT('Ctrl Pts',(-3.06357057981415,-0.781459707082962,
1.54451128714328));
#63620=CARTESIAN_POINT('Ctrl Pts',(-2.98402695259708,-1.72181051252855,
0.177659643287937));
#63621=CARTESIAN_POINT('Ctrl Pts',(-2.90448332538003,-1.08036890094558,
-1.3524043137253));
#63622=CARTESIAN_POINT('Ctrl Pts',(-2.82493969816297,0.553585721029618,
-1.64004184073856));
#63623=CARTESIAN_POINT('Ctrl Pts',(-2.74539607094591,1.6789723621865,-0.421006172066271));
#63624=CARTESIAN_POINT('Ctrl Pts',(-2.66585244372885,1.26192112671868,1.18479933317116));
#63625=CARTESIAN_POINT('Ctrl Pts',(-2.58630881651179,-0.31443146893764,
1.70215370668898));
#63626=CARTESIAN_POINT('Ctrl Pts',(-2.50676518929473,-1.60192224752698,
0.655773972323425));
#63627=CARTESIAN_POINT('Ctrl Pts',(-2.42722156207767,-1.4177595280854,-0.993052018097407));
#63628=CARTESIAN_POINT('Ctrl Pts',(-2.34767793486061,0.068870132154922,
-1.729581248278));
#63629=CARTESIAN_POINT('Ctrl Pts',(-2.26813430764355,1.49223019776091,-0.877179244431392));
#63630=CARTESIAN_POINT('Ctrl Pts',(-2.1885906804265,1.54470862835635,0.781069551792904));
#63631=CARTESIAN_POINT('Ctrl Pts',(-2.10904705320943,0.178094552325416,
1.7217655814153));
#63632=CARTESIAN_POINT('Ctrl Pts',(-2.02950342599238,-1.35213137753944,
1.08071047421022));
#63633=CARTESIAN_POINT('Ctrl Pts',(-1.94995979877531,-1.64018162108127,
-0.553171445322414));
#63634=CARTESIAN_POINT('Ctrl Pts',(-1.87041617155825,-0.421430250378147,
-1.67886596029095));
#63635=CARTESIAN_POINT('Ctrl Pts',(-1.79087254434119,1.18448053918477,-1.2622203677164));
#63636=CARTESIAN_POINT('Ctrl Pts',(-1.71132891712414,1.70223308530569,0.314001529299059));
#63637=CARTESIAN_POINT('Ctrl Pts',(-1.63178528990707,0.656178564515644,
1.60175651468699));
#63638=CARTESIAN_POINT('Ctrl Pts',(-1.55224166269002,-0.992693835592505,
1.41801039294902));
#63639=CARTESIAN_POINT('Ctrl Pts',(-1.47269803547296,-1.72959865836334,
-0.0684333912455062));
#63640=CARTESIAN_POINT('Ctrl Pts',(-1.3931544082559,-0.877556010062709,
-1.49200831766453));
#63641=CARTESIAN_POINT('Ctrl Pts',(-1.31361078103884,0.780679096811435,
-1.54490637237138));
#63642=CARTESIAN_POINT('Ctrl Pts',(-1.23406715382177,1.72172101468799,-0.178528498401339));
#63643=CARTESIAN_POINT('Ctrl Pts',(-1.15452352660472,1.0810510783977,1.35185654891102));
#63644=CARTESIAN_POINT('Ctrl Pts',(-1.07497989938766,-0.552755425847358,
1.64032472496632));
#63645=CARTESIAN_POINT('Ctrl Pts',(-0.995436272170598,-1.67876269403335,
0.421847794956357));
#63646=CARTESIAN_POINT('Ctrl Pts',(-0.915892644953538,-1.26251337329806,
-1.18414931936237));
#63647=CARTESIAN_POINT('Ctrl Pts',(-0.83634901773648,0.313559887373977,
-1.70233579666472));
#63648=CARTESIAN_POINT('Ctrl Pts',(-0.756805390519419,1.60161285332412,
-0.656538621811975));
#63649=CARTESIAN_POINT('Ctrl Pts',(-0.677261763302361,1.4182190784154,0.992251136832745));
#63650=CARTESIAN_POINT('Ctrl Pts',(-0.597718136085304,-0.0679167392546382,
1.7297762814003));
#63651=CARTESIAN_POINT('Ctrl Pts',(-0.518174508868237,-1.49193817974258,
0.877628180633763));
#63652=CARTESIAN_POINT('Ctrl Pts',(-0.438630881651179,-1.54481437551655,
-0.779708542229249));
#63653=CARTESIAN_POINT('Ctrl Pts',(-0.35908725443412,-0.179524439481945,
-1.72279441023562));
#63654=CARTESIAN_POINT('Ctrl Pts',(-0.279543627217061,1.35275091771125,
-1.07912501192066));
#63655=CARTESIAN_POINT('Ctrl Pts',(-0.226514542405688,1.54259118067785,
0.00486583246666068));
#63656=CARTESIAN_POINT('Ctrl Pts',(-0.2,1.38699088616441,0.466999498604503));
#63657=CARTESIAN_POINT('Ctrl Pts',(-34.7464852262806,0.795408277542816,
-1.1132985828233));
#63658=CARTESIAN_POINT('Ctrl Pts',(-34.7199706838749,1.16634997638047,-0.848275252789927));
#63659=CARTESIAN_POINT('Ctrl Pts',(-34.6669415990635,1.61598272073042,0.0771399500791215));
#63660=CARTESIAN_POINT('Ctrl Pts',(-34.5873979718465,0.807203207862427,
1.40386844011039));
#63661=CARTESIAN_POINT('Ctrl Pts',(-34.5078543446295,-0.743798775234758,
1.43668761512983));
#63662=CARTESIAN_POINT('Ctrl Pts',(-34.4283107174123,-1.61114028601272,
0.151766127691824));
#63663=CARTESIAN_POINT('Ctrl Pts',(-34.3487670901953,-0.998542967122596,
-1.2736823619854));
#63664=CARTESIAN_POINT('Ctrl Pts',(-34.2692234629782,0.531491994271277,
-1.52844520038366));
#63665=CARTESIAN_POINT('Ctrl Pts',(-34.1896798357612,1.57320521418612,-0.379361554962864));
#63666=CARTESIAN_POINT('Ctrl Pts',(-34.1101362085441,1.16967346714324,1.11839460788198));
#63667=CARTESIAN_POINT('Ctrl Pts',(-34.0305925813271,-0.308427691545578,
1.58861962571467));
#63668=CARTESIAN_POINT('Ctrl Pts',(-33.95104895411,-1.50317514966669,0.599456613073146));
#63669=CARTESIAN_POINT('Ctrl Pts',(-33.8715053268929,-1.31698998259737,
-0.940438546788035));
#63670=CARTESIAN_POINT('Ctrl Pts',(-33.7919616996759,0.0790892493159759,
-1.61635949102604));
#63671=CARTESIAN_POINT('Ctrl Pts',(-33.7124180724588,1.40250970409232,-0.807370259483987));
#63672=CARTESIAN_POINT('Ctrl Pts',(-33.6328744452418,1.43747349502384,0.743337102075247));
#63673=CARTESIAN_POINT('Ctrl Pts',(-33.5533308180247,0.151859221733174,
1.61115392399698));
#63674=CARTESIAN_POINT('Ctrl Pts',(-33.4737871908077,-1.27326488144399,
0.998837248074543));
#63675=CARTESIAN_POINT('Ctrl Pts',(-33.3942435635906,-1.52866643066679,
-0.531091464157164));
#63676=CARTESIAN_POINT('Ctrl Pts',(-33.3146999363736,-0.379713071742401,
-1.57311694851546));
#63677=CARTESIAN_POINT('Ctrl Pts',(-33.2351563091565,1.11807496622028,-1.16995191866883));
#63678=CARTESIAN_POINT('Ctrl Pts',(-33.1556126819394,1.58871020816909,0.308024297645402));
#63679=CARTESIAN_POINT('Ctrl Pts',(-33.0760690547224,0.599829578327863,
1.50302479657768));
#63680=CARTESIAN_POINT('Ctrl Pts',(-32.9965254275053,-0.940102323271568,
1.31722690138216));
#63681=CARTESIAN_POINT('Ctrl Pts',(-32.9169818002883,-1.61638127799984,
-0.0786806588829465));
#63682=CARTESIAN_POINT('Ctrl Pts',(-32.8374381730712,-0.807723515481981,
-1.40230588701147));
#63683=CARTESIAN_POINT('Ctrl Pts',(-32.7578945458541,0.742973467782488,
-1.43766112424875));
#63684=CARTESIAN_POINT('Ctrl Pts',(-32.678350918637,1.61111578641328,-0.152266226232503));
#63685=CARTESIAN_POINT('Ctrl Pts',(-32.59880729142,0.999158688993503,1.27301256658237));
#63686=CARTESIAN_POINT('Ctrl Pts',(-32.5192636642029,-0.530705243141331,
1.52880051868043));
#63687=CARTESIAN_POINT('Ctrl Pts',(-32.4397200369859,-1.57302102575292,
0.380110422584496));
#63688=CARTESIAN_POINT('Ctrl Pts',(-32.3601764097688,-1.1702342768756,-1.11777941383975));
#63689=CARTESIAN_POINT('Ctrl Pts',(-32.2806327825518,0.307622981690703,
-1.58878796004738));
#63690=CARTESIAN_POINT('Ctrl Pts',(-32.2010891553347,1.50287324245315,-0.60020921180962));
#63691=CARTESIAN_POINT('Ctrl Pts',(-32.1215455281177,1.3174643183768,0.939769573152954));
#63692=CARTESIAN_POINT('Ctrl Pts',(-32.0420019009006,-0.0782723701948242,
1.61640110025169));
#63693=CARTESIAN_POINT('Ctrl Pts',(-31.9624582736835,-1.40210181883799,
0.808077700742095));
#63694=CARTESIAN_POINT('Ctrl Pts',(-31.8829146464664,-1.43784874689912,
-0.742610302827902));
#63695=CARTESIAN_POINT('Ctrl Pts',(-31.8033710192494,-0.152673176153759,
-1.61107727378611));
#63696=CARTESIAN_POINT('Ctrl Pts',(-31.7238273920323,1.27276014686275,-0.999480209600985));
#63697=CARTESIAN_POINT('Ctrl Pts',(-31.6442837648153,1.52893452160575,0.530319063836459));
#63698=CARTESIAN_POINT('Ctrl Pts',(-31.5647401375983,0.380507742613516,
1.57292496281214));
#63699=CARTESIAN_POINT('Ctrl Pts',(-31.4851965103811,-1.11748378668527,
1.1705165813955));
#63700=CARTESIAN_POINT('Ctrl Pts',(-31.4056528831641,-1.58886561237809,
-0.30722165716086));
#63701=CARTESIAN_POINT('Ctrl Pts',(-31.326109255947,-0.600588806036943,
-1.50272158661857));
#63702=CARTESIAN_POINT('Ctrl Pts',(-31.24656562873,0.939436762569066,-1.31770165438161));
#63703=CARTESIAN_POINT('Ctrl Pts',(-31.1670220015129,1.61642081963931,0.0778640781290166));
#63704=CARTESIAN_POINT('Ctrl Pts',(-31.0874783742959,0.808431834304442,
1.40189766035522));
#63705=CARTESIAN_POINT('Ctrl Pts',(-31.0079347470788,-0.742247090418913,
1.43803627825968));
#63706=CARTESIAN_POINT('Ctrl Pts',(-30.9283911198618,-1.61103865840699,
0.153080116097703));
#63707=CARTESIAN_POINT('Ctrl Pts',(-30.8488474926447,-0.999801666418527,
-1.27250764581319));
#63708=CARTESIAN_POINT('Ctrl Pts',(-30.7693038654276,0.529932850685034,
-1.52906842704672));
#63709=CARTESIAN_POINT('Ctrl Pts',(-30.6897602382106,1.57282879952036,-0.380905038330596));
#63710=CARTESIAN_POINT('Ctrl Pts',(-30.6102166109935,1.17079881123042,1.11718808821421));
#63711=CARTESIAN_POINT('Ctrl Pts',(-30.5306729837765,-0.306820313027887,
1.58894316334467));
#63712=CARTESIAN_POINT('Ctrl Pts',(-30.4511293565594,-1.50256983490729,
0.600968361940099));
#63713=CARTESIAN_POINT('Ctrl Pts',(-30.3715857293423,-1.31793890631321,
-0.939103892044016));
#63714=CARTESIAN_POINT('Ctrl Pts',(-30.2920421021253,0.0774557810950461,
-1.61644043589649));
#63715=CARTESIAN_POINT('Ctrl Pts',(-30.2124984749082,1.40169341242787,-0.808785916286005));
#63716=CARTESIAN_POINT('Ctrl Pts',(-30.1329548476912,1.43822371786973,0.741883830652245));
#63717=CARTESIAN_POINT('Ctrl Pts',(-30.0534112204741,0.153487046274775,
1.61099994023964));
#63718=CARTESIAN_POINT('Ctrl Pts',(-29.973867593257,-1.27225506357436,1.00012305944603));
#63719=CARTESIAN_POINT('Ctrl Pts',(-29.89432396604,-1.52920223492915,-0.529546603722463));
#63720=CARTESIAN_POINT('Ctrl Pts',(-29.8147803388229,-0.381302309744958,
-1.57273253587807));
#63721=CARTESIAN_POINT('Ctrl Pts',(-29.7352367116059,1.11689231846367,-1.17108096636533));
#63722=CARTESIAN_POINT('Ctrl Pts',(-29.6556930843888,1.58902061293255,0.306418949318976));
#63723=CARTESIAN_POINT('Ctrl Pts',(-29.5761494571718,0.601347879499918,
1.50241798732817));
#63724=CARTESIAN_POINT('Ctrl Pts',(-29.4966058299547,-0.938770961601707,
1.3181760741569));
#63725=CARTESIAN_POINT('Ctrl Pts',(-29.4170622027376,-1.6164599490206,-0.0770474791191996));
#63726=CARTESIAN_POINT('Ctrl Pts',(-29.3375185755206,-0.809139946664935,
-1.40148907506886));
#63727=CARTESIAN_POINT('Ctrl Pts',(-29.2579749483035,0.741520523551474,
-1.43841106571739));
#63728=CARTESIAN_POINT('Ctrl Pts',(-29.1784313210865,1.61096111928633,-0.153893966658978));
#63729=CARTESIAN_POINT('Ctrl Pts',(-29.0988876938694,1.00044438866308,1.27200240016237));
#63730=CARTESIAN_POINT('Ctrl Pts',(-29.0193440666523,-0.529160322973449,
1.52933594524451));
#63731=CARTESIAN_POINT('Ctrl Pts',(-28.9398004394353,-1.57263617189136,
0.38169955683124));
#63732=CARTESIAN_POINT('Ctrl Pts',(-28.8602568122182,-1.17136304678224,
-1.1165964774525));
#63733=CARTESIAN_POINT('Ctrl Pts',(-28.7807131850011,0.306017566059744,
-1.58909796113681));
#63734=CARTESIAN_POINT('Ctrl Pts',(-28.7011695577841,1.5022660438909,-0.601727358692185));
#63735=CARTESIAN_POINT('Ctrl Pts',(-28.621625930567,1.31841315789754,0.93843797126338));
#63736=CARTESIAN_POINT('Ctrl Pts',(-28.54208230335,-0.0766391722275201,
1.61647935901037));
#63737=CARTESIAN_POINT('Ctrl Pts',(-28.4625386761329,-1.40128464829121,
0.809493925418639));
#63738=CARTESIAN_POINT('Ctrl Pts',(-28.3829950489159,-1.4385983217907,-0.741157169139769));
#63739=CARTESIAN_POINT('Ctrl Pts',(-28.3034514216988,-0.154300877224343,
-1.61092219554952));
#63740=CARTESIAN_POINT('Ctrl Pts',(-28.2239077944817,1.27174965559333,-1.0007656540492));
#63741=CARTESIAN_POINT('Ctrl Pts',(-28.1443641672647,1.52946955798429,0.528774008462636));
#63742=CARTESIAN_POINT('Ctrl Pts',(-28.0648205400476,0.382096779564106,
1.5725397075664));
#63743=CARTESIAN_POINT('Ctrl Pts',(-27.9852769128305,-1.11630056519958,
1.17164505246315));
#63744=CARTESIAN_POINT('Ctrl Pts',(-27.9057332856135,-1.5891752079525,-0.305616163275796));
#63745=CARTESIAN_POINT('Ctrl Pts',(-27.8261896583964,-0.602106799492688,
-1.50211400460516));
#63746=CARTESIAN_POINT('Ctrl Pts',(-27.7466460311794,0.938104921050279,
-1.31865015752001));
#63747=CARTESIAN_POINT('Ctrl Pts',(-27.6671024039623,1.61649866586457,0.0762308604460643));
#63748=CARTESIAN_POINT('Ctrl Pts',(-27.5875587767452,0.809847852524537,
1.40108013210797));
#63749=CARTESIAN_POINT('Ctrl Pts',(-27.5080151495282,-0.74079376744032,
1.43878548607771));
#63750=CARTESIAN_POINT('Ctrl Pts',(-27.4284715223112,-1.61088316903171,
0.154707777944918));
#63751=CARTESIAN_POINT('Ctrl Pts',(-27.3489278950941,-1.00108685558388,
-1.27149682988338));
#63752=CARTESIAN_POINT('Ctrl Pts',(-27.269384267877,0.528387660214671,-1.52960307313994));
#63753=CARTESIAN_POINT('Ctrl Pts',(-27.18984064066,1.57244314290934,-0.382493977918206));
#63754=CARTESIAN_POINT('Ctrl Pts',(-27.1102970134429,1.17192698339008,1.1160045817238));
#63755=CARTESIAN_POINT('Ctrl Pts',(-27.0307533862258,-0.305214740992747,
1.5892523533747));
#63756=CARTESIAN_POINT('Ctrl Pts',(-26.9512097590088,-1.50196186948066,
0.602486201877221));
#63757=CARTESIAN_POINT('Ctrl Pts',(-26.8716661317917,-1.31888707300918,
-0.937771810983659));
#63758=CARTESIAN_POINT('Ctrl Pts',(-26.7921225045747,0.0758225438008824,
-1.61651786958198));
#63759=CARTESIAN_POINT('Ctrl Pts',(-26.7125788773576,1.40087552653219,-0.810201727960045));
#63760=CARTESIAN_POINT('Ctrl Pts',(-26.6330352501405,1.43897255856648,0.740430318476311));
#63761=CARTESIAN_POINT('Ctrl Pts',(-26.5534916229235,0.155114668794731,
1.61084403973538));
#63762=CARTESIAN_POINT('Ctrl Pts',(-26.4739479957064,-1.27124392304863,
1.00140799324662));
#63763=CARTESIAN_POINT('Ctrl Pts',(-26.3944043684894,-1.52973649070296,
-0.528001278254208));
#63764=CARTESIAN_POINT('Ctrl Pts',(-26.3148607412723,-0.382891151868202,
-1.57234647792633));
#63765=CARTESIAN_POINT('Ctrl Pts',(-26.2353171140552,1.11570852704404,-1.17220883954503));
#63766=CARTESIAN_POINT('Ctrl Pts',(-26.1557734868382,1.58932939739848,0.304813299236206));
#63767=CARTESIAN_POINT('Ctrl Pts',(-26.0762298596211,0.602865565821572,
1.50180963852711));
#63768=CARTESIAN_POINT('Ctrl Pts',(-25.9966862324041,-0.937438641084768,
1.31912390434994));
#63769=CARTESIAN_POINT('Ctrl Pts',(-25.917142605187,-1.61653697016136,-0.0754142223180269));
#63770=CARTESIAN_POINT('Ctrl Pts',(-25.8375989779699,-0.810555551702585,
-1.40067083157693));
#63771=CARTESIAN_POINT('Ctrl Pts',(-25.7580553507529,0.740066822270931,
-1.43915953924508));
#63772=CARTESIAN_POINT('Ctrl Pts',(-25.6785117235358,1.61080480766303,-0.15552154974783));
#63773=CARTESIAN_POINT('Ctrl Pts',(-25.5989680963188,1.00172906701694,1.27099093510523));
#63774=CARTESIAN_POINT('Ctrl Pts',(-25.5194244691017,-0.527614862605903,
1.52986981066483));
#63775=CARTESIAN_POINT('Ctrl Pts',(-25.4398808418846,-1.57224971262355,
0.383288301388741));
#63776=CARTESIAN_POINT('Ctrl Pts',(-25.3603372146676,-1.17249062091002,
-1.11541240117919));
#63777=CARTESIAN_POINT('Ctrl Pts',(-25.2807935874505,0.304411838031798,
-1.58940634001894));
#63778=CARTESIAN_POINT('Ctrl Pts',(-25.2012499602335,1.50165731175422,-0.603244891301526));
#63779=CARTESIAN_POINT('Ctrl Pts',(-25.1217063330164,1.31936065152718,0.93710541137487));
#63780=CARTESIAN_POINT('Ctrl Pts',(-25.0421627057994,-0.0750058960235608,
1.61655596760149));
#63781=CARTESIAN_POINT('Ctrl Pts',(-24.9626190785823,-1.40046604725525,
0.810909323729573));
#63782=CARTESIAN_POINT('Ctrl Pts',(-24.8830754513652,-1.43934642810156,
-0.739703278847383));
#63783=CARTESIAN_POINT('Ctrl Pts',(-24.8035318241482,-0.155928420778242,
-1.61076547281716));
#63784=CARTESIAN_POINT('Ctrl Pts',(-24.7239881969311,1.27073786606932,-1.00205007687434));
#63785=CARTESIAN_POINT('Ctrl Pts',(-24.6444445697141,1.53000303301705,0.527228413294394));
#63786=CARTESIAN_POINT('Ctrl Pts',(-24.564900942497,0.383685426454499,1.57215284700716));
#63787=CARTESIAN_POINT('Ctrl Pts',(-24.4853573152799,-1.11511620414815,
1.17277232746708));
#63788=CARTESIAN_POINT('Ctrl Pts',(-24.4058136880629,-1.58948318123115,
-0.304010357405141));
#63789=CARTESIAN_POINT('Ctrl Pts',(-24.3262700608458,-0.603624178292887,
-1.5015048891717));
#63790=CARTESIAN_POINT('Ctrl Pts',(-24.2467264336287,0.936772121875235,
-1.31959731452578));
#63791=CARTESIAN_POINT('Ctrl Pts',(-24.1671828064117,1.61657486190117,0.0745975649435363));
#63792=CARTESIAN_POINT('Ctrl Pts',(-24.0876391791946,0.811263044018437,
1.40026117358021));
#63793=CARTESIAN_POINT('Ctrl Pts',(-24.0080955519776,-0.739339688228858,
1.43953322512401));
#63794=CARTESIAN_POINT('Ctrl Pts',(-23.9285519247605,-1.61072603520029,
0.156335281860002));
#63795=CARTESIAN_POINT('Ctrl Pts',(-23.8490082975435,-1.00237102279835,
-1.27048471595706));
#63796=CARTESIAN_POINT('Ctrl Pts',(-23.7694646703264,0.526841930344371,
-1.5301361577511));
#63797=CARTESIAN_POINT('Ctrl Pts',(-23.6899210431094,1.57205588108336,-0.384082527040115));
#63798=CARTESIAN_POINT('Ctrl Pts',(-23.6103774158923,1.17305395919821,1.11481993596979));
#63799=CARTESIAN_POINT('Ctrl Pts',(-23.5308337886752,-0.303608857381817,
1.58955992103022));
#63800=CARTESIAN_POINT('Ctrl Pts',(-23.4512901614582,-1.50135237078928,
0.604003426771492));
#63801=CARTESIAN_POINT('Ctrl Pts',(-23.3717465342411,-1.31983389333067,
-0.9364387726071));
#63802=CARTESIAN_POINT('Ctrl Pts',(-23.292202907024,0.0741892291039624,
-1.61659365305919));
#63803=CARTESIAN_POINT('Ctrl Pts',(-23.212659279807,1.40005621056488,-0.811616712546633));
#63804=CARTESIAN_POINT('Ctrl Pts',(-23.1331156525899,1.43971993030053,0.738976050438524));
#63805=CARTESIAN_POINT('Ctrl Pts',(-23.0535720253729,0.156742132967183,
1.61068649481492));
#63806=CARTESIAN_POINT('Ctrl Pts',(-22.9740283981558,-1.27023148478456,
1.00269190476851));
#63807=CARTESIAN_POINT('Ctrl Pts',(-22.8944847709387,-1.53026918485852,
-0.526455413780454));
#63808=CARTESIAN_POINT('Ctrl Pts',(-22.8149411437217,-0.384479603120299,
-1.57195881485831));
#63809=CARTESIAN_POINT('Ctrl Pts',(-22.7353975165047,1.11452359666304,-1.17333551608548));
#63810=CARTESIAN_POINT('Ctrl Pts',(-22.6558538892875,1.58963655941125,0.303207337987452));
#63811=CARTESIAN_POINT('Ctrl Pts',(-22.5763102620705,0.6043826367131,1.50119975661669));
#63812=CARTESIAN_POINT('Ctrl Pts',(-22.4967666348534,-0.936105363591735,
1.32007038792675));
#63813=CARTESIAN_POINT('Ctrl Pts',(-22.4172230076364,-1.61661234107435,
-0.0737808885309362));
#63814=CARTESIAN_POINT('Ctrl Pts',(-22.3376793804193,-0.81197032929159,
-1.39985115822233));
#63815=CARTESIAN_POINT('Ctrl Pts',(-22.2581357532022,0.738612365499613,
-1.43990654361919));
#63816=CARTESIAN_POINT('Ctrl Pts',(-22.1785921259852,1.61064685166359,-0.157148974073823));
#63817=CARTESIAN_POINT('Ctrl Pts',(-22.0990484987681,1.00301272276432,1.26997817256801));
#63818=CARTESIAN_POINT('Ctrl Pts',(-22.0195048715511,-0.526068863627305,
1.5304021143308));
#63819=CARTESIAN_POINT('Ctrl Pts',(-21.939961244334,-1.57186164833823,0.384876654669678));
#63820=CARTESIAN_POINT('Ctrl Pts',(-21.860417617117,-1.1736169981109,-1.11422718624679));
#63821=CARTESIAN_POINT('Ctrl Pts',(-21.7808739898999,0.302805799247685,
-1.58971309636936));
#63822=CARTESIAN_POINT('Ctrl Pts',(-21.7013303626829,1.50104704666367,-0.604761808093543));
#63823=CARTESIAN_POINT('Ctrl Pts',(-21.6217867354658,1.32030679829891,0.935771894850433));
#63824=CARTESIAN_POINT('Ctrl Pts',(-21.5422431082487,-0.0733725432504879,
1.61663092594545));
#63825=CARTESIAN_POINT('Ctrl Pts',(-21.4626994810317,-1.39964601656566,
0.812323894230727));
#63826=CARTESIAN_POINT('Ctrl Pts',(-21.3831558538146,-1.44009306506808,
-0.738248633435309));
#63827=CARTESIAN_POINT('Ctrl Pts',(-21.3036122265975,-0.157555805153939,
-1.61060710574882));
#63828=CARTESIAN_POINT('Ctrl Pts',(-21.2240685993805,1.26972477932356,-1.00333347676534));
#63829=CARTESIAN_POINT('Ctrl Pts',(-21.1445249721634,1.53053494615945,0.525682279909613));
#63830=CARTESIAN_POINT('Ctrl Pts',(-21.0649813449464,0.385273681662942,
1.5717643815293));
#63831=CARTESIAN_POINT('Ctrl Pts',(-20.9854377177293,-1.11393070473997,
1.17389840525652));
#63832=CARTESIAN_POINT('Ctrl Pts',(-20.9058940905123,-1.58978953189966,
-0.302404241188112));
#63833=CARTESIAN_POINT('Ctrl Pts',(-20.8263504632952,-0.605140940888606,
-1.50089424093996));
#63834=CARTESIAN_POINT('Ctrl Pts',(-20.7468068360781,0.935438366404454,
-1.32054312443209));
#63835=CARTESIAN_POINT('Ctrl Pts',(-20.667263208861,1.61664940767132,0.0729641932886911));
#63836=CARTESIAN_POINT('Ctrl Pts',(-20.587719581644,0.81267740734151,1.39944078560794));
#63837=CARTESIAN_POINT('Ctrl Pts',(-20.5081759544269,-0.737884854268845,
1.44027949463531));
#63838=CARTESIAN_POINT('Ctrl Pts',(-20.4286323272099,-1.61056725707314,
0.1579626261816));
#63839=CARTESIAN_POINT('Ctrl Pts',(-20.3490886999928,-1.00365416675107,
-1.26947130506739));
#63840=CARTESIAN_POINT('Ctrl Pts',(-20.2695450727758,0.525295662652017,
-1.53066768033603));
#63841=CARTESIAN_POINT('Ctrl Pts',(-20.1900014455587,1.57166701443773,-0.385670684074736));
#63842=CARTESIAN_POINT('Ctrl Pts',(-20.1104578183417,1.17417973750438,1.11363415216148));
#63843=CARTESIAN_POINT('Ctrl Pts',(-20.0309141911245,-0.302002663834377,
1.58986586599726));
#63844=CARTESIAN_POINT('Ctrl Pts',(-19.9513705639076,-1.50074133945531,
0.605520035074122));
#63845=CARTESIAN_POINT('Ctrl Pts',(-19.8718269366905,-1.32077936631118,
-0.935104778275095));
#63846=CARTESIAN_POINT('Ctrl Pts',(-19.7922833094734,0.0725558386715783,
-1.61666778625077));
#63847=CARTESIAN_POINT('Ctrl Pts',(-19.7127396822564,1.39923546536229,-0.813030868601358));
#63848=CARTESIAN_POINT('Ctrl Pts',(-19.6331960550393,1.44046583230898,0.737521028023404));
#63849=CARTESIAN_POINT('Ctrl Pts',(-19.5536524278223,0.158369437130823,
1.61052730563911));
#63850=CARTESIAN_POINT('Ctrl Pts',(-19.4741088006052,-1.26921774981566,
1.00397479270108));
#63851=CARTESIAN_POINT('Ctrl Pts',(-19.3945651733881,-1.53080031685203,
-0.524909011879212));
#63852=CARTESIAN_POINT('Ctrl Pts',(-19.315021546171,-0.386067661879754,
-1.57156954706974));
#63853=CARTESIAN_POINT('Ctrl Pts',(-19.235477918954,1.11333752853026,-1.17446099483654));
#63854=CARTESIAN_POINT('Ctrl Pts',(-19.1559342917369,1.58994209865731,0.301601067212078));
#63855=CARTESIAN_POINT('Ctrl Pts',(-19.0763906645199,0.605899090625881,
1.50058834221949));
#63856=CARTESIAN_POINT('Ctrl Pts',(-18.9968470373028,-0.934771130483621,
1.32101552392115));
#63857=CARTESIAN_POINT('Ctrl Pts',(-18.9173034100858,-1.61668606168263,
-0.0721474794252276));
#63858=CARTESIAN_POINT('Ctrl Pts',(-18.8377597828687,-0.813384277987742,
-1.39903005584178));
#63859=CARTESIAN_POINT('Ctrl Pts',(-18.7582161556516,0.737157154722223,
-1.44065207807719));
#63860=CARTESIAN_POINT('Ctrl Pts',(-18.6786725284346,1.61048725144926,-0.158776237975679));
#63861=CARTESIAN_POINT('Ctrl Pts',(-18.5991289012175,1.00429535459488,1.26896411358455));
#63862=CARTESIAN_POINT('Ctrl Pts',(-18.5195852740004,-0.524522327615841,
1.53093285569902));
#63863=CARTESIAN_POINT('Ctrl Pts',(-18.4400416467834,-1.57147197943155,
0.386464615052644));
#63864=CARTESIAN_POINT('Ctrl Pts',(-18.3604980195664,-1.17474217723504,
-1.11304083386521));
#63865=CARTESIAN_POINT('Ctrl Pts',(-18.2809543923493,0.301199451346863,
-1.59001822987494));
#63866=CARTESIAN_POINT('Ctrl Pts',(-18.2014107651322,1.50043524924223,-0.60627810751972));
#63867=CARTESIAN_POINT('Ctrl Pts',(-18.1218671379152,1.32125159724689,0.934437423051337));
#63868=CARTESIAN_POINT('Ctrl Pts',(-18.0423235106981,-0.0717391155756687,
1.61670423396573));
#63869=CARTESIAN_POINT('Ctrl Pts',(-17.962779883481,-1.39882455705954,0.813737635478094));
#63870=CARTESIAN_POINT('Ctrl Pts',(-17.883236256264,-1.44083823192808,-0.736793234388497));
#63871=CARTESIAN_POINT('Ctrl Pts',(-17.8036926290469,-0.159183028690188,
-1.61044709450615));
#63872=CARTESIAN_POINT('Ctrl Pts',(-17.7241490018299,1.26871039639025,-1.00461585241206));
#63873=CARTESIAN_POINT('Ctrl Pts',(-17.6446053746128,1.53106529686852,0.524135609886599));
#63874=CARTESIAN_POINT('Ctrl Pts',(-17.5650617473957,0.386861543568101,
1.57137431152937));
#63875=CARTESIAN_POINT('Ctrl Pts',(-17.4855181201787,-1.11274406818528,
1.17502328468195));
#63876=CARTESIAN_POINT('Ctrl Pts',(-17.4059744929616,-1.59009425964529,
-0.300797816264331));
#63877=CARTESIAN_POINT('Ctrl Pts',(-17.3264308657446,-0.606657085731434,
-1.50028206053333));
#63878=CARTESIAN_POINT('Ctrl Pts',(-17.2468872385275,0.934103655999516,
-1.32148758627337));
#63879=CARTESIAN_POINT('Ctrl Pts',(-17.1673436113105,1.61672230309892,0.0713307471489807));
#63880=CARTESIAN_POINT('Ctrl Pts',(-17.0877999840934,0.814090941049888,
1.39861896902866));
#63881=CARTESIAN_POINT('Ctrl Pts',(-17.0082563568763,-0.736429267045466,
1.44102429384975));
#63882=CARTESIAN_POINT('Ctrl Pts',(-16.9287127296593,-1.61040683481235,
0.159589809248418));
#63883=CARTESIAN_POINT('Ctrl Pts',(-16.8491691024422,-1.00493628613213,
-1.26845659824893));
#63884=CARTESIAN_POINT('Ctrl Pts',(-16.7696254752251,0.523748858716137,
-1.5311976403521));
#63885=CARTESIAN_POINT('Ctrl Pts',(-16.6900818480081,1.57127654336944,-0.38725844740078));
#63886=CARTESIAN_POINT('Ctrl Pts',(-16.610538220791,1.17530431715934,1.11244723150939));
#63887=CARTESIAN_POINT('Ctrl Pts',(-16.530994593574,-0.300396161990134,
1.5901701879635));
#63888=CARTESIAN_POINT('Ctrl Pts',(-16.4514509663569,-1.50012877610254,
0.607036025236869));
#63889=CARTESIAN_POINT('Ctrl Pts',(-16.3719073391398,-1.32172349098552,
-0.933769829349476));
#63890=CARTESIAN_POINT('Ctrl Pts',(-16.2923637119228,0.0709223741711957,
-1.61674026908103));
#63891=CARTESIAN_POINT('Ctrl Pts',(-16.2128200847057,1.39841329176228,-0.814444194680562));
#63892=CARTESIAN_POINT('Ctrl Pts',(-16.1332764574887,1.44121026383035,0.73606525271633));
#63893=CARTESIAN_POINT('Ctrl Pts',(-16.0537328302716,0.159996579624394,
1.61036647237043));
#63894=CARTESIAN_POINT('Ctrl Pts',(-15.9741892030546,-1.26820271917681,
1.00525665573467));
#63895=CARTESIAN_POINT('Ctrl Pts',(-15.8946455758375,-1.5313298861413,-0.523362074129152));
#63896=CARTESIAN_POINT('Ctrl Pts',(-15.8151019486205,-0.387655326525378,
-1.57117867495801));
#63897=CARTESIAN_POINT('Ctrl Pts',(-15.7355583214034,1.1121503238565,-1.17558527464926));
#63898=CARTESIAN_POINT('Ctrl Pts',(-15.6560146941863,1.59024601482475,0.299994488549867));
#63899=CARTESIAN_POINT('Ctrl Pts',(-15.5764710669692,0.60741492601182,1.49997539595966));
#63900=CARTESIAN_POINT('Ctrl Pts',(-15.4969274397522,-0.93343594312249,
1.32195931136829));
#63901=CARTESIAN_POINT('Ctrl Pts',(-15.4173838125351,-1.61675813191094,
-0.0705139966683875));
#63902=CARTESIAN_POINT('Ctrl Pts',(-15.3378401853181,-0.814797396347597,
-1.39820752527351));
#63903=CARTESIAN_POINT('Ctrl Pts',(-15.258296558101,0.73570119142432,-1.44139614185799));
#63904=CARTESIAN_POINT('Ctrl Pts',(-15.178752930884,1.61032600718294,-0.16040333979222));
#63905=CARTESIAN_POINT('Ctrl Pts',(-15.0992093036669,1.00557696119926,1.26794875919005));
#63906=CARTESIAN_POINT('Ctrl Pts',(-15.0196656764498,-0.522975256150292,
1.5314620342277));
#63907=CARTESIAN_POINT('Ctrl Pts',(-14.9401220492328,-1.57108070630129,
0.388052180916562));
#63908=CARTESIAN_POINT('Ctrl Pts',(-14.8605784220157,-1.17586615713382,
-1.1118533452455));
#63909=CARTESIAN_POINT('Ctrl Pts',(-14.7810347947987,0.299592795969159,
-1.59032174022419));
#63910=CARTESIAN_POINT('Ctrl Pts',(-14.7014911675816,1.49982192011447,-0.607793788032152));
#63911=CARTESIAN_POINT('Ctrl Pts',(-14.6219475403645,1.32219504740662,0.93310199733987));
#63912=CARTESIAN_POINT('Ctrl Pts',(-14.5424039131475,-0.0701056146665614,
1.61677589158748));
#63913=CARTESIAN_POINT('Ctrl Pts',(-14.4628602859304,-1.39800166957547,
0.815150546028472));
#63914=CARTESIAN_POINT('Ctrl Pts',(-14.3833166587134,-1.44158192792085,
-0.735337083192683));
#63915=CARTESIAN_POINT('Ctrl Pts',(-14.3037730314963,-0.160810089725831,
-1.61028543925251));
#63916=CARTESIAN_POINT('Ctrl Pts',(-14.2242294042792,1.26769471830488,-1.0058972025054));
#63917=CARTESIAN_POINT('Ctrl Pts',(-14.1446857770622,1.53159408460286,0.522588404804257));
#63918=CARTESIAN_POINT('Ctrl Pts',(-14.0651421498451,0.388449010549016,
1.57098263740558));
#63919=CARTESIAN_POINT('Ctrl Pts',(-13.9855985226281,-1.11155629569543,
1.17614696459504));
#63920=CARTESIAN_POINT('Ctrl Pts',(-13.906054895411,-1.59039736415696,-0.299191084273672));
#63921=CARTESIAN_POINT('Ctrl Pts',(-13.8265112681939,-0.608172611273664,
-1.49966834857674));
#63922=CARTESIAN_POINT('Ctrl Pts',(-13.7469676409769,0.932767992022944,
-1.32243069908551));
#63923=CARTESIAN_POINT('Ctrl Pts',(-13.6674240137598,1.61679354810954,0.0696972281918805));
#63924=CARTESIAN_POINT('Ctrl Pts',(-13.5878803865428,0.815503643700602,
1.3977957246813));
#63925=CARTESIAN_POINT('Ctrl Pts',(-13.5083367593257,-0.734972928044621,
1.44176762200704));
#63926=CARTESIAN_POINT('Ctrl Pts',(-13.4287931321086,-1.6102447685817,0.161216829399376));
#63927=CARTESIAN_POINT('Ctrl Pts',(-13.3492495048916,-1.00621737963268,
-1.26744059653753));
#63928=CARTESIAN_POINT('Ctrl Pts',(-13.2697058776745,0.522201520115732,
-1.53172603725832));
#63929=CARTESIAN_POINT('Ctrl Pts',(-13.1901622504575,1.5708844682771,-0.388845815397424));
#63930=CARTESIAN_POINT('Ctrl Pts',(-13.1106186232404,1.17642769701507,1.11125917522517));
#63931=CARTESIAN_POINT('Ctrl Pts',(-13.0310749960234,-0.298789353489053,
1.59047288661827));
#63932=CARTESIAN_POINT('Ctrl Pts',(-12.9515313688063,-1.49951468135628,
0.608551395712171));
#63933=CARTESIAN_POINT('Ctrl Pts',(-12.8719877415893,-1.32266626638989,
-0.932433927192988));
#63934=CARTESIAN_POINT('Ctrl Pts',(-12.7924441143722,0.0692888372703077,
-1.616811101476));
#63935=CARTESIAN_POINT('Ctrl Pts',(-12.7129004871551,1.39758969060416,-0.815856689341468));
#63936=CARTESIAN_POINT('Ctrl Pts',(-12.633356859938,1.44195322410471,0.734608726003382));
#63937=CARTESIAN_POINT('Ctrl Pts',(-12.553813232721,0.161623558786877,1.61020399517309));
#63938=CARTESIAN_POINT('Ctrl Pts',(-12.4742696055039,-1.26718639390419,
1.00653749256072));
#63939=CARTESIAN_POINT('Ctrl Pts',(-12.3947259782869,-1.53185789218571,
-0.521814602109434));
#63940=CARTESIAN_POINT('Ctrl Pts',(-12.3151823510698,-0.389242595436448,
-1.57078619892211));
#63941=CARTESIAN_POINT('Ctrl Pts',(-12.2356387238528,1.11096198385369,-1.17670835437596));
#63942=CARTESIAN_POINT('Ctrl Pts',(-12.1560950966357,1.59054830760332,0.298387603640872));
#63943=CARTESIAN_POINT('Ctrl Pts',(-12.0765514694187,0.608930141323501,
1.49936091846293));
#63944=CARTESIAN_POINT('Ctrl Pts',(-11.9970078422015,-0.93209980287133,
1.32290174930472));
#63945=CARTESIAN_POINT('Ctrl Pts',(-11.9174642149845,-1.61682855168572,
-0.0688804419279146));
#63946=CARTESIAN_POINT('Ctrl Pts',(-11.8379205877674,-0.816209682928599,
-1.39738356735719));
#63947=CARTESIAN_POINT('Ctrl Pts',(-11.7583769605504,0.734244477092241,
-1.44213873420202));
#63948=CARTESIAN_POINT('Ctrl Pts',(-11.6788333333333,1.61016311902928,-0.162030277862366));
#63949=CARTESIAN_POINT('Ctrl Pts',(-11.5992897061163,1.00685754126906,1.26693211042105));
#63950=CARTESIAN_POINT('Ctrl Pts',(-11.5197460788992,-0.52142765080999,
1.53198964937662));
#63951=CARTESIAN_POINT('Ctrl Pts',(-11.4402024516822,-1.57068782934691,
0.389639350640762));
#63952=CARTESIAN_POINT('Ctrl Pts',(-11.3606588244651,-1.1769889366598,-1.11066472159995));
#63953=CARTESIAN_POINT('Ctrl Pts',(-11.2811151972481,0.297985834754776,
-1.59062362710725));
#63954=CARTESIAN_POINT('Ctrl Pts',(-11.201571570031,1.49920705990647,-0.609308848083547));
#63955=CARTESIAN_POINT('Ctrl Pts',(-11.1220279428139,1.32313714781499,0.931765619079327));
#63956=CARTESIAN_POINT('Ctrl Pts',(-11.0424843155969,-0.06847204219078,
1.61684589873756));
#63957=CARTESIAN_POINT('Ctrl Pts',(-10.9629406883798,-1.39717735495351,
0.816562624439442));
#63958=CARTESIAN_POINT('Ctrl Pts',(-10.8833970611627,-1.44232415228718,
-0.733880181334382));
#63959=CARTESIAN_POINT('Ctrl Pts',(-10.8038534339457,-0.162436986599875,
-1.61012214015292));
#63960=CARTESIAN_POINT('Ctrl Pts',(-10.7243098067286,1.26667774610436,-1.00717752573727));
#63961=CARTESIAN_POINT('Ctrl Pts',(-10.6447661795116,1.53212130882261,0.521040666242096));
#63962=CARTESIAN_POINT('Ctrl Pts',(-10.5652225522945,0.390036080985107,
1.57058935955777));
#63963=CARTESIAN_POINT('Ctrl Pts',(-10.4856789250774,-1.11036738848296,
1.17726944384868));
#63964=CARTESIAN_POINT('Ctrl Pts',(-10.4061352978604,-1.59069884512526,
-0.297584046856419));
#63965=CARTESIAN_POINT('Ctrl Pts',(-10.3265916706433,-0.609687515968113,
-1.49905310569671));
#63966=CARTESIAN_POINT('Ctrl Pts',(-10.2470480434263,0.931431375838247,
-1.32337246190571));
#63967=CARTESIAN_POINT('Ctrl Pts',(-10.1675044162092,1.61686314263048,0.0680636380849846));
#63968=CARTESIAN_POINT('Ctrl Pts',(-10.0879607889922,0.816915513851456,
1.39697105340629));
#63969=CARTESIAN_POINT('Ctrl Pts',(-10.0084171617751,-0.733515838753049,
1.44250947834832));
#63970=CARTESIAN_POINT('Ctrl Pts',(-9.92887353455802,-1.61008105854661,
0.162843684973514));
#63971=CARTESIAN_POINT('Ctrl Pts',(-9.84932990734096,-1.00749744594493,
-1.26642330097038));
#63972=CARTESIAN_POINT('Ctrl Pts',(-9.7697862801239,0.520653648430462,-1.53225287051528));
#63973=CARTESIAN_POINT('Ctrl Pts',(-9.69024265290685,1.57049078956095,-0.39043278644415));
#63974=CARTESIAN_POINT('Ctrl Pts',(-9.61069902568979,1.17754987592476,1.11006998452165));
#63975=CARTESIAN_POINT('Ctrl Pts',(-9.53115539847272,-0.297182239971462,
1.59077396165257));
#63976=CARTESIAN_POINT('Ctrl Pts',(-9.45161177125567,-1.49889905584346,
0.610066144953023));
#63977=CARTESIAN_POINT('Ctrl Pts',(-9.37206814403861,-1.32360769156184,
-0.931097073169421));
#63978=CARTESIAN_POINT('Ctrl Pts',(-9.29252451682155,0.0676552296365225,
-1.61688028336335));
#63979=CARTESIAN_POINT('Ctrl Pts',(-9.21298088960448,1.39676466272872,-0.817268351142129));
#63980=CARTESIAN_POINT('Ctrl Pts',(-9.13343726238743,1.44269471237359,0.73315144937151));
#63981=CARTESIAN_POINT('Ctrl Pts',(-9.05389363517037,0.163250372957315,
1.61003987421294));
#63982=CARTESIAN_POINT('Ctrl Pts',(-8.97435000795331,-1.26616877503531,
1.00781730187167));
#63983=CARTESIAN_POINT('Ctrl Pts',(-8.89480638073625,-1.53238433444625,
-0.520266597399813));
#63984=CARTESIAN_POINT('Ctrl Pts',(-8.81526275351919,-0.390829466992555,
-1.57039211936273));
#63985=CARTESIAN_POINT('Ctrl Pts',(-8.73571912630214,1.10977250973498,-1.1778302328701));
#63986=CARTESIAN_POINT('Ctrl Pts',(-8.65617549908506,1.59084897668441,0.296780414125484));
#63987=CARTESIAN_POINT('Ctrl Pts',(-8.57663187186802,0.610444735014109,
1.4987449103566));
#63988=CARTESIAN_POINT('Ctrl Pts',(-8.49708824465095,-0.930762711094184,
1.32384283676835));
#63989=CARTESIAN_POINT('Ctrl Pts',(-8.4175446174339,-1.61689732093506,-0.0672468168714717));
#63990=CARTESIAN_POINT('Ctrl Pts',(-8.33800099021683,-0.817621136288996,
-1.39655818293396));
#63991=CARTESIAN_POINT('Ctrl Pts',(-8.25845736299976,0.732787013213042,
-1.44287985435121));
#63992=CARTESIAN_POINT('Ctrl Pts',(-8.17891373578272,1.60999858715454,-0.163657050525305));
#63993=CARTESIAN_POINT('Ctrl Pts',(-8.09937010856565,1.00813709349707,1.26591416831537));
#63994=CARTESIAN_POINT('Ctrl Pts',(-8.01982648134859,-0.519879513174783,
1.53251570060716));
#63995=CARTESIAN_POINT('Ctrl Pts',(-7.94028285413154,-1.57029334896946,
0.391226122605003));
#63996=CARTESIAN_POINT('Ctrl Pts',(-7.86073922691447,-1.17811051466681,
-1.10947496414194));
#63997=CARTESIAN_POINT('Ctrl Pts',(-7.78119559969742,0.296378569344132,
-1.59092389021595));
#63998=CARTESIAN_POINT('Ctrl Pts',(-7.70165197248035,1.49859066924594,-0.610823286127277));
#63999=CARTESIAN_POINT('Ctrl Pts',(-7.6221083452633,1.32407789751025,0.930428289633915));
#64000=CARTESIAN_POINT('Ctrl Pts',(-7.54256471804623,-0.066838399815906,
1.61691425534452));
#64001=CARTESIAN_POINT('Ctrl Pts',(-7.46302109082919,-1.39635161403515,
0.817973869269524));
#64002=CARTESIAN_POINT('Ctrl Pts',(-7.3834774636121,-1.44306490426939,-0.73242253030085));
#64003=CARTESIAN_POINT('Ctrl Pts',(-7.30393383639506,-0.164063717651527,
-1.60995719737409));
#64004=CARTESIAN_POINT('Ctrl Pts',(-7.22439020917799,1.26565948082683,-1.00845682080068));
#64005=CARTESIAN_POINT('Ctrl Pts',(-7.14484658196095,1.53264696898959,0.519492395780081));
#64006=CARTESIAN_POINT('Ctrl Pts',(-7.06530295474387,0.391622753256244,
1.57019447838741));
#64007=CARTESIAN_POINT('Ctrl Pts',(-6.98575932752683,-1.10917734776157,
1.178390721297));
#64008=CARTESIAN_POINT('Ctrl Pts',(-6.90621570030976,-1.59099870224241,
-0.295976705653066));
#64009=CARTESIAN_POINT('Ctrl Pts',(-6.8266720730927,-0.611201798268341,
-1.49843633252129));
#64010=CARTESIAN_POINT('Ctrl Pts',(-6.74712844587563,0.930093808809897,
-1.32431287377259));
#64011=CARTESIAN_POINT('Ctrl Pts',(-6.66758481865858,1.61693108659067,0.0664299784959112));
#64012=CARTESIAN_POINT('Ctrl Pts',(-6.58804119144151,0.818326550061182,
1.39614495604548));
#64013=CARTESIAN_POINT('Ctrl Pts',(-6.50849756422447,-0.732058000658186,
1.44324986211628));
#64014=CARTESIAN_POINT('Ctrl Pts',(-6.42895393700739,-1.60991570487421,
0.164470374310088));
#64015=CARTESIAN_POINT('Ctrl Pts',(-6.34941030979035,-1.00877648376213,
-1.26540471258597));
#64016=CARTESIAN_POINT('Ctrl Pts',(-6.26986668257327,0.519105245240422,
-1.53277813958516));
#64017=CARTESIAN_POINT('Ctrl Pts',(-6.19032305535623,1.57009550762287,-0.392019358920946));
#64018=CARTESIAN_POINT('Ctrl Pts',(-6.11077942813917,1.17867085274286,1.10887966061279));
#64019=CARTESIAN_POINT('Ctrl Pts',(-6.0312358009221,-0.295574823077957,
1.59107341275904));
#64020=CARTESIAN_POINT('Ctrl Pts',(-5.95169217370504,-1.49828190019252,
0.611580271413133));
#64021=CARTESIAN_POINT('Ctrl Pts',(-5.87214854648798,-1.32454776554033,
-0.929759268643466));
#64022=CARTESIAN_POINT('Ctrl Pts',(-5.79260491927093,0.0660215529374821,
-1.61694781467246));
#64023=CARTESIAN_POINT('Ctrl Pts',(-5.71306129205386,1.39593820897817,-0.818679178641469));
#64024=CARTESIAN_POINT('Ctrl Pts',(-5.63351766483681,1.44343472788007,0.731693424308328));
#64025=CARTESIAN_POINT('Ctrl Pts',(-5.55397403761973,0.164877020475022,
1.60987410965752));
#64026=CARTESIAN_POINT('Ctrl Pts',(-5.47443041040269,-1.265149863609,1.00909608236106));
#64027=CARTESIAN_POINT('Ctrl Pts',(-5.39488678318562,-1.53290921238552,
-0.518718061580541));
#64028=CARTESIAN_POINT('Ctrl Pts',(-5.31534315596856,-0.392415939573786,
-1.56999643668216));
#64029=CARTESIAN_POINT('Ctrl Pts',(-5.23579952875151,1.10858190271461,-1.17895090898645));
#64030=CARTESIAN_POINT('Ctrl Pts',(-5.15625590153444,1.59114802176109,0.295172921644379));
#64031=CARTESIAN_POINT('Ctrl Pts',(-5.07671227431739,0.611958705537498,
1.49812737226951));
#64032=CARTESIAN_POINT('Ctrl Pts',(-4.99716864710033,-0.929424669155988,
1.32478257279848));
#64033=CARTESIAN_POINT('Ctrl Pts',(-4.91762501988327,-1.61696443958877,
-0.0656131231666956));
#64034=CARTESIAN_POINT('Ctrl Pts',(-4.83808139266621,-0.819031754987941,
-1.3957313728464));
#64035=CARTESIAN_POINT('Ctrl Pts',(-4.75853776544915,0.73132880127457,-1.44361950154899));
#64036=CARTESIAN_POINT('Ctrl Pts',(-4.67899413823209,1.60983241172668,-0.165283656120365));
#64037=CARTESIAN_POINT('Ctrl Pts',(-4.59945051101503,1.00941561657705,1.26489493391218));
#64038=CARTESIAN_POINT('Ctrl Pts',(-4.51990688379797,-0.51833084482508,
1.53304018738233));
#64039=CARTESIAN_POINT('Ctrl Pts',(-4.44036325658091,-1.56989726557164,
0.392812495189444));
#64040=CARTESIAN_POINT('Ctrl Pts',(-4.36081962936385,-1.1792308900099,-1.10828407408602));
#64041=CARTESIAN_POINT('Ctrl Pts',(-4.28127600214679,0.294771001377991,
-1.59122252924377));
#64042=CARTESIAN_POINT('Ctrl Pts',(-4.20173237492973,1.49797274876209,-0.612337100617345));
#64043=CARTESIAN_POINT('Ctrl Pts',(-4.12218874771267,1.32501729553206,0.929090010368841));
#64044=CARTESIAN_POINT('Ctrl Pts',(-4.04264512049562,-0.065204689209657,
1.61698096133857));
#64045=CARTESIAN_POINT('Ctrl Pts',(-3.96310149327855,-1.39552444766335,
0.819384279078032));
#64046=CARTESIAN_POINT('Ctrl Pts',(-3.88355786606149,-1.44380418311125,
-0.730964131580138));
#64047=CARTESIAN_POINT('Ctrl Pts',(-3.80401423884443,-0.165690281220156,
-1.60979061108439));
#64048=CARTESIAN_POINT('Ctrl Pts',(-3.72447061162737,1.26463992351181,-1.00973508638967));
#64049=CARTESIAN_POINT('Ctrl Pts',(-3.64492698441031,1.53317106456717,0.517943594998788));
#64050=CARTESIAN_POINT('Ctrl Pts',(-3.56538335719325,0.393209025742654,
1.56979799429761));
#64051=CARTESIAN_POINT('Ctrl Pts',(-3.4858397299762,-1.10798617474608,1.17951079579536));
#64052=CARTESIAN_POINT('Ctrl Pts',(-3.40629610275913,-1.59129693520231,
-0.294369062304476));
#64053=CARTESIAN_POINT('Ctrl Pts',(-3.32675247554208,-0.612715456628484,
-1.49781802968016));
#64054=CARTESIAN_POINT('Ctrl Pts',(-3.24720884832501,0.928755292303373,
-1.32525193372606));
#64055=CARTESIAN_POINT('Ctrl Pts',(-3.16766522110795,1.61699737992072,0.0647962510922705));
#64056=CARTESIAN_POINT('Ctrl Pts',(-3.0881215938909,0.819736750889412,1.39531743344239));
#64057=CARTESIAN_POINT('Ctrl Pts',(-3.00857796667384,-0.730599415248462,
1.44398877255475));
#64058=CARTESIAN_POINT('Ctrl Pts',(-2.92903433945677,-1.60974870773295,
0.166096895749144));
#64059=CARTESIAN_POINT('Ctrl Pts',(-2.84949071223972,-1.01005449177923,
-1.26438483242538));
#64060=CARTESIAN_POINT('Ctrl Pts',(-2.76994708502266,0.517556312127521,
-1.53330184392934));
#64061=CARTESIAN_POINT('Ctrl Pts',(-2.6904034578056,1.56969862286412,-0.393605531212727));
#64062=CARTESIAN_POINT('Ctrl Pts',(-2.61085983058854,1.17979062632931,1.10768820472246));
#64063=CARTESIAN_POINT('Ctrl Pts',(-2.53131620337148,-0.293967104457652,
1.59137123961546));
#64064=CARTESIAN_POINT('Ctrl Pts',(-2.45177257615442,-1.49766321501792,
0.613093773578183));
#64065=CARTESIAN_POINT('Ctrl Pts',(-2.37222894893736,-1.32548648739524,
-0.928420515040416));
#64066=CARTESIAN_POINT('Ctrl Pts',(-2.2926853217203,0.06438780889704,-1.61701369522131));
#64067=CARTESIAN_POINT('Ctrl Pts',(-2.21314169450324,1.3951103300897,-0.820089170613862));
#64068=CARTESIAN_POINT('Ctrl Pts',(-2.13359806728618,1.44417327007082,0.730234652709602));
#64069=CARTESIAN_POINT('Ctrl Pts',(-2.05405444006912,0.166503499295801,
1.60970670090295));
#64070=CARTESIAN_POINT('Ctrl Pts',(-1.97451081285206,-1.2641296599373,1.01037383419081));
#64071=CARTESIAN_POINT('Ctrl Pts',(-1.894967185635,-1.53343252684967,-0.517168999017592));
#64072=CARTESIAN_POINT('Ctrl Pts',(-1.81542355841794,-0.394002008937513,
-1.56959914599798));
#64073=CARTESIAN_POINT('Ctrl Pts',(-1.73587993120088,1.10739015902935,-1.18007039161467));
#64074=CARTESIAN_POINT('Ctrl Pts',(-1.65633630398382,1.59144545197782,0.293565146883011));
#64075=CARTESIAN_POINT('Ctrl Pts',(-1.57679267676676,0.613472033412145,
1.49750826868494));
#64076=CARTESIAN_POINT('Ctrl Pts',(-1.49724904954971,-0.928085644379445,
1.32572102504447));
#64077=CARTESIAN_POINT('Ctrl Pts',(-1.41770542233264,-1.61702997219381,
-0.0639794927034563));
#64078=CARTESIAN_POINT('Ctrl Pts',(-1.33816179511559,-0.82044141494256,
-1.39490289077172));
#64079=CARTESIAN_POINT('Ctrl Pts',(-1.25861816789853,0.729869609984358,
-1.44435814417302));
#64080=CARTESIAN_POINT('Ctrl Pts',(-1.17907454068147,1.60966503474331,-0.166909202554005));
#64081=CARTESIAN_POINT('Ctrl Pts',(-1.0995309134644,1.01069227059636,1.26387271817383));
#64082=CARTESIAN_POINT('Ctrl Pts',(-1.01998728624735,-0.516780055630681,
1.53356631700391));
#64083=CARTESIAN_POINT('Ctrl Pts',(-0.940443659030288,-1.56950260069087,
0.394392378168218));
#64084=CARTESIAN_POINT('Ctrl Pts',(-0.860900031813227,-1.18034432730794,
-1.10708049621965));
#64085=CARTESIAN_POINT('Ctrl Pts',(-0.781356404596169,0.293152248650012,
-1.59154147850122));
#64086=CARTESIAN_POINT('Ctrl Pts',(-0.701812777379109,1.49737395733561,
-0.613808656846177));
#64087=CARTESIAN_POINT('Ctrl Pts',(-0.62226915016205,1.32591612848784,0.927671758094482));
#64088=CARTESIAN_POINT('Ctrl Pts',(-0.542725522944993,-0.0634964663375496,
1.61719603486571));
#64089=CARTESIAN_POINT('Ctrl Pts',(-0.463181895727927,-1.39483731768548,
0.820508888385569));
#64090=CARTESIAN_POINT('Ctrl Pts',(-0.383638268510867,-1.44427213481421,
-0.72896222268878));
#64091=CARTESIAN_POINT('Ctrl Pts',(-0.30409464129381,-0.167840324100667,
-1.61066856973343));
#64092=CARTESIAN_POINT('Ctrl Pts',(-0.22455101407675,1.26470887814029,-1.00889155965874));
#64093=CARTESIAN_POINT('Ctrl Pts',(-0.171521929265377,1.44219363372905,
0.00454914606926524));
#64094=CARTESIAN_POINT('Ctrl Pts',(-0.145007386859689,1.29672038264059,
0.436605441725649));
#64095=CARTESIAN_POINT('Ctrl Pts',(-34.6914926131403,0.740036351041036,
-1.03579689087092));
#64096=CARTESIAN_POINT('Ctrl Pts',(-34.6649780707346,1.08515513972758,-0.789223019771014));
#64097=CARTESIAN_POINT('Ctrl Pts',(-34.6119489859232,1.50348693841757,0.0717698932582256));
#64098=CARTESIAN_POINT('Ctrl Pts',(-34.5324053587062,0.751010183525675,
1.30613888124279));
#64099=CARTESIAN_POINT('Ctrl Pts',(-34.4528617314891,-0.69201961693675,
1.33667336675341));
#64100=CARTESIAN_POINT('Ctrl Pts',(-34.3733181042721,-1.49898160723127,
0.141201008990934));
#64101=CARTESIAN_POINT('Ctrl Pts',(-34.293774477055,-0.929029926656085,
-1.18501563808319));
#64102=CARTESIAN_POINT('Ctrl Pts',(-34.2142308498379,0.494492460228167,
-1.4220432962459));
#64103=CARTESIAN_POINT('Ctrl Pts',(-34.1346872226209,1.46368736536371,-0.352952500981455));
#64104=CARTESIAN_POINT('Ctrl Pts',(-34.0551435954038,1.08824726743903,1.0405381588406));
#64105=CARTESIAN_POINT('Ctrl Pts',(-33.9755999681868,-0.286956660944541,
1.47802871078736));
#64106=CARTESIAN_POINT('Ctrl Pts',(-33.8960563409697,-1.39853240674266,
0.557725758042946));
#64107=CARTESIAN_POINT('Ctrl Pts',(-33.8165127137527,-1.2253084215944,-0.874970414807997));
#64108=CARTESIAN_POINT('Ctrl Pts',(-33.7369690865356,0.0735834930598086,
-1.50383748004835));
#64109=CARTESIAN_POINT('Ctrl Pts',(-33.6574254593186,1.3048747329139,-0.751165605936964));
#64110=CARTESIAN_POINT('Ctrl Pts',(-33.5778818321015,1.33740453803429,0.691590082910031));
#64111=CARTESIAN_POINT('Ctrl Pts',(-33.4983382048844,0.141287622339839,
1.49899429581447));
#64112=CARTESIAN_POINT('Ctrl Pts',(-33.4187945776674,-1.18462722022883,
0.929303721395224));
#64113=CARTESIAN_POINT('Ctrl Pts',(-33.3392509504503,-1.42224912569989,
-0.494119812806082));
#64114=CARTESIAN_POINT('Ctrl Pts',(-33.2597073232332,-0.353279547106323,
-1.46360524426102));
#64115=CARTESIAN_POINT('Ctrl Pts',(-33.1801636960162,1.04024076886409,-1.08850633470896));
#64116=CARTESIAN_POINT('Ctrl Pts',(-33.1006200687991,1.47811298739213,0.286581349097347));
#64117=CARTESIAN_POINT('Ctrl Pts',(-33.021076441582,0.558072759518739,1.39839252040441));
#64118=CARTESIAN_POINT('Ctrl Pts',(-32.941532814365,-0.87465759731378,1.22552884740331));
#64119=CARTESIAN_POINT('Ctrl Pts',(-32.8619891871479,-1.5038577503335,-0.0732033464336459));
#64120=CARTESIAN_POINT('Ctrl Pts',(-32.7824455599309,-0.751494270205516,
-1.30468510445132));
#64121=CARTESIAN_POINT('Ctrl Pts',(-32.7029019327138,0.691251762826216,
-1.33757910554996));
#64122=CARTESIAN_POINT('Ctrl Pts',(-32.6233583054968,1.49895881315848,-0.141666293436237));
#64123=CARTESIAN_POINT('Ctrl Pts',(-32.5438146782797,0.929602785374642,
1.18439247013284));
#64124=CARTESIAN_POINT('Ctrl Pts',(-32.4642710510626,-0.493760478361972,
1.42237387924739));
#64125=CARTESIAN_POINT('Ctrl Pts',(-32.3847274238456,-1.46351599911086,
0.35364923657973));
#64126=CARTESIAN_POINT('Ctrl Pts',(-32.3051837966285,-1.08876903669851,
-1.03996579120621));
#64127=CARTESIAN_POINT('Ctrl Pts',(-32.2256401694115,0.286207970540554,
-1.47818532661454));
#64128=CARTESIAN_POINT('Ctrl Pts',(-32.1460965421944,1.39825151664009,-0.558425965016473));
#64129=CARTESIAN_POINT('Ctrl Pts',(-32.0665529149773,1.22574973673945,0.87434801141866));
#64130=CARTESIAN_POINT('Ctrl Pts',(-31.9870092877603,-0.0728234805465783,
1.50387619266977));
#64131=CARTESIAN_POINT('Ctrl Pts',(-31.9074656605432,-1.3044952423758,0.751823799046095));
#64132=CARTESIAN_POINT('Ctrl Pts',(-31.8279220333262,-1.33775366694877,
-0.690913879407841));
#64133=CARTESIAN_POINT('Ctrl Pts',(-31.7483784061091,-0.142044913753986,
-1.49892298156748));
#64134=CARTESIAN_POINT('Ctrl Pts',(-31.668834778892,1.18415762247848,-0.929901923495103));
#64135=CARTESIAN_POINT('Ctrl Pts',(-31.589291151675,1.42249855362995,0.493401182725134));
#64136=CARTESIAN_POINT('Ctrl Pts',(-31.5097475244579,0.354018897385096,
1.46342662354088));
#64137=CARTESIAN_POINT('Ctrl Pts',(-31.4302038972408,-1.03969074397971,
1.08903168873859));
#64138=CARTESIAN_POINT('Ctrl Pts',(-31.3506602700238,-1.47825757321933,
-0.285834584005571));
#64139=CARTESIAN_POINT('Ctrl Pts',(-31.2711166428067,-0.558779133992451,
-1.39811041824621));
#64140=CARTESIAN_POINT('Ctrl Pts',(-31.1915730155897,0.874038369267525,
-1.22597055072383));
#64141=CARTESIAN_POINT('Ctrl Pts',(-31.1120293883726,1.50389453930265,0.0724436115169605));
#64142=CARTESIAN_POINT('Ctrl Pts',(-31.0324857611556,0.752153279787823,
1.30430529627782));
#64143=CARTESIAN_POINT('Ctrl Pts',(-30.9529421339385,-0.690575951838579,
1.33792814341286));
#64144=CARTESIAN_POINT('Ctrl Pts',(-30.8733985067215,-1.49888705437755,
0.142423524788989));
#64145=CARTESIAN_POINT('Ctrl Pts',(-30.7938548795044,-0.93020100226633,
-1.18392269915593));
#64146=CARTESIAN_POINT('Ctrl Pts',(-30.7143112522874,0.493041855597954,
-1.42262313731447));
#64147=CARTESIAN_POINT('Ctrl Pts',(-30.6347676250702,1.4633371546058,-0.354388535570987));
#64148=CARTESIAN_POINT('Ctrl Pts',(-30.5552239978532,1.08929427129284,1.0394156304013));
#64149=CARTESIAN_POINT('Ctrl Pts',(-30.4756803706361,-0.28546117923212,
1.47832972551638));
#64150=CARTESIAN_POINT('Ctrl Pts',(-30.3961367434191,-1.39796923065005,
0.55913226731218));
#64151=CARTESIAN_POINT('Ctrl Pts',(-30.316593116202,-1.22619128648771,-0.873728671348003));
#64152=CARTESIAN_POINT('Ctrl Pts',(-30.237049488985,0.0720637378650388,
-1.50391278998447));
#64153=CARTESIAN_POINT('Ctrl Pts',(-30.1575058617679,1.30411526696189,-0.752482712539535));
#64154=CARTESIAN_POINT('Ctrl Pts',(-30.0779622345508,1.33810253451361,0.69023798020842));
#64155=CARTESIAN_POINT('Ctrl Pts',(-29.9984186073338,0.142802126737032,
1.49885103155494));
#64156=CARTESIAN_POINT('Ctrl Pts',(-29.9188749801168,-1.18368770029605,
0.930500021688224));
#64157=CARTESIAN_POINT('Ctrl Pts',(-29.8393313528997,-1.42274763023194,
-0.492682497013374));
#64158=CARTESIAN_POINT('Ctrl Pts',(-29.7597877256826,-0.354758151145976,
-1.46324759230604));
#64159=CARTESIAN_POINT('Ctrl Pts',(-29.6802440984655,1.03914045050549,-1.08955678434728));
#64160=CARTESIAN_POINT('Ctrl Pts',(-29.6007004712485,1.47840178349218,0.285087756245499));
#64161=CARTESIAN_POINT('Ctrl Pts',(-29.5211568440314,0.55948536495782,1.39782795385983));
#64162=CARTESIAN_POINT('Ctrl Pts',(-29.4416132168144,-0.873418917682327,
1.22641194401741));
#64163=CARTESIAN_POINT('Ctrl Pts',(-29.3620695895973,-1.50393094471276,
-0.071683859615264));
#64164=CARTESIAN_POINT('Ctrl Pts',(-29.2825259623802,-0.752812097280904,
-1.30392515444003));
#64165=CARTESIAN_POINT('Ctrl Pts',(-29.2029823351632,0.689899964539293,
-1.33827684023995));
#64166=CARTESIAN_POINT('Ctrl Pts',(-29.1234387079461,1.49881491310176,-0.143180719573932));
#64167=CARTESIAN_POINT('Ctrl Pts',(-29.0438950807291,0.930798981741808,
1.18345262591384));
#64168=CARTESIAN_POINT('Ctrl Pts',(-28.964351453512,-0.492323106994374,
1.42287203237443));
#64169=CARTESIAN_POINT('Ctrl Pts',(-28.884807826295,-1.4631579366473,0.355127744086476));
#64170=CARTESIAN_POINT('Ctrl Pts',(-28.8052641990779,-1.08981922788518,
-1.03886520430982));
#64171=CARTESIAN_POINT('Ctrl Pts',(-28.7257205718608,0.284714315069542,
-1.47847374714211));
#64172=CARTESIAN_POINT('Ctrl Pts',(-28.6461769446438,1.39768658788457,-0.559838426906849));
#64173=CARTESIAN_POINT('Ctrl Pts',(-28.5666333174267,1.22663252329886,0.873109108290266));
#64174=CARTESIAN_POINT('Ctrl Pts',(-28.4870896902097,-0.0713039767918712,
1.50394900348636));
#64175=CARTESIAN_POINT('Ctrl Pts',(-28.4075460629926,-1.30373495872438,
0.75314143399091));
#64176=CARTESIAN_POINT('Ctrl Pts',(-28.3280024357756,-1.33845106058076,
-0.689561904852759));
#64177=CARTESIAN_POINT('Ctrl Pts',(-28.2484588085585,-0.143559303275531,
-1.4987786990203));
#64178=CARTESIAN_POINT('Ctrl Pts',(-28.1689151813415,1.18321747602428,-0.931097882408006));
#64179=CARTESIAN_POINT('Ctrl Pts',(-28.0893715541243,1.422996343734,0.491963685563887));
#64180=CARTESIAN_POINT('Ctrl Pts',(-28.0098279269073,0.355497314368909,
1.4630681876353));
#64181=CARTESIAN_POINT('Ctrl Pts',(-27.9302842996902,-1.03858989183187,
1.09008160188979));
#64182=CARTESIAN_POINT('Ctrl Pts',(-27.8507406724732,-1.47854561646158,
-0.284340855728072));
#64183=CARTESIAN_POINT('Ctrl Pts',(-27.7711970452561,-0.560191453136734,
-1.39754513273328));
#64184=CARTESIAN_POINT('Ctrl Pts',(-27.6916534180391,0.87279924319158,-1.22685302431797));
#64185=CARTESIAN_POINT('Ctrl Pts',(-27.612109790822,1.50396696630412,0.0709240894191014));
#64186=CARTESIAN_POINT('Ctrl Pts',(-27.532566163605,0.753470722648544,1.30354467982705));
#64187=CARTESIAN_POINT('Ctrl Pts',(-27.4530225363879,-0.689223801170392,
1.33862519552494));
#64188=CARTESIAN_POINT('Ctrl Pts',(-27.3734789091708,-1.49874238931288,
0.143937877817675));
#64189=CARTESIAN_POINT('Ctrl Pts',(-27.2939352819538,-0.931396723667748,
-1.18298225064238));
#64190=CARTESIAN_POINT('Ctrl Pts',(-27.2143916547367,0.491604232744841,
-1.42312056430272));
#64191=CARTESIAN_POINT('Ctrl Pts',(-27.1348480275197,1.46297834527575,-0.355866861969689));
#64192=CARTESIAN_POINT('Ctrl Pts',(-27.0553044003026,1.09034390634437,1.03831451308919));
#64193=CARTESIAN_POINT('Ctrl Pts',(-26.9757607730855,-0.283967378244922,
1.47861739144602));
#64194=CARTESIAN_POINT('Ctrl Pts',(-26.8962171458685,-1.397403588415,0.560544443624956));
#64195=CARTESIAN_POINT('Ctrl Pts',(-26.8166735186514,-1.22707344706068,
-0.872489322406045));
#64196=CARTESIAN_POINT('Ctrl Pts',(-26.7371298914344,0.0705441975211899,
-1.50398483316489));
#64197=CARTESIAN_POINT('Ctrl Pts',(-26.6575862642173,1.30335431776021,-0.753799963232794));
#64198=CARTESIAN_POINT('Ctrl Pts',(-26.5780426370002,1.33879924506136,0.688885653513762));
#64199=CARTESIAN_POINT('Ctrl Pts',(-26.4984990097832,0.144316443176208,
1.49870598398182));
#64200=CARTESIAN_POINT('Ctrl Pts',(-26.4189553825661,-1.18274694978316,
0.931695505501969));
#64201=CARTESIAN_POINT('Ctrl Pts',(-26.339411755349,-1.42324469407266,-0.491244748560173));
#64202=CARTESIAN_POINT('Ctrl Pts',(-26.259868128132,-0.356236386865245,
-1.46288840957441));
#64203=CARTESIAN_POINT('Ctrl Pts',(-26.1803245009149,1.03803906809936,-1.09060614123218));
#64204=CARTESIAN_POINT('Ctrl Pts',(-26.1007808736979,1.47868907209085,0.283593882643916));
#64205=CARTESIAN_POINT('Ctrl Pts',(-26.0212372464808,0.560897398348989,
1.39726195493876));
#64206=CARTESIAN_POINT('Ctrl Pts',(-25.9416936192638,-0.87217934595343,
1.22729379151293));
#64207=CARTESIAN_POINT('Ctrl Pts',(-25.8621499920467,-1.50400260406754,
-0.0701643011223775));
#64208=CARTESIAN_POINT('Ctrl Pts',(-25.7826063648297,-0.754129155722656,
-1.30316387253598));
#64209=CARTESIAN_POINT('Ctrl Pts',(-25.7030627376126,0.688547461904444,
-1.33897320917892));
#64210=CARTESIAN_POINT('Ctrl Pts',(-25.6235191103955,1.49866948302943,-0.144694999326982));
#64211=CARTESIAN_POINT('Ctrl Pts',(-25.5439754831785,0.931994227891605,
1.18251157346162));
#64212=CARTESIAN_POINT('Ctrl Pts',(-25.4644318559614,-0.490885233032826,
1.42336873303591));
#64213=CARTESIAN_POINT('Ctrl Pts',(-25.3848882287444,-1.46279838053699,
0.356605889031989));
#64214=CARTESIAN_POINT('Ctrl Pts',(-25.3053446015273,-1.0908683065365,-1.03776355687995));
#64215=CARTESIAN_POINT('Ctrl Pts',(-25.2258009743102,0.283220368948894,
-1.47876065839148));
#64216=CARTESIAN_POINT('Ctrl Pts',(-25.1462573470932,1.39712023231358,-0.561250317286305));
#64217=CARTESIAN_POINT('Ctrl Pts',(-25.0667137198761,1.22751405766065,0.871869313853523));
#64218=CARTESIAN_POINT('Ctrl Pts',(-24.987170092659,-0.069784400246911,
1.50402027901093));
#64219=CARTESIAN_POINT('Ctrl Pts',(-24.907626465442,-1.30297334416653,0.754458300097118));
#64220=CARTESIAN_POINT('Ctrl Pts',(-24.8280828382249,-1.33914708786651,
-0.688209226364027));
#64221=CARTESIAN_POINT('Ctrl Pts',(-24.7485392110079,-0.14507354624583,
-1.49863288645805));
#64222=CARTESIAN_POINT('Ctrl Pts',(-24.6689955837908,1.18227612169278,-0.932292890817585));
#64223=CARTESIAN_POINT('Ctrl Pts',(-24.5894519565737,1.42349268118454,0.490525686185724));
#64224=CARTESIAN_POINT('Ctrl Pts',(-24.5099083293567,0.356975368446356,
1.46270825816925));
#64225=CARTESIAN_POINT('Ctrl Pts',(-24.4303647021396,-1.03748797944855,
1.0911304022406));
#64226=CARTESIAN_POINT('Ctrl Pts',(-24.3508210749226,-1.47883215034335,
-0.282846837183695));
#64227=CARTESIAN_POINT('Ctrl Pts',(-24.2712774477055,-0.56160320041439,
-1.39697842054852));
#64228=CARTESIAN_POINT('Ctrl Pts',(-24.1917338204884,0.871559226126107,
-1.2277342454898));
#64229=CARTESIAN_POINT('Ctrl Pts',(-24.1121901932714,1.50403785799393,0.0694044949190318));
#64230=CARTESIAN_POINT('Ctrl Pts',(-24.0326465660543,0.754787396335176,
1.30278273266401));
#64231=CARTESIAN_POINT('Ctrl Pts',(-23.9531029388373,-0.687870946914086,
1.33932088111306));
#64232=CARTESIAN_POINT('Ctrl Pts',(-23.8735593116202,-1.49859619427002,
0.145452083908596));
#64233=CARTESIAN_POINT('Ctrl Pts',(-23.7940156844031,-0.932591494260859,
-1.18204059449168));
#64234=CARTESIAN_POINT('Ctrl Pts',(-23.7144720571861,0.490166108041832,
-1.42361653851066));
#64235=CARTESIAN_POINT('Ctrl Pts',(-23.634928429969,1.46261804247694,-0.357344825084754));
#64236=CARTESIAN_POINT('Ctrl Pts',(-23.555384802752,1.09139242832774,1.03721233582272));
#64237=CARTESIAN_POINT('Ctrl Pts',(-23.4758411755349,-0.282473287372118,
1.4789035479419));
#64238=CARTESIAN_POINT('Ctrl Pts',(-23.3962975483179,-1.39683651965262,
0.561956047710764));
#64239=CARTESIAN_POINT('Ctrl Pts',(-23.3167539211008,-1.22795435498632,
-0.871249082790945));
#64240=CARTESIAN_POINT('Ctrl Pts',(-23.2372102938837,0.0690245851629364,
-1.50405534101542));
#64241=CARTESIAN_POINT('Ctrl Pts',(-23.1576666666667,1.30259203804057,-0.755116444415858));
#64242=CARTESIAN_POINT('Ctrl Pts',(-23.0781230394496,1.33949458890747,0.687532623576175));
#64243=CARTESIAN_POINT('Ctrl Pts',(-22.9985794122326,0.145830612291159,
1.49855940646767));
#64244=CARTESIAN_POINT('Ctrl Pts',(-22.9190357850155,-1.1818049918733,0.932890038202402));
#64245=CARTESIAN_POINT('Ctrl Pts',(-22.8394921577985,-1.42374030500635,
-0.48980649862406));
#64246=CARTESIAN_POINT('Ctrl Pts',(-22.7599485305814,-0.357714258923656,
-1.46252773346581));
#64247=CARTESIAN_POINT('Ctrl Pts',(-22.6804049033643,1.03693662602006,-1.09165438478123));
#64248=CARTESIAN_POINT('Ctrl Pts',(-22.6008612761473,1.47897485118257,0.282099719538004));
#64249=CARTESIAN_POINT('Ctrl Pts',(-22.5213176489302,0.562308859152876,
1.39669452963493));
#64250=CARTESIAN_POINT('Ctrl Pts',(-22.4417740217131,-0.870938883867826,
1.22817438613619));
#64251=CARTESIAN_POINT('Ctrl Pts',(-22.3622303944961,-1.50407272807429,
-0.068644671002907));
#64252=CARTESIAN_POINT('Ctrl Pts',(-22.282686767279,-0.755445444318166,
-1.30240126030838));
#64253=CARTESIAN_POINT('Ctrl Pts',(-22.2031431400619,0.687194256371912,
-1.33966821123866));
#64254=CARTESIAN_POINT('Ctrl Pts',(-22.1235995128449,1.49852252305334,-0.146209131369364));
#64255=CARTESIAN_POINT('Ctrl Pts',(-22.0440558856278,0.933188522623136,
1.18156931385272));
#64256=CARTESIAN_POINT('Ctrl Pts',(-21.9645122584108,-0.489446857955352,
1.42386398066373));
#64257=CARTESIAN_POINT('Ctrl Pts',(-21.8849686311937,-1.46243733114162,
0.358083669939449));
#64258=CARTESIAN_POINT('Ctrl Pts',(-21.8054250039767,-1.09191627158435,
-1.03666085005814));
#64259=CARTESIAN_POINT('Ctrl Pts',(-21.7258813767596,0.281726133705207,
-1.47904606006083));
#64260=CARTESIAN_POINT('Ctrl Pts',(-21.6463377495426,1.39655245050451,-0.562661634718235));
#64261=CARTESIAN_POINT('Ctrl Pts',(-21.5667941223254,1.22839433892534,0.870628629376558));
#64262=CARTESIAN_POINT('Ctrl Pts',(-21.4872504951085,-0.0682647524631571,
1.50409001916943));
#64263=CARTESIAN_POINT('Ctrl Pts',(-21.4077068678913,-1.30221039947963,
0.755774396021086));
#64264=CARTESIAN_POINT('Ctrl Pts',(-21.3281632406743,-1.33984174809555,
-0.686855845322866));
#64265=CARTESIAN_POINT('Ctrl Pts',(-21.2486196134572,-0.146587641119035,
-1.4984855440294));
#64266=CARTESIAN_POINT('Ctrl Pts',(-21.1690759862402,1.18133356044495,-0.933486947504037));
#64267=CARTESIAN_POINT('Ctrl Pts',(-21.0895323590231,1.4239875654749,0.48908718605868));
#64268=CARTESIAN_POINT('Ctrl Pts',(-21.0099887318061,0.358453058108589,
1.46234683551015));
#64269=CARTESIAN_POINT('Ctrl Pts',(-20.930445104589,-1.03638500795459,1.09217808872037));
#64270=CARTESIAN_POINT('Ctrl Pts',(-20.8509014773719,-1.47911717457211,
-0.281352529897543));
#64271=CARTESIAN_POINT('Ctrl Pts',(-20.7713578501549,-0.563014374384315,
-1.39641028227043));
#64272=CARTESIAN_POINT('Ctrl Pts',(-20.6918142229378,0.870318319336921,
-1.22861421333977));
#64273=CARTESIAN_POINT('Ctrl Pts',(-20.6122705957208,1.50410721429972,0.0678848295679509));
#64274=CARTESIAN_POINT('Ctrl Pts',(-20.5327269685037,0.756103299503655,
1.30201945556648));
#64275=CARTESIAN_POINT('Ctrl Pts',(-20.4531833412866,-0.686517390450649,
1.34001519946707));
#64276=CARTESIAN_POINT('Ctrl Pts',(-20.3736397140696,-1.49844846939821,
0.146966141516047));
#64277=CARTESIAN_POINT('Ctrl Pts',(-20.2940960868525,-0.933785312826044,
-1.18109773166504));
#64278=CARTESIAN_POINT('Ctrl Pts',(-20.2145524596355,0.488727482956969,
-1.42411105943198));
#64279=CARTESIAN_POINT('Ctrl Pts',(-20.1350088324184,1.46225624657716,-0.358822423407484));
#64280=CARTESIAN_POINT('Ctrl Pts',(-20.0554652052013,1.09243983617262,1.03610909972699));
#64281=CARTESIAN_POINT('Ctrl Pts',(-19.9759215779843,-0.280978908138871,
1.47918819471189));
#64282=CARTESIAN_POINT('Ctrl Pts',(-19.8963779507672,-1.39626802494175,
0.563367078128633));
#64283=CARTESIAN_POINT('Ctrl Pts',(-19.8168343235502,-1.22883400936541,
-0.870007953768733));
#64284=CARTESIAN_POINT('Ctrl Pts',(-19.7372906963331,0.0675049023415035,
-1.50412431346408));
#64285=CARTESIAN_POINT('Ctrl Pts',(-19.657747069116,1.30182842858112,-0.756432154744866));
#64286=CARTESIAN_POINT('Ctrl Pts',(-19.578203441899,1.34018856534215,0.686178891776835));
#64287=CARTESIAN_POINT('Ctrl Pts',(-19.4986598146819,0.147344632536228,
1.49841129916212));
#64288=CARTESIAN_POINT('Ctrl Pts',(-19.4191161874649,-1.18086182752804,
0.934083618570138));
#64289=CARTESIAN_POINT('Ctrl Pts',(-19.3395725602478,-1.42423446252709,
-0.488367748673187));
#64290=CARTESIAN_POINT('Ctrl Pts',(-19.2600289330307,-0.35919176581259,
-1.46216556434843));
#64291=CARTESIAN_POINT('Ctrl Pts',(-19.1804853058137,1.03583312539295,-1.09270151392437));
#64292=CARTESIAN_POINT('Ctrl Pts',(-19.1009416785966,1.47925912047564,0.280605268453003));
#64293=CARTESIAN_POINT('Ctrl Pts',(-19.0213980513796,0.563719745928661,
1.39612567852757));
#64294=CARTESIAN_POINT('Ctrl Pts',(-18.9418544241625,-0.869697532691776,
1.22905372698828));
#64295=CARTESIAN_POINT('Ctrl Pts',(-18.8623107969454,-1.50414131666142,
-0.0671249708080826));
#64296=CARTESIAN_POINT('Ctrl Pts',(-18.7827671697284,-0.756760961723758,
-1.30163731853572));
#64297=CARTESIAN_POINT('Ctrl Pts',(-18.7032235425113,0.685840349323042,
-1.34036184570973));
#64298=CARTESIAN_POINT('Ctrl Pts',(-18.6236799152943,1.49837403332351,-0.14772311415545));
#64299=CARTESIAN_POINT('Ctrl Pts',(-18.5441362880772,0.934381864717273,
1.180625848049));
#64300=CARTESIAN_POINT('Ctrl Pts',(-18.4645926608601,-0.488007983230271,
1.42435777475235));
#64301=CARTESIAN_POINT('Ctrl Pts',(-18.3850490336431,-1.46207478882976,
0.359561085300321));
#64302=CARTESIAN_POINT('Ctrl Pts',(-18.305505406426,-1.09296312195894,-1.03555708497007));
#64303=CARTESIAN_POINT('Ctrl Pts',(-18.225961779209,0.280231610863807,-1.47932995185882));
#64304=CARTESIAN_POINT('Ctrl Pts',(-18.1464181519919,1.39598324303695,-0.56407237776192));
#64305=CARTESIAN_POINT('Ctrl Pts',(-18.0668745247749,1.22927336619432,0.869387056125872));
#64306=CARTESIAN_POINT('Ctrl Pts',(-17.9873308975578,-0.0667450349919024,
1.50415822389065));
#64307=CARTESIAN_POINT('Ctrl Pts',(-17.9077872703407,-1.30144612544251,
0.75708972041933));
#64308=CARTESIAN_POINT('Ctrl Pts',(-17.8282436431237,-1.34053504055875,
-0.685501763110848));
#64309=CARTESIAN_POINT('Ctrl Pts',(-17.7487000159066,-0.148101586349544,
-1.49833667188476));
#64310=CARTESIAN_POINT('Ctrl Pts',(-17.6691563886896,1.18038979324296,-0.934680051248432));
#64311=CARTESIAN_POINT('Ctrl Pts',(-17.5896127614725,1.42448099609989,0.48764818665119));
#64312=CARTESIAN_POINT('Ctrl Pts',(-17.5100691342554,0.359930381847136,
1.46198392002693));
#64313=CARTESIAN_POINT('Ctrl Pts',(-17.4305255070384,-1.03528097847597,
1.09322466025962));
#64314=CARTESIAN_POINT('Ctrl Pts',(-17.3509818798213,-1.47940068885692,
-0.279857935395096));
#64315=CARTESIAN_POINT('Ctrl Pts',(-17.2714382526042,-0.564424973605891,
-1.39584071847899));
#64316=CARTESIAN_POINT('Ctrl Pts',(-17.1918946253872,0.869076524090815,
-1.22949292696956));
#64317=CARTESIAN_POINT('Ctrl Pts',(-17.1123509981701,1.50417503515068,0.0663650949172277));
#64318=CARTESIAN_POINT('Ctrl Pts',(-17.0328073709531,0.757418430810628,
1.30125484931366));
#64319=CARTESIAN_POINT('Ctrl Pts',(-16.953263743736,-0.685163133161878,
1.34070814987817));
#64320=CARTESIAN_POINT('Ctrl Pts',(-16.873720116519,-1.49829921484824,0.148480049094385));
#64321=CARTESIAN_POINT('Ctrl Pts',(-16.7941764893019,-0.934978178144577,
-1.18015366312501));
#64322=CARTESIAN_POINT('Ctrl Pts',(-16.7146328620849,0.487288358958884,
-1.42460412656187));
#64323=CARTESIAN_POINT('Ctrl Pts',(-16.6350892348678,1.46189295794575,-0.360299655429449));
#64324=CARTESIAN_POINT('Ctrl Pts',(-16.5555456076507,1.09348612880975,1.03500480592826));
#64325=CARTESIAN_POINT('Ctrl Pts',(-16.4760019804336,-0.279484242070737,
1.47947133146543));
#64326=CARTESIAN_POINT('Ctrl Pts',(-16.3964583532166,-1.39569810486277,
0.564777533438098));
#64327=CARTESIAN_POINT('Ctrl Pts',(-16.3169147259995,-1.22971240929995,
-0.868765936606435));
#64328=CARTESIAN_POINT('Ctrl Pts',(-16.2373710987825,0.0659851506082771,
-1.50419175044046));
#64329=CARTESIAN_POINT('Ctrl Pts',(-16.1578274715654,1.30106349016138,-0.757747092876659));
#64330=CARTESIAN_POINT('Ctrl Pts',(-16.0782838443484,1.34088117365694,0.684824459497715));
#64331=CARTESIAN_POINT('Ctrl Pts',(-15.9987402171313,0.148858502365802,
1.49826166221637));
#64332=CARTESIAN_POINT('Ctrl Pts',(-15.9191965899142,-1.1799174577102,0.9352762453867));
#64333=CARTESIAN_POINT('Ctrl Pts',(-15.8396529626972,-1.4247271661304,-0.486928500176328));
#64334=CARTESIAN_POINT('Ctrl Pts',(-15.7601093354801,-0.360668906023721,
-1.461801902592));
#64335=CARTESIAN_POINT('Ctrl Pts',(-15.6805657082631,1.03472856734457,-1.09374752759263));
#64336=CARTESIAN_POINT('Ctrl Pts',(-15.601022081046,1.47954187967984,0.279110530914547));
#64337=CARTESIAN_POINT('Ctrl Pts',(-15.521478453829,0.565130057236024,1.3955554021974));
#64338=CARTESIAN_POINT('Ctrl Pts',(-15.4419348266119,-0.868455293692529,
1.22993181317151));
#64339=CARTESIAN_POINT('Ctrl Pts',(-15.3623911993948,-1.50420836975891,
-0.0656052020893142));
#64340=CARTESIAN_POINT('Ctrl Pts',(-15.2828475721778,-0.758075706596474,
-1.30087204799788));
#64341=CARTESIAN_POINT('Ctrl Pts',(-15.2033039449607,0.684485742139975,
-1.34105411188401));
#64342=CARTESIAN_POINT('Ctrl Pts',(-15.1237603177436,1.4982240139915,-0.149236946139704));
#64343=CARTESIAN_POINT('Ctrl Pts',(-15.0442166905266,0.935574252955802,
1.17968117701358));
#64344=CARTESIAN_POINT('Ctrl Pts',(-14.9646730633095,-0.486568610326457,
1.42485011479767));
#64345=CARTESIAN_POINT('Ctrl Pts',(-14.8851294360925,-1.4617107539715,0.361038133606384));
#64346=CARTESIAN_POINT('Ctrl Pts',(-14.8055858088754,-1.0940088565916,-1.03445226274248));
#64347=CARTESIAN_POINT('Ctrl Pts',(-14.7260421816584,0.278736801950366,
-1.47961233349565));
#64348=CARTESIAN_POINT('Ctrl Pts',(-14.6464985544413,1.39541261049198,-0.565482544977215));
#64349=CARTESIAN_POINT('Ctrl Pts',(-14.5669549272242,1.23015113857024,0.868144595368921));
#64350=CARTESIAN_POINT('Ctrl Pts',(-14.4874113000072,-0.065225249384528,
1.50422489310497));
#64351=CARTESIAN_POINT('Ctrl Pts',(-14.4078676727901,-1.30068052283537,
0.758404271949116));
#64352=CARTESIAN_POINT('Ctrl Pts',(-14.328324045573,-1.34122696454837,-0.684146981110283));
#64353=CARTESIAN_POINT('Ctrl Pts',(-14.248780418356,-0.149615380391841,
-1.49818627017608));
#64354=CARTESIAN_POINT('Ctrl Pts',(-14.1692367911389,1.17944482105025,-0.935872200832809));
#64355=CARTESIAN_POINT('Ctrl Pts',(-14.0896931639219,1.42497297255581,0.486208689432246));
#64356=CARTESIAN_POINT('Ctrl Pts',(-14.0101495367048,0.361407338153881,
1.46161951209009));
#64357=CARTESIAN_POINT('Ctrl Pts',(-13.9306059094878,-1.03417589213971,
1.09427011578995));
#64358=CARTESIAN_POINT('Ctrl Pts',(-13.8510622822707,-1.47968269290834,
-0.27836305520207));
#64359=CARTESIAN_POINT('Ctrl Pts',(-13.7715186550536,-0.56583499663915,
-1.39526972975562));
#64360=CARTESIAN_POINT('Ctrl Pts',(-13.6919750278366,0.867833841655458,
-1.23037038548215));
#64361=CARTESIAN_POINT('Ctrl Pts',(-13.6124314006195,1.50424132047758,0.0648452925182609));
#64362=CARTESIAN_POINT('Ctrl Pts',(-13.5328877734025,0.758732788913574,
1.30048891468607));
#64363=CARTESIAN_POINT('Ctrl Pts',(-13.4533441461854,-0.683808176430229,
1.34139973163898));
#64364=CARTESIAN_POINT('Ctrl Pts',(-13.3738005189683,-1.49814843077251,
0.149993805098161));
#64365=CARTESIAN_POINT('Ctrl Pts',(-13.2942568917513,-0.936170088998737,
-1.17920838983532));
#64366=CARTESIAN_POINT('Ctrl Pts',(-13.2147132645342,0.485848737516666,
-1.42509573939696));
#64367=CARTESIAN_POINT('Ctrl Pts',(-13.1351696373171,1.46152817695356,-0.361776519642661));
#64368=CARTESIAN_POINT('Ctrl Pts',(-13.0556260101001,1.09453130517105,1.03389945555383));
#64369=CARTESIAN_POINT('Ctrl Pts',(-12.976082382883,-0.277989290693522,
1.47975295791346));
#64370=CARTESIAN_POINT('Ctrl Pts',(-12.896538755666,-1.39512675999743,0.566187412199333));
#64371=CARTESIAN_POINT('Ctrl Pts',(-12.8169951284489,-1.23058955389324,
-0.867523032571931));
#64372=CARTESIAN_POINT('Ctrl Pts',(-12.7374515012319,0.0644653315146698,
-1.50425765187572));
#64373=CARTESIAN_POINT('Ctrl Pts',(-12.6579078740148,1.30029722356223,-0.759061257468899));
#64374=CARTESIAN_POINT('Ctrl Pts',(-12.5783642467977,1.34157241314479,0.683469328121443));
#64375=CARTESIAN_POINT('Ctrl Pts',(-12.4988206195807,0.150372220234496,
1.49811049578318));
#64376=CARTESIAN_POINT('Ctrl Pts',(-12.4192769923636,-1.17897188338383,
0.936467917434619));
#64377=CARTESIAN_POINT('Ctrl Pts',(-12.3397333651466,-1.42521841531332,
-0.485488754602712));
#64378=CARTESIAN_POINT('Ctrl Pts',(-12.2601897379295,-0.36214567804915,
-1.46143674856774));
#64379=CARTESIAN_POINT('Ctrl Pts',(-12.1806461107125,1.03362295300247,-1.09479242471822));
#64380=CARTESIAN_POINT('Ctrl Pts',(-12.1011024834954,1.47982312850652,0.277615508448512));
#64381=CARTESIAN_POINT('Ctrl Pts',(-12.0215588562783,0.566539791635272,
1.39498370122657));
#64382=CARTESIAN_POINT('Ctrl Pts',(-11.9420152290612,-0.867212168138187,
1.23080864378951));
#64383=CARTESIAN_POINT('Ctrl Pts',(-11.8624716018442,-1.50427388729832,
-0.0640853663980119));
#64384=CARTESIAN_POINT('Ctrl Pts',(-11.7829279746271,-0.759389677594182,
-1.30010544947607));
#64385=CARTESIAN_POINT('Ctrl Pts',(-11.7033843474101,0.683130436205578,
-1.34174500905481));
#64386=CARTESIAN_POINT('Ctrl Pts',(-11.623840720193,1.4980724652105,-0.150750625776684));
#64387=CARTESIAN_POINT('Ctrl Pts',(-11.544297092976,0.936765686121424,1.17873530171087));
#64388=CARTESIAN_POINT('Ctrl Pts',(-11.4647534657589,-0.485128740713296,
1.42534100029708));
#64389=CARTESIAN_POINT('Ctrl Pts',(-11.3852098385418,-1.46134522693848,
0.362514813349782));
#64390=CARTESIAN_POINT('Ctrl Pts',(-11.3056662113248,-1.09505347441479,
-1.03334638450329));
#64391=CARTESIAN_POINT('Ctrl Pts',(-11.2261225841077,0.277241708490902,
-1.47989320468303));
#64392=CARTESIAN_POINT('Ctrl Pts',(-11.1465789568907,1.39484055345213,-0.566892134924538));
#64393=CARTESIAN_POINT('Ctrl Pts',(-11.0670353296736,1.231027655157,0.866901248374095));
#64394=CARTESIAN_POINT('Ctrl Pts',(-10.9874917024566,-0.0637053971925516,
1.50429002674433));
#64395=CARTESIAN_POINT('Ctrl Pts',(-10.9079480752395,-1.29991359243979,
0.75971804926844));
#64396=CARTESIAN_POINT('Ctrl Pts',(-10.8284044480224,-1.34191751935805,
-0.682791500704204));
#64397=CARTESIAN_POINT('Ctrl Pts',(-10.7488608208054,-0.151129021700562,
-1.49803433905693));
#64398=CARTESIAN_POINT('Ctrl Pts',(-10.6693171935883,1.17849864483154,-0.937063395040135));
#64399=CARTESIAN_POINT('Ctrl Pts',(-10.5897735663713,1.42546349434039,0.484768695871397));
#64400=CARTESIAN_POINT('Ctrl Pts',(-10.5102299391542,0.362883925521062,
1.46125361207163));
#64401=CARTESIAN_POINT('Ctrl Pts',(-10.4306863119371,-1.03306975007396,
1.09531445424409));
#64402=CARTESIAN_POINT('Ctrl Pts',(-10.3511426847201,-1.4799631864385,-0.276867890844559));
#64403=CARTESIAN_POINT('Ctrl Pts',(-10.271599057503,-0.56724444204462,-1.39469731668325));
#64404=CARTESIAN_POINT('Ctrl Pts',(-10.1920554302859,0.866590273299441,
-1.23124658798177));
#64405=CARTESIAN_POINT('Ctrl Pts',(-10.1125118030689,1.50430607021276,0.0633254239225505));
#64406=CARTESIAN_POINT('Ctrl Pts',(-10.0329681758518,0.760046372470701,
1.29972165246565));
#64407=CARTESIAN_POINT('Ctrl Pts',(-9.95342454863479,-0.682452521638949,
1.34208994404347));
#64408=CARTESIAN_POINT('Ctrl Pts',(-9.8738809214177,-1.49799611732492,0.151507407982049));
#64409=CARTESIAN_POINT('Ctrl Pts',(-9.79433729420066,-0.937361044171762,
-1.17826191276097));
#64410=CARTESIAN_POINT('Ctrl Pts',(-9.71479366698359,0.484408620100003,
-1.42558589743541));
#64411=CARTESIAN_POINT('Ctrl Pts',(-9.63525003976654,1.461161903973,-0.363253014539415));
#64412=CARTESIAN_POINT('Ctrl Pts',(-9.55570641254947,1.09557536418953,1.0327930497321));
#64413=CARTESIAN_POINT('Ctrl Pts',(-9.47616278533242,-0.276494055533358,
1.4800330737685));
#64414=CARTESIAN_POINT('Ctrl Pts',(-9.39661915811535,-1.39455399092905,
0.567596712973026));
#64415=CARTESIAN_POINT('Ctrl Pts',(-9.3170755308983,-1.23146544224981,-0.866279242934072));
#64416=CARTESIAN_POINT('Ctrl Pts',(-9.23753190368124,0.0629454466121958,
-1.50432201770258));
#64417=CARTESIAN_POINT('Ctrl Pts',(-9.15798827646418,1.29952962956593,-0.760374647180021));
#64418=CARTESIAN_POINT('Ctrl Pts',(-9.07844464924712,1.34226228310006,0.682113499031458));
#64419=CARTESIAN_POINT('Ctrl Pts',(-8.99890102203006,0.15188578459698,1.49795780001685));
#64420=CARTESIAN_POINT('Ctrl Pts',(-8.919357394813,-1.17802510551424,0.937658633497361));
#64421=CARTESIAN_POINT('Ctrl Pts',(-8.83981376759594,-1.42570820957437,
-0.484048513422119));
#64422=CARTESIAN_POINT('Ctrl Pts',(-8.76027014037887,-0.363622080381272,
-1.46107010264844));
#64423=CARTESIAN_POINT('Ctrl Pts',(-8.68072651316182,1.03251628349535,-1.09583620423442));
#64424=CARTESIAN_POINT('Ctrl Pts',(-8.60118288594475,1.48010286666857,0.276120202581098));
#64425=CARTESIAN_POINT('Ctrl Pts',(-8.5216392587277,0.567948947687269,1.39441057619872));
#64426=CARTESIAN_POINT('Ctrl Pts',(-8.44209563151064,-0.865968157297839,
1.23168421794716));
#64427=CARTESIAN_POINT('Ctrl Pts',(-8.36255200429358,-1.50433786921275,
-0.0625654652857498));
#64428=CARTESIAN_POINT('Ctrl Pts',(-8.28300837707652,-0.760702873375501,
-1.29933752375286));
#64429=CARTESIAN_POINT('Ctrl Pts',(-8.20346474985946,0.681774432903392,
-1.34243453651684));
#64430=CARTESIAN_POINT('Ctrl Pts',(-8.12392112264241,1.49791938713518,-0.152264151521192));
#64431=CARTESIAN_POINT('Ctrl Pts',(-8.04437749542534,0.937956162997909,
1.17778822310643));
#64432=CARTESIAN_POINT('Ctrl Pts',(-7.96483386820828,-0.483688375860664,
1.42583043074948));
#64433=CARTESIAN_POINT('Ctrl Pts',(-7.88529024099122,-1.46097820810384,
0.363991123023073));
#64434=CARTESIAN_POINT('Ctrl Pts',(-7.80574661377416,-1.09609697436211,
-1.03223945138139));
#64435=CARTESIAN_POINT('Ctrl Pts',(-7.72620298655711,0.275746332011639,
-1.48017256513424));
#64436=CARTESIAN_POINT('Ctrl Pts',(-7.64665935934005,1.39426707250139,-0.568301146164932));
#64437=CARTESIAN_POINT('Ctrl Pts',(-7.56711573212298,1.23190291505985,0.865657016410631));
#64438=CARTESIAN_POINT('Ctrl Pts',(-7.48757210490593,-0.0621854799674716,
1.50435362474225));
#64439=CARTESIAN_POINT('Ctrl Pts',(-7.40802847768887,-1.29914533503867,
0.761031051036168));
#64440=CARTESIAN_POINT('Ctrl Pts',(-7.3284848504718,-1.34260670428284,-0.681435323276333));
#64441=CARTESIAN_POINT('Ctrl Pts',(-7.24894122325475,-0.15264250873053,
-1.4978808786824));
#64442=CARTESIAN_POINT('Ctrl Pts',(-7.16939759603768,1.17755126555268,-0.938253632654406));
#64443=CARTESIAN_POINT('Ctrl Pts',(-7.08985396882063,1.4259525609529,0.483328207438623));
#64444=CARTESIAN_POINT('Ctrl Pts',(-7.01031034160357,0.364360142441329,
1.46088622034507));
#64445=CARTESIAN_POINT('Ctrl Pts',(-6.9307667143865,-1.0319625534079,1.09635767455596));
#64446=CARTESIAN_POINT('Ctrl Pts',(-6.85122308716946,-1.48024216916106,
-0.275372443848858));
#64447=CARTESIAN_POINT('Ctrl Pts',(-6.77167945995239,-0.568653308383513,
-1.39412347984619));
#64448=CARTESIAN_POINT('Ctrl Pts',(-6.69213583273533,0.865345820292249,
-1.23212153357398));
#64449=CARTESIAN_POINT('Ctrl Pts',(-6.61259220551826,1.5043692842901,0.0618054906816298));
#64450=CARTESIAN_POINT('Ctrl Pts',(-6.53304857830121,0.76135918014107,1.29895306343564));
#64451=CARTESIAN_POINT('Ctrl Pts',(-6.45350495108415,-0.681096170171921,
1.34277878638706));
#64452=CARTESIAN_POINT('Ctrl Pts',(-6.37396132386708,-1.49784227466095,
0.15302085620091));
#64453=CARTESIAN_POINT('Ctrl Pts',(-6.29441769665004,-0.938551042447882,
-1.17731423286814));
#64454=CARTESIAN_POINT('Ctrl Pts',(-6.21487406943297,0.482968008178995,
-1.42607460017684));
#64455=CARTESIAN_POINT('Ctrl Pts',(-6.13533044221592,1.46079413937795,-0.364729138612472));
#64456=CARTESIAN_POINT('Ctrl Pts',(-6.05578681499884,1.09661830479939,1.03168558959253));
#64457=CARTESIAN_POINT('Ctrl Pts',(-5.9762431877818,-0.274998538116634,
1.48031167874459));
#64458=CARTESIAN_POINT('Ctrl Pts',(-5.89669956056473,-1.39397979824229,
0.569005434320529));
#64459=CARTESIAN_POINT('Ctrl Pts',(-5.81715593334767,-1.23234007347556,
-0.865034568962549));
#64460=CARTESIAN_POINT('Ctrl Pts',(-5.73761230613061,0.0614254974524097,
-1.50438484785532));
#64461=CARTESIAN_POINT('Ctrl Pts',(-5.65806867891355,1.29876070895606,-0.761687260669268));
#64462=CARTESIAN_POINT('Ctrl Pts',(-5.5785250516965,1.34295078281849,0.680756973611814));
#64463=CARTESIAN_POINT('Ctrl Pts',(-5.49898142447944,0.153399193908172,
1.49780357507327));
#64464=CARTESIAN_POINT('Ctrl Pts',(-5.41943779726237,-1.1770771250679,0.938848392359403));
#64465=CARTESIAN_POINT('Ctrl Pts',(-5.33989417004532,-1.42619654841353,
-0.482607778104791));
#64466=CARTESIAN_POINT('Ctrl Pts',(-5.26035054282825,-0.36509811151294,
-1.46070196520837));
#64467=CARTESIAN_POINT('Ctrl Pts',(-5.1808069156112,1.03140855995292,-1.09687886507572));
#64468=CARTESIAN_POINT('Ctrl Pts',(-5.10126328839413,1.48038109388043,0.274624614838766));
#64469=CARTESIAN_POINT('Ctrl Pts',(-5.02171966117708,0.569357523953502,
1.3938360276989));
#64470=CARTESIAN_POINT('Ctrl Pts',(-4.94217603396002,-0.8647232624414,1.23255853475063));
#64471=CARTESIAN_POINT('Ctrl Pts',(-4.86263240674296,-1.50440031543688,
-0.0610455003040735));
#64472=CARTESIAN_POINT('Ctrl Pts',(-4.7830887795259,-0.762015292599876,
-1.29856827161219));
#64473=CARTESIAN_POINT('Ctrl Pts',(-4.70354515230884,0.680417733617677,
-1.34312269356619));
#64474=CARTESIAN_POINT('Ctrl Pts',(-4.62400152509178,1.49776477992184,-0.15377752182816));
#64475=CARTESIAN_POINT('Ctrl Pts',(-4.54445789787472,0.939145682369963,
1.17683994216708));
#64476=CARTESIAN_POINT('Ctrl Pts',(-4.46491427065766,-0.482247517238938,
1.42631840565522));
#64477=CARTESIAN_POINT('Ctrl Pts',(-4.3853706434406,-1.46060969784225,0.365467061119176));
#64478=CARTESIAN_POINT('Ctrl Pts',(-4.30582701622354,-1.09713935536833,
-1.03113146450678));
#64479=CARTESIAN_POINT('Ctrl Pts',(-4.22628338900648,0.274250674039124,
-1.48045041456411));
#64480=CARTESIAN_POINT('Ctrl Pts',(-4.14673976178942,1.39369216822517,-0.569709577260021));
#64481=CARTESIAN_POINT('Ctrl Pts',(-4.06719613457236,1.23277691738527,0.864411900748698));
#64482=CARTESIAN_POINT('Ctrl Pts',(-3.9876525073553,-0.0606654992609097,
1.5044156870338));
#64483=CARTESIAN_POINT('Ctrl Pts',(-3.90810888013824,-1.29837575141631,
0.762343275911907));
#64484=CARTESIAN_POINT('Ctrl Pts',(-3.82856525292117,-1.34329451861918,
-0.680078450211127));
#64485=CARTESIAN_POINT('Ctrl Pts',(-3.74902162570413,-0.154155839936718,
-1.49772588920915));
#64486=CARTESIAN_POINT('Ctrl Pts',(-3.66947799848706,1.17660268418084,-0.939442912460569));
#64487=CARTESIAN_POINT('Ctrl Pts',(-3.58993437127,1.42644017189407,0.481887225604464));
#64488=CARTESIAN_POINT('Ctrl Pts',(-3.51039074405294,0.365835987407674,
1.46051733728545));
#64489=CARTESIAN_POINT('Ctrl Pts',(-3.43084711683588,-1.03085430327181,
1.09739977566059));
#64490=CARTESIAN_POINT('Ctrl Pts',(-3.35130348961882,-1.48051964079121,
-0.2738767157416));
#64491=CARTESIAN_POINT('Ctrl Pts',(-3.27175986240177,-0.570061594217579,
-1.39354821983028));
#64492=CARTESIAN_POINT('Ctrl Pts',(-3.1922162351847,0.864100483904304,-1.23299522136551));
#64493=CARTESIAN_POINT('Ctrl Pts',(-3.11267260796765,1.50443096264505,0.0602854943470151));
#64494=CARTESIAN_POINT('Ctrl Pts',(-3.03312898075058,0.762671210584582,
1.29818314838084));
#64495=CARTESIAN_POINT('Ctrl Pts',(-2.95358535353353,-0.679739123413961,
1.34346625796621));
#64496=CARTESIAN_POINT('Ctrl Pts',(-2.87404172631646,-1.49768690293735,
0.154534148210354));
#64497=CARTESIAN_POINT('Ctrl Pts',(-2.79449809909941,-0.939740082612886,
-1.17636535112546));
#64498=CARTESIAN_POINT('Ctrl Pts',(-2.71495447188235,0.481526903225423,
-1.42656184712011));
#64499=CARTESIAN_POINT('Ctrl Pts',(-2.63541084466529,1.46042488354174,-0.366204890359183));
#64500=CARTESIAN_POINT('Ctrl Pts',(-2.55586721744823,1.09766012593993,1.03057707627376));
#64501=CARTESIAN_POINT('Ctrl Pts',(-2.47632359023116,-0.273502739977664,
1.48058877254194));
#64502=CARTESIAN_POINT('Ctrl Pts',(-2.39677996301411,-1.39340418250887,
0.570413574832941));
#64503=CARTESIAN_POINT('Ctrl Pts',(-2.31723633579704,-1.23321344670508,
-0.863789011983425));
#64504=CARTESIAN_POINT('Ctrl Pts',(-2.23769270857999,0.0599054856391566,
-1.50444614216461));
#64505=CARTESIAN_POINT('Ctrl Pts',(-2.15814908136293,1.2979904624185,-0.76299909679633));
#64506=CARTESIAN_POINT('Ctrl Pts',(-2.07860545414587,1.34363791178529,0.679399753626298));
#64507=CARTESIAN_POINT('Ctrl Pts',(-1.99906182692881,0.154912446266186,
1.4976478203906));
#64508=CARTESIAN_POINT('Ctrl Pts',(-1.91951819971175,-1.17612794233516,
0.940037194171402));
#64509=CARTESIAN_POINT('Ctrl Pts',(-1.83997457249469,-1.42668343261808,
-0.481166552712769));
#64510=CARTESIAN_POINT('Ctrl Pts',(-1.76043094527763,-0.366573767496878,
-1.46033233170502));
#64511=CARTESIAN_POINT('Ctrl Pts',(-1.68088731806057,1.03029977887392,-1.09792041551294));
#64512=CARTESIAN_POINT('Ctrl Pts',(-1.60134369084351,1.48065781864995,0.27312876446696));
#64513=CARTESIAN_POINT('Ctrl Pts',(-1.52180006362645,0.570765502308645,
1.3932600226829));
#64514=CARTESIAN_POINT('Ctrl Pts',(-1.44225643640939,-0.863477453166383,
1.23343165713992));
#64515=CARTESIAN_POINT('Ctrl Pts',(-1.36271280919234,-1.50446128602429,
-0.0595255941614048));
#64516=CARTESIAN_POINT('Ctrl Pts',(-1.28316918197527,-0.76332681982241,
-1.29779746387891));
#64517=CARTESIAN_POINT('Ctrl Pts',(-1.20362555475822,0.679060123157279,
-1.34380991597466));
#64518=CARTESIAN_POINT('Ctrl Pts',(-1.12408192754115,1.49760905479862,-0.155289906706672));
#64519=CARTESIAN_POINT('Ctrl Pts',(-1.04453830032409,0.94033346279502,1.17588888743665));
#64520=CARTESIAN_POINT('Ctrl Pts',(-0.964994673107034,-0.480804685414002,
1.4268079090415));
#64521=CARTESIAN_POINT('Ctrl Pts',(-0.885451045889976,-1.46024250734839,
0.366936961380079));
#64522=CARTESIAN_POINT('Ctrl Pts',(-0.805907418672918,-1.09817528131783,
-1.03001167307692));
#64523=CARTESIAN_POINT('Ctrl Pts',(-0.726363791455856,0.272744609926045,
-1.48074716033771));
#64524=CARTESIAN_POINT('Ctrl Pts',(-0.646820164238799,1.3931350613471,-0.571078691880378));
#64525=CARTESIAN_POINT('Ctrl Pts',(-0.567276537021739,1.23361317856029,
0.86309237935622));
#64526=CARTESIAN_POINT('Ctrl Pts',(-0.487732909804683,-0.0590761934204603,
1.50461578833112));
#64527=CARTESIAN_POINT('Ctrl Pts',(-0.408189282587616,-1.29773645562838,
0.763389596137374));
#64528=CARTESIAN_POINT('Ctrl Pts',(-0.328645655370557,-1.34372989411186,
-0.678215903148311));
#64529=CARTESIAN_POINT('Ctrl Pts',(-0.249102028153499,-0.15615620871939,
-1.49854272923124));
#64530=CARTESIAN_POINT('Ctrl Pts',(-0.169558400936439,1.17666683856934,
-0.938658107396819));
#64531=CARTESIAN_POINT('Ctrl Pts',(-0.116529316125066,1.34179608678025,
0.00423245967186979));
#64532=CARTESIAN_POINT('Ctrl Pts',(-0.0900147737193787,1.20644987911676,
0.406211384846794));
#64533=CARTESIAN_POINT('Ctrl Pts',(-34.6365,0.684664424539256,-0.958295198918542));
#64534=CARTESIAN_POINT('Ctrl Pts',(-34.6099854575943,1.00396030307469,-0.7301707867521));
#64535=CARTESIAN_POINT('Ctrl Pts',(-34.556956372783,1.39099115610471,0.0663998364373292));
#64536=CARTESIAN_POINT('Ctrl Pts',(-34.4774127455658,0.694817159188923,
1.20840932237519));
#64537=CARTESIAN_POINT('Ctrl Pts',(-34.3978691183489,-0.640240458638742,
1.23665911837698));
#64538=CARTESIAN_POINT('Ctrl Pts',(-34.3183254911317,-1.38682292844981,
0.130635890290045));
#64539=CARTESIAN_POINT('Ctrl Pts',(-34.2387818639147,-0.859516886189572,
-1.09634891418097));
#64540=CARTESIAN_POINT('Ctrl Pts',(-34.1592382366976,0.457492926185055,
-1.31564139210814));
#64541=CARTESIAN_POINT('Ctrl Pts',(-34.0796946094806,1.3541695165413,-0.326543447000047));
#64542=CARTESIAN_POINT('Ctrl Pts',(-34.0001509822635,1.00682106773482,0.962681709799215));
#64543=CARTESIAN_POINT('Ctrl Pts',(-33.9206073550465,-0.265485630343504,
1.36743779586005));
#64544=CARTESIAN_POINT('Ctrl Pts',(-33.8410637278294,-1.29388966381863,
0.515994903012744));
#64545=CARTESIAN_POINT('Ctrl Pts',(-33.7615201006123,-1.13362686059144,
-0.809502282827959));
#64546=CARTESIAN_POINT('Ctrl Pts',(-33.6819764733953,0.0680777368036397,
-1.39131546907066));
#64547=CARTESIAN_POINT('Ctrl Pts',(-33.6024328461782,1.20723976173548,-0.694960952389941));
#64548=CARTESIAN_POINT('Ctrl Pts',(-33.5228892189612,1.23733558104474,0.639843063744817));
#64549=CARTESIAN_POINT('Ctrl Pts',(-33.4433455917441,0.130716022946506,
1.38683466763195));
#64550=CARTESIAN_POINT('Ctrl Pts',(-33.3638019645271,-1.09598955901368,
0.859770194715907));
#64551=CARTESIAN_POINT('Ctrl Pts',(-33.2842583373099,-1.31583182073299,
-0.457148161455002));
#64552=CARTESIAN_POINT('Ctrl Pts',(-33.204714710093,-0.326846022470247,
-1.35409354000658));
#64553=CARTESIAN_POINT('Ctrl Pts',(-33.1251710828758,0.962406571507915,
-1.00706075074908));
#64554=CARTESIAN_POINT('Ctrl Pts',(-33.0456274556588,1.36751576661517,0.26513840054929));
#64555=CARTESIAN_POINT('Ctrl Pts',(-32.9660838284418,0.516315940709615,
1.29376024423113));
#64556=CARTESIAN_POINT('Ctrl Pts',(-32.8865402012247,-0.809212871355991,
1.13383079342446));
#64557=CARTESIAN_POINT('Ctrl Pts',(-32.8069965740076,-1.39133422266715,
-0.0677260339843446));
#64558=CARTESIAN_POINT('Ctrl Pts',(-32.7274529467905,-0.69526502492905,
-1.20706432189118));
#64559=CARTESIAN_POINT('Ctrl Pts',(-32.6479093195736,0.639530057869942,
-1.23749708685117));
#64560=CARTESIAN_POINT('Ctrl Pts',(-32.5683656923564,1.38680183990368,-0.131066360639972));
#64561=CARTESIAN_POINT('Ctrl Pts',(-32.4888220651394,0.860046881755779,
1.09577237368332));
#64562=CARTESIAN_POINT('Ctrl Pts',(-32.4092784379223,-0.456815713582613,
1.31594723981434));
#64563=CARTESIAN_POINT('Ctrl Pts',(-32.3297348107053,-1.35401097246879,
0.327188050574965));
#64564=CARTESIAN_POINT('Ctrl Pts',(-32.2501911834881,-1.00730379652143,
-0.962152168572661));
#64565=CARTESIAN_POINT('Ctrl Pts',(-32.1706475562712,0.264792959390405,
-1.3675826931817));
#64566=CARTESIAN_POINT('Ctrl Pts',(-32.0911039290541,1.29362979082703,-0.516642718223328));
#64567=CARTESIAN_POINT('Ctrl Pts',(-32.011560301837,1.1340351551021,0.808926449684369));
#64568=CARTESIAN_POINT('Ctrl Pts',(-31.93201667462,-0.0673745908983318,
1.39135128508784));
#64569=CARTESIAN_POINT('Ctrl Pts',(-31.8524730474029,-1.20688866591361,
0.695569897350098));
#64570=CARTESIAN_POINT('Ctrl Pts',(-31.7729294201859,-1.23765858699842,
-0.639217455987783));
#64571=CARTESIAN_POINT('Ctrl Pts',(-31.6933857929688,-0.131416651354211,
-1.38676868934885));
#64572=CARTESIAN_POINT('Ctrl Pts',(-31.6138421657517,1.09555509809422,-0.860323637389223));
#64573=CARTESIAN_POINT('Ctrl Pts',(-31.5342985385347,1.31606258565414,0.45648330161381));
#64574=CARTESIAN_POINT('Ctrl Pts',(-31.4547549113176,0.327530052156675,
1.35392828426963));
#64575=CARTESIAN_POINT('Ctrl Pts',(-31.3752112841005,-0.961897701274149,
1.00754679608168));
#64576=CARTESIAN_POINT('Ctrl Pts',(-31.2956676568835,-1.36764953406056,
-0.264447510850282));
#64577=CARTESIAN_POINT('Ctrl Pts',(-31.2161240296664,-0.516969461947962,
-1.29349924987385));
#64578=CARTESIAN_POINT('Ctrl Pts',(-31.1365804024493,0.808639975965988,
-1.13423944706605));
#64579=CARTESIAN_POINT('Ctrl Pts',(-31.0570367752323,1.39136825896598,0.067023144904906));
#64580=CARTESIAN_POINT('Ctrl Pts',(-30.9774931480152,0.695874725271205,
1.20671293220041));
#64581=CARTESIAN_POINT('Ctrl Pts',(-30.8979495207982,-0.638904813258247,
1.23782000856604));
#64582=CARTESIAN_POINT('Ctrl Pts',(-30.8184058935811,-1.38673545034811,
0.131766933480272));
#64583=CARTESIAN_POINT('Ctrl Pts',(-30.7388622663641,-0.860600338114134,
-1.09533775249866));
#64584=CARTESIAN_POINT('Ctrl Pts',(-30.659318639147,0.456150860510873,-1.31617784758222));
#64585=CARTESIAN_POINT('Ctrl Pts',(-30.57977501193,1.35384550969123,-0.327872032811375));
#64586=CARTESIAN_POINT('Ctrl Pts',(-30.5002313847129,1.00778973135526,0.961643172588391));
#64587=CARTESIAN_POINT('Ctrl Pts',(-30.4206877574958,-0.264102045436351,
1.3677162876881));
#64588=CARTESIAN_POINT('Ctrl Pts',(-30.3411441302788,-1.2933686263928,0.517296172684261));
#64589=CARTESIAN_POINT('Ctrl Pts',(-30.2616005030617,-1.13444366666221,
-0.808353450651991));
#64590=CARTESIAN_POINT('Ctrl Pts',(-30.1820568758447,0.0666716946350309,
-1.39138514407244));
#64591=CARTESIAN_POINT('Ctrl Pts',(-30.1025132486276,1.2065371214959,-0.696179508793066));
#64592=CARTESIAN_POINT('Ctrl Pts',(-30.0229696214105,1.23798135115748,0.638592129764595));
#64593=CARTESIAN_POINT('Ctrl Pts',(-29.9434259941935,0.132117207199287,
1.38670212287024));
#64594=CARTESIAN_POINT('Ctrl Pts',(-29.8638823669764,-1.09512033701773,
0.860876983930424));
#64595=CARTESIAN_POINT('Ctrl Pts',(-29.7843387397594,-1.31629302553474,
-0.455818390304285));
#64596=CARTESIAN_POINT('Ctrl Pts',(-29.7047951125423,-0.328213992546994,
-1.35376264873402));
#64597=CARTESIAN_POINT('Ctrl Pts',(-29.6252514853253,0.96138858254731,-1.00803260232924));
#64598=CARTESIAN_POINT('Ctrl Pts',(-29.5457078581082,1.3677829540518,0.263756563172021));
#64599=CARTESIAN_POINT('Ctrl Pts',(-29.4661642308912,0.517622850415724,
1.29323792039148));
#64600=CARTESIAN_POINT('Ctrl Pts',(-29.386620603674,-0.808066873762948,
1.13464781387793));
#64601=CARTESIAN_POINT('Ctrl Pts',(-29.3070769764571,-1.39140194040491,
-0.066320240111329));
#64602=CARTESIAN_POINT('Ctrl Pts',(-29.2275333492399,-0.696484247896873,
-1.20636123381121));
#64603=CARTESIAN_POINT('Ctrl Pts',(-29.1479897220229,0.638279405527112,
-1.23814261476251));
#64604=CARTESIAN_POINT('Ctrl Pts',(-29.0684460948058,1.38666870691719,-0.132467472488888));
#64605=CARTESIAN_POINT('Ctrl Pts',(-28.9889024675888,0.86115357482053,1.0949028516653));
#64606=CARTESIAN_POINT('Ctrl Pts',(-28.9093588403717,-0.455485891015299,
1.31640811950435));
#64607=CARTESIAN_POINT('Ctrl Pts',(-28.8298152131546,-1.35367970140324,
0.328555931341711));
#64608=CARTESIAN_POINT('Ctrl Pts',(-28.7502715859376,-1.00827540898812,
-0.961133931167149));
#64609=CARTESIAN_POINT('Ctrl Pts',(-28.6707279587205,0.26341106407934,-1.3678495331474));
#64610=CARTESIAN_POINT('Ctrl Pts',(-28.5911843315035,1.29310713187823,-0.517949495121513));
#64611=CARTESIAN_POINT('Ctrl Pts',(-28.5116407042864,1.13485188870017,0.807780245317151));
#64612=CARTESIAN_POINT('Ctrl Pts',(-28.4320970770694,-0.0659687813562216,
1.39141864796234));
#64613=CARTESIAN_POINT('Ctrl Pts',(-28.3525534498523,-1.20618526915755,
0.696788942563181));
#64614=CARTESIAN_POINT('Ctrl Pts',(-28.2730098226353,-1.23830379937083,
-0.637966640565749));
#64615=CARTESIAN_POINT('Ctrl Pts',(-28.1934661954182,-0.132817729326718,
-1.38663520249108));
#64616=CARTESIAN_POINT('Ctrl Pts',(-28.1139225682011,1.09468529645522,-0.861430110766812));
#64617=CARTESIAN_POINT('Ctrl Pts',(-28.0343789409841,1.31652312948372,0.455153362665139));
#64618=CARTESIAN_POINT('Ctrl Pts',(-27.954835313767,0.32889784917371,1.35359666770419));
#64619=CARTESIAN_POINT('Ctrl Pts',(-27.8752916865499,-0.960879218464155,
1.00851815131642));
#64620=CARTESIAN_POINT('Ctrl Pts',(-27.7957480593329,-1.36791602497067,
-0.26306554818035));
#64621=CARTESIAN_POINT('Ctrl Pts',(-27.7162044321158,-0.51827610678078,
-1.2929762608614));
#64622=CARTESIAN_POINT('Ctrl Pts',(-27.6366608048988,0.807493565332879,
-1.13505589111593));
#64623=CARTESIAN_POINT('Ctrl Pts',(-27.5571171776817,1.39143526674366,0.0656173183921381));
#64624=CARTESIAN_POINT('Ctrl Pts',(-27.4775735504646,0.697093592772551,
1.20600922754614));
#64625=CARTESIAN_POINT('Ctrl Pts',(-27.3980299232476,-0.637653834900464,
1.23846490497216));
#64626=CARTESIAN_POINT('Ctrl Pts',(-27.3184862960305,-1.38660160959405,
0.133167977690434));
#64627=CARTESIAN_POINT('Ctrl Pts',(-27.2389426688135,-0.861706591751621,
-1.09446767140139));
#64628=CARTESIAN_POINT('Ctrl Pts',(-27.1593990415964,0.454820805275012,
-1.3166380554655));
#64629=CARTESIAN_POINT('Ctrl Pts',(-27.0798554143794,1.35351354764217,-0.329239746021173));
#64630=CARTESIAN_POINT('Ctrl Pts',(-27.0003117871623,1.00876082929865,0.960624444454579));
#64631=CARTESIAN_POINT('Ctrl Pts',(-26.9207681599452,-0.262720015497096,
1.36798242951735));
#64632=CARTESIAN_POINT('Ctrl Pts',(-26.8412245327282,-1.29284530734934,
0.518602685372692));
#64633=CARTESIAN_POINT('Ctrl Pts',(-26.761680905511,-1.13525982111218,-0.807206833828431));
#64634=CARTESIAN_POINT('Ctrl Pts',(-26.6821372782941,0.065265851241496,
-1.39145179674781));
#64635=CARTESIAN_POINT('Ctrl Pts',(-26.6025936510769,1.20583310898822,-0.697398198505544));
#64636=CARTESIAN_POINT('Ctrl Pts',(-26.52305002386,1.23862593155623,0.637340988551213));
#64637=CARTESIAN_POINT('Ctrl Pts',(-26.4435063966428,0.133518217557687,
1.38656792822826));
#64638=CARTESIAN_POINT('Ctrl Pts',(-26.3639627694258,-1.09424997651769,
0.861983017757319));
#64639=CARTESIAN_POINT('Ctrl Pts',(-26.2844191422087,-1.31675289744237,
-0.454488218866141));
#64640=CARTESIAN_POINT('Ctrl Pts',(-26.2048755149917,-0.329581621862289,
-1.35343034122248));
#64641=CARTESIAN_POINT('Ctrl Pts',(-26.1253318877746,0.960369609154678,
-1.00900344291933));
#64642=CARTESIAN_POINT('Ctrl Pts',(-26.0457882605576,1.36804874678321,0.262374466051626));
#64643=CARTESIAN_POINT('Ctrl Pts',(-25.9662446333405,0.518929230876408,
1.2927142713504));
#64644=CARTESIAN_POINT('Ctrl Pts',(-25.8867010061234,-0.806920050822095,
1.13546367867592));
#64645=CARTESIAN_POINT('Ctrl Pts',(-25.8071573789064,-1.39146823797373,
-0.0649143799267269));
#64646=CARTESIAN_POINT('Ctrl Pts',(-25.7276137516893,-0.697702759742729,
-1.20565691349503));
#64647=CARTESIAN_POINT('Ctrl Pts',(-25.6480701244723,0.637028101537958,
-1.23878687911276));
#64648=CARTESIAN_POINT('Ctrl Pts',(-25.5685264972552,1.38653415839583,-0.133868448906134));
#64649=CARTESIAN_POINT('Ctrl Pts',(-25.4889828700381,0.862259388766268,
1.09403221181801));
#64650=CARTESIAN_POINT('Ctrl Pts',(-25.4094392428211,-0.454155603459752,
1.31686765540699));
#64651=CARTESIAN_POINT('Ctrl Pts',(-25.329895615604,-1.35334704845044,0.329923476675237));
#64652=CARTESIAN_POINT('Ctrl Pts',(-25.250351988387,-1.00924599216297,-0.960114712580717));
#64653=CARTESIAN_POINT('Ctrl Pts',(-25.1708083611699,0.262028899865992,
-1.36811497676401));
#64654=CARTESIAN_POINT('Ctrl Pts',(-25.0912647339529,1.29258315287295,-0.519255743271084));
#64655=CARTESIAN_POINT('Ctrl Pts',(-25.0117211067357,1.13566746379413,0.806633216332175));
#64656=CARTESIAN_POINT('Ctrl Pts',(-24.9321774795188,-0.0645629044702633,
1.39148459042037));
#64657=CARTESIAN_POINT('Ctrl Pts',(-24.8526338523016,-1.20548064107781,
0.698007276464662));
#64658=CARTESIAN_POINT('Ctrl Pts',(-24.7730902250846,-1.23894774763147,
-0.63671517388067));
#64659=CARTESIAN_POINT('Ctrl Pts',(-24.6935465978676,-0.134218671713418,
-1.38650030009895));
#64660=CARTESIAN_POINT('Ctrl Pts',(-24.6140029706505,1.09381437731624,-0.862535704760827));
#64661=CARTESIAN_POINT('Ctrl Pts',(-24.5344593434334,1.31698232935204,0.453822959077054));
#64662=CARTESIAN_POINT('Ctrl Pts',(-24.4549157162164,0.330265310438215,
1.35326366933134));
#64663=CARTESIAN_POINT('Ctrl Pts',(-24.3753720889993,-0.959859754748951,
1.00948847701412));
#64664=CARTESIAN_POINT('Ctrl Pts',(-24.2958284617822,-1.36818111945554,
-0.261683316962251));
#64665=CARTESIAN_POINT('Ctrl Pts',(-24.2162848345652,-0.519582222535895,
-1.29245195192535));
#64666=CARTESIAN_POINT('Ctrl Pts',(-24.1367412073481,0.806346330376981,
-1.13587117645381));
#64667=CARTESIAN_POINT('Ctrl Pts',(-24.057197580131,1.39150085408669,0.0642114248945288));
#64668=CARTESIAN_POINT('Ctrl Pts',(-23.977653952914,0.698311748651915,1.20530429174781));
#64669=CARTESIAN_POINT('Ctrl Pts',(-23.8981103256969,-0.636402205599313,
1.2391085371021));
#64670=CARTESIAN_POINT('Ctrl Pts',(-23.8185666984799,-1.38646635333975,
0.134568885957192));
#64671=CARTESIAN_POINT('Ctrl Pts',(-23.7390230712628,-0.862811965723368,
-1.0935964730263));
#64672=CARTESIAN_POINT('Ctrl Pts',(-23.6594794440458,0.453490285739293,
-1.31709691927021));
#64673=CARTESIAN_POINT('Ctrl Pts',(-23.5799358168287,1.35318020387053,-0.330607123129397));
#64674=CARTESIAN_POINT('Ctrl Pts',(-23.5003921896117,1.00973089745727,0.959604735675643));
#64675=CARTESIAN_POINT('Ctrl Pts',(-23.4208485623946,-0.261337717362417,
1.36824717485357));
#64676=CARTESIAN_POINT('Ctrl Pts',(-23.3413049351776,-1.29232066851596,
0.519908668650037));
#64677=CARTESIAN_POINT('Ctrl Pts',(-23.2617613079605,-1.13607481664197,
-0.806059392974791));
#64678=CARTESIAN_POINT('Ctrl Pts',(-23.1822176807434,0.063859941221911,
-1.39151702897166));
#64679=CARTESIAN_POINT('Ctrl Pts',(-23.1026740535264,1.20512786551627,-0.698616176285083));
#64680=CARTESIAN_POINT('Ctrl Pts',(-23.0231304263093,1.23926924751441,0.636089196713827));
#64681=CARTESIAN_POINT('Ctrl Pts',(-22.9435867990922,0.134919091615136,
1.38643231812041));
#64682=CARTESIAN_POINT('Ctrl Pts',(-22.8640431718752,-1.09337849896205,
0.863088171636293));
#64683=CARTESIAN_POINT('Ctrl Pts',(-22.7844995446581,-1.31721142515419,
-0.453157583467666));
#64684=CARTESIAN_POINT('Ctrl Pts',(-22.7049559174411,-0.330948914727013,
-1.35309665207331));
#64685=CARTESIAN_POINT('Ctrl Pts',(-22.625412290224,0.959349655377068,-1.00997325347698));
#64686=CARTESIAN_POINT('Ctrl Pts',(-22.5458686630069,1.36831314295389,0.260992101088554));
#64687=CARTESIAN_POINT('Ctrl Pts',(-22.4663250357899,0.520235081592649,
1.29218930265316));
#64688=CARTESIAN_POINT('Ctrl Pts',(-22.3867814085728,-0.805772404143914,
1.13627838434563));
#64689=CARTESIAN_POINT('Ctrl Pts',(-22.3072377813558,-1.39153311507424,
-0.0635084534748757));
#64690=CARTESIAN_POINT('Ctrl Pts',(-22.2276941541387,-0.69892055934474,
-1.20495136239444));
#64691=CARTESIAN_POINT('Ctrl Pts',(-22.1481505269216,0.635776147244211,
-1.23942987885813));
#64692=CARTESIAN_POINT('Ctrl Pts',(-22.0686068997046,1.38639819444309,-0.135269288664905));
#64693=CARTESIAN_POINT('Ctrl Pts',(-21.9890632724875,0.863364322481949,
1.09316045513743));
#64694=CARTESIAN_POINT('Ctrl Pts',(-21.9095196452704,-0.4528248522834,1.31732584699667));
#64695=CARTESIAN_POINT('Ctrl Pts',(-21.8299760180534,-1.35301301394502,
0.331290685209222));
#64696=CARTESIAN_POINT('Ctrl Pts',(-21.7504323908363,-1.01021554505779,
-0.959094513869495));
#64697=CARTESIAN_POINT('Ctrl Pts',(-21.6708887636193,0.260646468162729,
-1.36837902375229));
#64698=CARTESIAN_POINT('Ctrl Pts',(-21.5913451364022,1.29205785434534,-0.520561461342927));
#64699=CARTESIAN_POINT('Ctrl Pts',(-21.5118015091852,1.13648187955178,0.805485363902682));
#64700=CARTESIAN_POINT('Ctrl Pts',(-21.4322578819681,-0.0631569616758272,
1.3915491123934));
#64701=CARTESIAN_POINT('Ctrl Pts',(-21.352714254751,-1.2047747823936,0.699224897811445));
#64702=CARTESIAN_POINT('Ctrl Pts',(-21.273170627534,-1.23959043112302,-0.635463057210422));
#64703=CARTESIAN_POINT('Ctrl Pts',(-21.1936270003169,-0.135619477084131,
-1.38636398230999));
#64704=CARTESIAN_POINT('Ctrl Pts',(-21.1140833730999,1.09294234156633,-0.863640418242735));
#64705=CARTESIAN_POINT('Ctrl Pts',(-21.0345397458828,1.31744018479035,0.452492092207748));
#64706=CARTESIAN_POINT('Ctrl Pts',(-20.9549961186657,0.331632434554235,
1.352929289491));
#64707=CARTESIAN_POINT('Ctrl Pts',(-20.8754524914487,-0.958839311169214,
1.01045777218423));
#64708=CARTESIAN_POINT('Ctrl Pts',(-20.7959088642316,-1.36844481724457,
-0.260300818606975));
#64709=CARTESIAN_POINT('Ctrl Pts',(-20.7163652370146,-0.520887807880025,
-1.29192632360089));
#64710=CARTESIAN_POINT('Ctrl Pts',(-20.6368216097975,0.80519827226939,-1.13668530224745));
#64711=CARTESIAN_POINT('Ctrl Pts',(-20.5572779825804,1.39156502092812,0.06280546584721));
#64712=CARTESIAN_POINT('Ctrl Pts',(-20.4777343553634,0.699529191665802,
1.20459812552501));
#64713=CARTESIAN_POINT('Ctrl Pts',(-20.3981907281463,-0.635149926632454,
1.23975090429883));
#64714=CARTESIAN_POINT('Ctrl Pts',(-20.3186471009293,-1.38632968172327,
0.135969656850494));
#64715=CARTESIAN_POINT('Ctrl Pts',(-20.2391034737122,-0.863916458901017,
-1.09272415826269));
#64716=CARTESIAN_POINT('Ctrl Pts',(-20.1595598464952,0.452159303261918,
-1.31755443852794));
#64717=CARTESIAN_POINT('Ctrl Pts',(-20.0800162192781,1.35284547871658,-0.331974162740232));
#64718=CARTESIAN_POINT('Ctrl Pts',(-20.0004725920611,1.01069993484086,0.958584047292498));
#64719=CARTESIAN_POINT('Ctrl Pts',(-19.920928964844,-0.259955152443364,
1.36851052342652));
#64720=CARTESIAN_POINT('Ctrl Pts',(-19.8413853376269,-1.29179471042819,
0.521214121183144));
#64721=CARTESIAN_POINT('Ctrl Pts',(-19.7618417104099,-1.13688865241964,
-0.804911129262371));
#64722=CARTESIAN_POINT('Ctrl Pts',(-19.6822980831928,0.0624539660114313,
-1.3915808406774));
#64723=CARTESIAN_POINT('Ctrl Pts',(-19.6027544559757,1.20442139179994,-0.699833440888375));
#64724=CARTESIAN_POINT('Ctrl Pts',(-19.5232108287587,1.23991129837533,0.634836755530266));
#64725=CARTESIAN_POINT('Ctrl Pts',(-19.4436672015416,0.13631982794163,1.38629529268513));
#64726=CARTESIAN_POINT('Ctrl Pts',(-19.3641235743245,-1.09250590524041,
0.864192444439202));
#64727=CARTESIAN_POINT('Ctrl Pts',(-19.2845799471075,-1.31766860820214,
-0.451826485467164));
#64728=CARTESIAN_POINT('Ctrl Pts',(-19.2050363198904,-0.332315869745427,
-1.35276158162712));
#64729=CARTESIAN_POINT('Ctrl Pts',(-19.1254926926734,0.958328722255644,
-1.0109420330122));
#64730=CARTESIAN_POINT('Ctrl Pts',(-19.0459490654563,1.36857614229396,0.25960946969393));
#64731=CARTESIAN_POINT('Ctrl Pts',(-18.9664054382392,0.521540401231442,
1.29166301483565));
#64732=CARTESIAN_POINT('Ctrl Pts',(-18.8868618110222,-0.804623934899931,
1.13709193005541));
#64733=CARTESIAN_POINT('Ctrl Pts',(-18.8073181838051,-1.39159657164021,
-0.0621024621909377));
#64734=CARTESIAN_POINT('Ctrl Pts',(-18.7277745565881,-0.700137645459773,
-1.20424458122967));
#64735=CARTESIAN_POINT('Ctrl Pts',(-18.648230929371,0.63452354392386,-1.24007161334226));
#64736=CARTESIAN_POINT('Ctrl Pts',(-18.5686873021539,1.38626081519776,-0.136669990335221));
#64737=CARTESIAN_POINT('Ctrl Pts',(-18.4891436749369,0.864468374839663,
1.09228758251344));
#64738=CARTESIAN_POINT('Ctrl Pts',(-18.4096000477198,-0.451493638844702,
1.31778269380568));
#64739=CARTESIAN_POINT('Ctrl Pts',(-18.3300564205028,-1.35267759822798,
0.332657555548002));
#64740=CARTESIAN_POINT('Ctrl Pts',(-18.2505127932857,-1.01118406668283,
-0.958073336074932));
#64741=CARTESIAN_POINT('Ctrl Pts',(-18.1709691660687,0.259263770380752,
-1.36864167384269));
#64742=CARTESIAN_POINT('Ctrl Pts',(-18.0914255388516,1.29153123683166,-0.521866648004122));
#64743=CARTESIAN_POINT('Ctrl Pts',(-18.0118819116345,1.13729513514176,0.804336689200407));
#64744=CARTESIAN_POINT('Ctrl Pts',(-17.9323382844175,-0.0617509544081363,
1.39161221381557));
#64745=CARTESIAN_POINT('Ctrl Pts',(-17.8527946572004,-1.20406769382548,
0.700441805360565));
#64746=CARTESIAN_POINT('Ctrl Pts',(-17.7732510299834,-1.24023184918943,
-0.634210291833199));
#64747=CARTESIAN_POINT('Ctrl Pts',(-17.6937074027663,-0.137020144008901,
-1.38622624926336));
#64748=CARTESIAN_POINT('Ctrl Pts',(-17.6141637755493,1.09206919009568,-0.864744250084811));
#64749=CARTESIAN_POINT('Ctrl Pts',(-17.5346201483322,1.31789669533126,0.451160763415784));
#64750=CARTESIAN_POINT('Ctrl Pts',(-17.4550765211151,0.332999220126171,
1.35259352852449));
#64751=CARTESIAN_POINT('Ctrl Pts',(-17.3755328938981,-0.957817888766664,
1.0114260358373));
#64752=CARTESIAN_POINT('Ctrl Pts',(-17.295989266681,-1.36870711806855,-0.258918054525863));
#64753=CARTESIAN_POINT('Ctrl Pts',(-17.2164456394639,-0.522192861480347,
-1.29139937642464));
#64754=CARTESIAN_POINT('Ctrl Pts',(-17.1369020122469,0.804049392182112,
-1.13749826766574));
#64755=CARTESIAN_POINT('Ctrl Pts',(-17.0573583850298,1.39162776720246,0.0613994426854746));
#64756=CARTESIAN_POINT('Ctrl Pts',(-16.9778147578128,0.700745920571368,
1.20389072959865));
#64757=CARTESIAN_POINT('Ctrl Pts',(-16.8982711305957,-0.63389699927829,
1.24039200590658));
#64758=CARTESIAN_POINT('Ctrl Pts',(-16.8187275033786,-1.38619159488414,
0.137370288940351));
#64759=CARTESIAN_POINT('Ctrl Pts',(-16.7391838761616,-0.865020070157029,
-1.09185072800109));
#64760=CARTESIAN_POINT('Ctrl Pts',(-16.6596402489445,0.450827859201633,
-1.31801061277163));
#64761=CARTESIAN_POINT('Ctrl Pts',(-16.5800966217275,1.35250937252205,-0.333340863458119));
#64762=CARTESIAN_POINT('Ctrl Pts',(-16.5005529945104,1.01166794046017,0.957562380347131));
#64763=CARTESIAN_POINT('Ctrl Pts',(-16.4210093672934,-0.258572322151341,
1.36877247496735));
#64764=CARTESIAN_POINT('Ctrl Pts',(-16.3414657400763,-1.29126743362299,
0.522519041639328));
#64765=CARTESIAN_POINT('Ctrl Pts',(-16.2619221128592,-1.13770132761438,
-0.803762043863395));
#64766=CARTESIAN_POINT('Ctrl Pts',(-16.1823784856422,0.061047927045359,
-1.39164323179989));
#64767=CARTESIAN_POINT('Ctrl Pts',(-16.1028348584251,1.20371368856048,-0.701049991072757));
#64768=CARTESIAN_POINT('Ctrl Pts',(-16.0232912312081,1.24055208348352,0.633583666279101));
#64769=CARTESIAN_POINT('Ctrl Pts',(-15.943747603991,0.13772042510721,1.3861568520623));
#64770=CARTESIAN_POINT('Ctrl Pts',(-15.8642039767739,-1.09163219624359,
0.865295835038735));
#64771=CARTESIAN_POINT('Ctrl Pts',(-15.7846603495569,-1.31812444611951,
-0.450494926223506));
#64772=CARTESIAN_POINT('Ctrl Pts',(-15.7051167223398,-0.333682485522065,
-1.352425130226));
#64773=CARTESIAN_POINT('Ctrl Pts',(-15.6255730951227,0.957306810832643,
-1.011909780536));
#64774=CARTESIAN_POINT('Ctrl Pts',(-15.5460294679057,1.36883774453492,0.258226573279226));
#64775=CARTESIAN_POINT('Ctrl Pts',(-15.4664858406886,0.52284518846023,1.29113540843514));
#64776=CARTESIAN_POINT('Ctrl Pts',(-15.3869422134716,-0.803474644262568,
1.13790431497473));
#64777=CARTESIAN_POINT('Ctrl Pts',(-15.3073985862545,-1.39165860760688,
-0.0606964075102383));
#64778=CARTESIAN_POINT('Ctrl Pts',(-15.2278549590375,-0.70135401684535,
-1.20353657072225));
#64779=CARTESIAN_POINT('Ctrl Pts',(-15.1483113318204,0.633270292855629,
-1.24071208191002));
#64780=CARTESIAN_POINT('Ctrl Pts',(-15.0687677046033,1.38612202080006,-0.138070552487189));
#64781=CARTESIAN_POINT('Ctrl Pts',(-14.9892240773863,0.865571544712346,
1.09141359483712));
#64782=CARTESIAN_POINT('Ctrl Pts',(-14.9096804501692,-0.45016196450262,
1.31823819536764));
#64783=CARTESIAN_POINT('Ctrl Pts',(-14.8301368229522,-1.35234080164171,
0.334024086296205));
#64784=CARTESIAN_POINT('Ctrl Pts',(-14.7505931957351,-1.01215155604939,
-0.957051180239471));
#64785=CARTESIAN_POINT('Ctrl Pts',(-14.6710495685181,0.25788080793157,-1.36890292676711));
#64786=CARTESIAN_POINT('Ctrl Pts',(-14.591505941301,1.2910033008695,-0.523171301922277));
#64787=CARTESIAN_POINT('Ctrl Pts',(-14.5119623140839,1.13810722973384,0.803187193397973));
#64788=CARTESIAN_POINT('Ctrl Pts',(-14.4324186868668,-0.0603448841024907,
1.39167389462245));
#64789=CARTESIAN_POINT('Ctrl Pts',(-14.3528750596498,-1.20335937609527,
0.701657997869762));
#64790=CARTESIAN_POINT('Ctrl Pts',(-14.2733314324327,-1.2408720011759,-0.632956879027886));
#64791=CARTESIAN_POINT('Ctrl Pts',(-14.1937878052157,-0.138420671057853,
-1.38608710109966));
#64792=CARTESIAN_POINT('Ctrl Pts',(-14.1142441779986,1.09119492379563,-0.865847199160223));
#64793=CARTESIAN_POINT('Ctrl Pts',(-14.0347005507816,1.31835186050876,0.449828974060237));
#64794=CARTESIAN_POINT('Ctrl Pts',(-13.9551569235645,0.334365665758747,
1.3522563867746));
#64795=CARTESIAN_POINT('Ctrl Pts',(-13.8756132963474,-0.956795488584001,
1.01239326698485));
#64796=CARTESIAN_POINT('Ctrl Pts',(-13.7960696691304,-1.36896802165973,
-0.257535026130468));
#64797=CARTESIAN_POINT('Ctrl Pts',(-13.7165260419133,-0.523497382004637,
-1.29087111093451));
#64798=CARTESIAN_POINT('Ctrl Pts',(-13.6369824146963,0.802899691287971,
-1.13831007187878));
#64799=CARTESIAN_POINT('Ctrl Pts',(-13.5574387874792,1.39168909284562,0.05999335684464));
#64800=CARTESIAN_POINT('Ctrl Pts',(-13.4778951602621,0.701961934126549,
1.20318210469084));
#64801=CARTESIAN_POINT('Ctrl Pts',(-13.3983515330451,-0.632643424815839,
1.24103184127092));
#64802=CARTESIAN_POINT('Ctrl Pts',(-13.318807905828,-1.38605209296332,0.138770780796948));
#64803=CARTESIAN_POINT('Ctrl Pts',(-13.2392642786109,-0.866122798364796,
-1.09097618313311));
#64804=CARTESIAN_POINT('Ctrl Pts',(-13.1597206513939,0.449495954917602,
-1.3184654415356));
#64805=CARTESIAN_POINT('Ctrl Pts',(-13.0801770241768,1.35217188563002,-0.334707223887899));
#64806=CARTESIAN_POINT('Ctrl Pts',(-13.0006333969598,1.01263491332703,0.956539735882493));
#64807=CARTESIAN_POINT('Ctrl Pts',(-12.9210897697427,-0.25718922789799,
1.36903302920864));
#64808=CARTESIAN_POINT('Ctrl Pts',(-12.8415461425257,-1.29073883863859,
0.523823428686496));
#64809=CARTESIAN_POINT('Ctrl Pts',(-12.7620025153086,-1.13851284139658,
-0.802612137950876));
#64810=CARTESIAN_POINT('Ctrl Pts',(-12.6824588880915,0.0596418257590296,
-1.39170420227544));
#64811=CARTESIAN_POINT('Ctrl Pts',(-12.6029152608745,1.2030047565203,-0.702265825596333));
#64812=CARTESIAN_POINT('Ctrl Pts',(-12.5233716336574,1.24119160218488,0.632329930239507));
#64813=CARTESIAN_POINT('Ctrl Pts',(-12.4438280064404,0.139120881682115,
1.38601699639326));
#64814=CARTESIAN_POINT('Ctrl Pts',(-12.3642843792233,-1.09075737286348,
0.86639834230852));
#64815=CARTESIAN_POINT('Ctrl Pts',(-12.2847407520063,-1.31857893844094,
-0.449162907095992));
#64816=CARTESIAN_POINT('Ctrl Pts',(-12.2051971247892,-0.335048760661853,
-1.35208729821336));
#64817=CARTESIAN_POINT('Ctrl Pts',(-12.1256534975721,0.956283922151258,
-1.01287649506048));
#64818=CARTESIAN_POINT('Ctrl Pts',(-12.0461098703551,1.36909794940973,0.256843413256152));
#64819=CARTESIAN_POINT('Ctrl Pts',(-11.966566243138,0.524149441947044,1.29060648399021));
#64820=CARTESIAN_POINT('Ctrl Pts',(-11.887022615921,-0.802324533405046,
1.1387155382743));
#64821=CARTESIAN_POINT('Ctrl Pts',(-11.8074789887039,-1.39171922291092,
-0.0592902908681086));
#64822=CARTESIAN_POINT('Ctrl Pts',(-11.7279353614868,-0.702569672259767,
-1.20282733159494));
#64823=CARTESIAN_POINT('Ctrl Pts',(-11.6483917342698,0.632016395318918,
-1.2413512839076));
#64824=CARTESIAN_POINT('Ctrl Pts',(-11.5688481070527,1.38598181139171,-0.139470973691));
#64825=CARTESIAN_POINT('Ctrl Pts',(-11.4893044798357,0.866673830973786,
1.09053849300069));
#64826=CARTESIAN_POINT('Ctrl Pts',(-11.4097608526186,-0.448829830616605,
1.31869235121755));
#64827=CARTESIAN_POINT('Ctrl Pts',(-11.3302172254015,-1.35200262453006,
0.335390276058804));
#64828=CARTESIAN_POINT('Ctrl Pts',(-11.2506735981845,-1.01311801216977,
-0.956028047406628));
#64829=CARTESIAN_POINT('Ctrl Pts',(-11.1711299709674,0.256497582227027,
-1.36916278225881));
#64830=CARTESIAN_POINT('Ctrl Pts',(-11.0915863437504,1.2904740469978,-0.52447542176553));
#64831=CARTESIAN_POINT('Ctrl Pts',(-11.0120427165333,1.13891816249902,0.802036877668863));
#64832=CARTESIAN_POINT('Ctrl Pts',(-10.9324990893162,-0.0589387521943207,
1.39173415475109));
#64833=CARTESIAN_POINT('Ctrl Pts',(-10.8529554620992,-1.20264982992607,
0.702873474097439));
#64834=CARTESIAN_POINT('Ctrl Pts',(-10.7734118348821,-1.24151088642892,
-0.631702820074028));
#64835=CARTESIAN_POINT('Ctrl Pts',(-10.6938682076651,-0.139821056801252,
-1.38594653796095));
#64836=CARTESIAN_POINT('Ctrl Pts',(-10.614324580448,1.09031954355872,-0.866949264343001));
#64837=CARTESIAN_POINT('Ctrl Pts',(-10.534780953231,1.31880567985816,0.4484967255007));
#64838=CARTESIAN_POINT('Ctrl Pts',(-10.4552373260139,0.335731770057017,
1.35191786458549));
#64839=CARTESIAN_POINT('Ctrl Pts',(-10.3756936987968,-0.955772111664961,
1.0133594646395));
#64840=CARTESIAN_POINT('Ctrl Pts',(-10.2961500715798,-1.36922752775175,
-0.256151734832699));
#64841=CARTESIAN_POINT('Ctrl Pts',(-10.2166064443627,-0.524801368121128,
-1.29034152766978));
#64842=CARTESIAN_POINT('Ctrl Pts',(-10.1370628171456,0.801749170760637,
-1.13912071405783));
#64843=CARTESIAN_POINT('Ctrl Pts',(-10.0575191899286,1.39174899779504,0.0585872097601163));
#64844=CARTESIAN_POINT('Ctrl Pts',(-9.97797556271153,0.703177231089948,
1.20247225152501));
#64845=CARTESIAN_POINT('Ctrl Pts',(-9.89843193549446,-0.63138920452485,
1.24167040973862));
#64846=CARTESIAN_POINT('Ctrl Pts',(-9.8188883082774,-1.38591117610322,0.140171130990584));
#64847=CARTESIAN_POINT('Ctrl Pts',(-9.73934468106035,-0.867224642398599,
-1.09010052455156));
#64848=CARTESIAN_POINT('Ctrl Pts',(-9.65980105384327,0.448163591769547,
-1.31891892435554));
#64849=CARTESIAN_POINT('Ctrl Pts',(-9.58025742662623,1.35183301838504,-0.33607324263468));
#64850=CARTESIAN_POINT('Ctrl Pts',(-9.50071379940917,1.0136008524543,0.955516114942553));
#64851=CARTESIAN_POINT('Ctrl Pts',(-9.42117017219209,-0.255805871095256,
1.36929218588443));
#64852=CARTESIAN_POINT('Ctrl Pts',(-9.34162654497505,-1.29020892601463,
0.525127280993029));
#64853=CARTESIAN_POINT('Ctrl Pts',(-9.26208291775799,-1.13932319293779,
-0.801461412698725));
#64854=CARTESIAN_POINT('Ctrl Pts',(-9.18253929054092,0.0582356635878705,
-1.3917637520418));
#64855=CARTESIAN_POINT('Ctrl Pts',(-9.10299566332388,1.20229459640314,-0.703480943217913));
#64856=CARTESIAN_POINT('Ctrl Pts',(-9.02345203610679,1.24182985382652,0.631075548691406));
#64857=CARTESIAN_POINT('Ctrl Pts',(-8.94390840888976,0.140521196236644,
1.38587572582076));
#64858=CARTESIAN_POINT('Ctrl Pts',(-8.86436478167268,-1.08988143599316,
0.867499965123046));
#64859=CARTESIAN_POINT('Ctrl Pts',(-8.78482115445563,-1.31903208470249,
-0.447830429444425));
#64860=CARTESIAN_POINT('Ctrl Pts',(-8.70527752723856,-0.336414693769986,
-1.35174808593414));
#64861=CARTESIAN_POINT('Ctrl Pts',(-8.62573390002151,0.955260057255724,
-1.01384217559874));
#64862=CARTESIAN_POINT('Ctrl Pts',(-8.54619027280444,1.36935675665274,0.255459991036712));
#64863=CARTESIAN_POINT('Ctrl Pts',(-8.46664664558739,0.525453160360428,
1.29007624204083));
#64864=CARTESIAN_POINT('Ctrl Pts',(-8.38710301837033,-0.801173603501495,
1.13952559912596));
#64865=CARTESIAN_POINT('Ctrl Pts',(-8.30755939115328,-1.39177841749043,
-0.0578841137000273));
#64866=CARTESIAN_POINT('Ctrl Pts',(-8.2280157639362,-0.703784610462002,
-1.20211686457176));
#64867=CARTESIAN_POINT('Ctrl Pts',(-8.14847213671916,0.630761852593739,
-1.24198921868246));
#64868=CARTESIAN_POINT('Ctrl Pts',(-8.06892850950209,1.38584018711583,-0.140871252517076));
#64869=CARTESIAN_POINT('Ctrl Pts',(-7.98938488228504,0.867775232498749,
1.08966227789749));
#64870=CARTESIAN_POINT('Ctrl Pts',(-7.90984125506796,-0.447497238546542,
1.31914516089179));
#64871=CARTESIAN_POINT('Ctrl Pts',(-7.83029762785092,-1.35166306723823,
0.336756123441143));
#64872=CARTESIAN_POINT('Ctrl Pts',(-7.75075400063385,-1.01408343405741,
-0.955003938620828));
#64873=CARTESIAN_POINT('Ctrl Pts',(-7.6712103734168,0.255114094679148,-1.36942124005254));
#64874=CARTESIAN_POINT('Ctrl Pts',(-7.59166674619974,1.28994347575683,-0.525779006202587));
#64875=CARTESIAN_POINT('Ctrl Pts',(-7.51212311898267,1.13972793260945,0.800885743187348));
#64876=CARTESIAN_POINT('Ctrl Pts',(-7.43257949176562,-0.0575325601190364,
1.39179299413997));
#64877=CARTESIAN_POINT('Ctrl Pts',(-7.35303586454856,-1.2019390560422,0.704088232802815));
#64878=CARTESIAN_POINT('Ctrl Pts',(-7.27349223733148,-1.2421485042963,-0.630448116251818));
#64879=CARTESIAN_POINT('Ctrl Pts',(-7.19394861011444,-0.141221299809534,
-1.38580455999072));
#64880=CARTESIAN_POINT('Ctrl Pts',(-7.11440498289737,1.08944305027853,-0.868050444508131));
#64881=CARTESIAN_POINT('Ctrl Pts',(-7.03486135568032,1.3192581529162,0.447164019097165));
#64882=CARTESIAN_POINT('Ctrl Pts',(-6.95531772846325,0.337097531626415,
1.35157796230272));
#64883=CARTESIAN_POINT('Ctrl Pts',(-6.8757741012462,-0.954747759054236,
1.01432462781492));
#64884=CARTESIAN_POINT('Ctrl Pts',(-6.79623047402913,-1.3694856360797,-0.254768182044651));
#64885=CARTESIAN_POINT('Ctrl Pts',(-6.71668684681209,-0.526104818498686,
-1.28981062717108));
#64886=CARTESIAN_POINT('Ctrl Pts',(-6.63714321959501,0.800597831774603,
-1.13993019337537));
#64887=CARTESIAN_POINT('Ctrl Pts',(-6.55759959237797,1.39180748198953,0.0571810028673485));
#64888=CARTESIAN_POINT('Ctrl Pts',(-6.47805596516089,0.704391810220957,
1.2017611708258));
#64889=CARTESIAN_POINT('Ctrl Pts',(-6.39851233794385,-0.630134339685656,
1.24230771065784));
#64890=CARTESIAN_POINT('Ctrl Pts',(-6.31896871072677,-1.3857688444477,0.141571338091734));
#64891=CARTESIAN_POINT('Ctrl Pts',(-6.23942508350973,-0.868325601133633,
-1.08922375315032));
#64892=CARTESIAN_POINT('Ctrl Pts',(-6.15988145629266,0.446830771117568,
-1.31937106076852));
#64893=CARTESIAN_POINT('Ctrl Pts',(-6.08033782907561,1.35149277113303,-0.337438918303999));
#64894=CARTESIAN_POINT('Ctrl Pts',(-6.00079420185854,1.01456575685592,0.954491518572258));
#64895=CARTESIAN_POINT('Ctrl Pts',(-5.92125057464148,-0.254422253155312,
1.36954994473014));
#64896=CARTESIAN_POINT('Ctrl Pts',(-5.84170694742441,-1.28967769629207,
0.526430597227924));
#64897=CARTESIAN_POINT('Ctrl Pts',(-5.76216332020736,-1.14013238141078,
-0.80030986928163));
#64898=CARTESIAN_POINT('Ctrl Pts',(-5.68261969299031,0.0568294419673366,
-1.39182188103819));
#64899=CARTESIAN_POINT('Ctrl Pts',(-5.60307606577323,1.20158320893396,-0.704695342697066));
#64900=CARTESIAN_POINT('Ctrl Pts',(-5.52353243855619,1.24246683775691,0.629820522915297));
#64901=CARTESIAN_POINT('Ctrl Pts',(-5.44398881133912,0.141921367341324,
1.38573304048903));
#64902=CARTESIAN_POINT('Ctrl Pts',(-5.36444518412207,-1.08900438652681,
0.868600702357744));
#64903=CARTESIAN_POINT('Ctrl Pts',(-5.284901556905,-1.31948388444155,-0.446497494629042));
#64904=CARTESIAN_POINT('Ctrl Pts',(-5.20535792968794,-0.337780283452094,
-1.35140749373458));
#64905=CARTESIAN_POINT('Ctrl Pts',(-5.12581430247089,0.954235217191234,
-1.01480682116499));
#64906=CARTESIAN_POINT('Ctrl Pts',(-5.04627067525382,1.36961416599977,0.254076308033152));
#64907=CARTESIAN_POINT('Ctrl Pts',(-4.96672704803676,0.526756342369506,
1.2895446831283));
#64908=CARTESIAN_POINT('Ctrl Pts',(-4.88718342081971,-0.800021855726812,
1.14033449670278));
#64909=CARTESIAN_POINT('Ctrl Pts',(-4.80763979360265,-1.39183619128499,
-0.0564778774414496));
#64910=CARTESIAN_POINT('Ctrl Pts',(-4.72809616638559,-0.704998830211815,
-1.20140517037799));
#64911=CARTESIAN_POINT('Ctrl Pts',(-4.64855253916853,0.629506665960787,
-1.24262588558339));
#64912=CARTESIAN_POINT('Ctrl Pts',(-4.56900891195147,1.38569714811699,-0.142271387535955));
#64913=CARTESIAN_POINT('Ctrl Pts',(-4.48946528473441,0.868875748162881,
1.08878495042198));
#64914=CARTESIAN_POINT('Ctrl Pts',(-4.40992165751735,-0.446164189652799,
1.31959662392811));
#64915=CARTESIAN_POINT('Ctrl Pts',(-4.33037803030028,-1.35132213011286,
0.338121627048909));
#64916=CARTESIAN_POINT('Ctrl Pts',(-4.25083440308323,-1.01504782072675,
-0.953978854927527));
#64917=CARTESIAN_POINT('Ctrl Pts',(-4.17129077586617,0.253730346700255,
-1.36967829988445));
#64918=CARTESIAN_POINT('Ctrl Pts',(-4.09174714864911,1.28941158768824,-0.527082053902699));
#64919=CARTESIAN_POINT('Ctrl Pts',(-4.01220352143205,1.14053653923849,0.799733791128557));
#64920=CARTESIAN_POINT('Ctrl Pts',(-3.93265989421499,-0.0561263093121601,
1.39185041272904));
#64921=CARTESIAN_POINT('Ctrl Pts',(-3.85311626699793,-1.20122705516927,
0.705302272745785));
#64922=CARTESIAN_POINT('Ctrl Pts',(-3.77357263978087,-1.24278485412711,
-0.629192768842119));
#64923=CARTESIAN_POINT('Ctrl Pts',(-3.69402901256381,-0.142621398653279,
-1.3856611673339));
#64924=CARTESIAN_POINT('Ctrl Pts',(-3.61448538534675,1.08856544484988,-0.869150738531468));
#64925=CARTESIAN_POINT('Ctrl Pts',(-3.53494175812969,1.31970927922097,0.445830856210143));
#64926=CARTESIAN_POINT('Ctrl Pts',(-3.45539813091263,0.338462949072693,
1.35123668027329));
#64927=CARTESIAN_POINT('Ctrl Pts',(-3.37585450369557,-0.95372243179753,
1.01528875552582));
#64928=CARTESIAN_POINT('Ctrl Pts',(-3.29631087647852,-1.36974234638011,
-0.253384369178725));
#64929=CARTESIAN_POINT('Ctrl Pts',(-3.21676724926146,-0.527407731806677,
-1.28927840998041));
#64930=CARTESIAN_POINT('Ctrl Pts',(-3.13722362204439,0.799445675505238,
-1.14073850900496));
#64931=CARTESIAN_POINT('Ctrl Pts',(-3.05767999482733,1.39186454536937,0.0557747376017607));
#64932=CARTESIAN_POINT('Ctrl Pts',(-2.97813636761027,0.705605670279753,
1.20104886331929));
#64933=CARTESIAN_POINT('Ctrl Pts',(-2.89859274039321,-0.62887883157946,
1.24294374337767));
#64934=CARTESIAN_POINT('Ctrl Pts',(-2.81904911317616,-1.38562509814175,
0.142971400671562));
#64935=CARTESIAN_POINT('Ctrl Pts',(-2.7395054859591,-0.869425673446542,
-1.08834586982554));
#64936=CARTESIAN_POINT('Ctrl Pts',(-2.65996185874204,0.445497494323327,
-1.31982185031089));
#64937=CARTESIAN_POINT('Ctrl Pts',(-2.58041823152498,1.35115114421937,-0.338804249505638));
#64938=CARTESIAN_POINT('Ctrl Pts',(-2.50087460430792,1.01552962555056,0.953465947825067));
#64939=CARTESIAN_POINT('Ctrl Pts',(-2.42133097709085,-0.253038375497675,
1.36980630546842));
#64940=CARTESIAN_POINT('Ctrl Pts',(-2.3417873498738,-1.28914514999981,0.527733376087698));
#64941=CARTESIAN_POINT('Ctrl Pts',(-2.26224372265673,-1.14094040601493,
-0.799157508926434));
#64942=CARTESIAN_POINT('Ctrl Pts',(-2.18270009543968,0.0554231623812737,
-1.39187858910792));
#64943=CARTESIAN_POINT('Ctrl Pts',(-2.10315646822262,1.2008705947473,-0.7059090229788));
#64944=CARTESIAN_POINT('Ctrl Pts',(-2.02361284100557,1.24310255349976,0.628564854542996));
#64945=CARTESIAN_POINT('Ctrl Pts',(-1.9440692137885,0.143321393236571,1.38558893987825));
#64946=CARTESIAN_POINT('Ctrl Pts',(-1.86452558657144,-1.08812622473303,
0.869700554151995));
#64947=CARTESIAN_POINT('Ctrl Pts',(-1.78498195935438,-1.31993433838648,
-0.445164106407946));
#64948=CARTESIAN_POINT('Ctrl Pts',(-1.70543833213732,-0.339145526056245,
-1.35106551741206));
#64949=CARTESIAN_POINT('Ctrl Pts',(-1.62589470492026,0.9532093987185,-1.01577043941121));
#64950=CARTESIAN_POINT('Ctrl Pts',(-1.5463510777032,1.36987018532208,0.25269238205091));
#64951=CARTESIAN_POINT('Ctrl Pts',(-1.46680745048614,0.528058971205146,
1.28901177668085));
#64952=CARTESIAN_POINT('Ctrl Pts',(-1.38726382326908,-0.798869261953324,
1.14114228923538));
#64953=CARTESIAN_POINT('Ctrl Pts',(-1.30772019605202,-1.39189259985476,
-0.0550716956193558));
#64954=CARTESIAN_POINT('Ctrl Pts',(-1.22817656883496,-0.70621222470226,
-1.20069203698611));
#64955=CARTESIAN_POINT('Ctrl Pts',(-1.14863294161791,0.628250636330202,
-1.24326168777629));
#64956=CARTESIAN_POINT('Ctrl Pts',(-1.06908931440084,1.38555307485394,-0.143670610859339));
#64957=CARTESIAN_POINT('Ctrl Pts',(-0.989545687183782,0.869974654993682,
1.08790505669946));
#64958=CARTESIAN_POINT('Ctrl Pts',(-0.910002059966723,-0.444829315197323,
1.32004950107908));
#64959=CARTESIAN_POINT('Ctrl Pts',(-0.830458432749666,-1.35098241400592,
0.33948154459194));
#64960=CARTESIAN_POINT('Ctrl Pts',(-0.750914805532605,-1.01600623532771,
-0.952942849934193));
#64961=CARTESIAN_POINT('Ctrl Pts',(-0.671371178315547,0.252336971202078,
-1.36995284217421));
#64962=CARTESIAN_POINT('Ctrl Pts',(-0.591827551098487,1.28889616535859,
-0.528348726914579));
#64963=CARTESIAN_POINT('Ctrl Pts',(-0.512283923881428,1.14131022863273,
0.798513000617958));
#64964=CARTESIAN_POINT('Ctrl Pts',(-0.432740296664372,-0.0546559205033708,
1.39203554179653));
#64965=CARTESIAN_POINT('Ctrl Pts',(-0.353196669447305,-1.20063559357129,
0.70627030388918));
#64966=CARTESIAN_POINT('Ctrl Pts',(-0.273653042230246,-1.24318765340952,
-0.627469583607843));
#64967=CARTESIAN_POINT('Ctrl Pts',(-0.194109415013188,-0.144472093338112,
-1.38641688872905));
#64968=CARTESIAN_POINT('Ctrl Pts',(-0.114565787796129,1.08862479899838,
-0.868424655134898));
#64969=CARTESIAN_POINT('Ctrl Pts',(-0.0615367029847556,1.24139853983146,
0.00391577327447434));
#64970=CARTESIAN_POINT('Ctrl Pts',(-0.0350221605790679,1.11617937559294,
0.375817327967939));
#64971=CARTESIAN_POINT('Ctrl Pts',(-0.200000000000004,1.38699088616444,
0.466999498604424));
#64972=CARTESIAN_POINT('Ctrl Pts',(-0.22651454240569,1.54259118067784,0.00486583246659934));
#64973=CARTESIAN_POINT('Ctrl Pts',(-0.253029084811376,1.44767104919453,
-0.537129589727037));
#64974=CARTESIAN_POINT('Ctrl Pts',(-0.279543627217062,1.14483175725401,
-0.915405533876346));
#64975=CARTESIAN_POINT('Ctrl Pts',(-0.306058169622748,0.841992465313498,
-1.29368147802566));
#64976=CARTESIAN_POINT('Ctrl Pts',(-0.332572712028434,0.331234012915777,
-1.50823794413064));
#64977=CARTESIAN_POINT('Ctrl Pts',(-0.35908725443412,-0.151693535955519,
-1.45833519918207));
#64978=CARTESIAN_POINT('Ctrl Pts',(-0.385601796839806,-0.634621084826815,
-1.4084324542335));
#64979=CARTESIAN_POINT('Ctrl Pts',(-0.412116339245492,-1.08971773017168,
-1.09407049823137));
#64980=CARTESIAN_POINT('Ctrl Pts',(-0.438630881651178,-1.30845335354846,
-0.660666733086481));
#64981=CARTESIAN_POINT('Ctrl Pts',(-0.451035572486509,-1.41078767790324,
-0.457901034503743));
#64982=CARTESIAN_POINT('Ctrl Pts',(-0.463440263321839,-1.46138759520564,
-0.229079612523116));
#64983=CARTESIAN_POINT('Ctrl Pts',(-0.47584495415717,-1.4610556053668,-0.000134560743048767));
#64984=CARTESIAN_POINT('Origin',(-0.2,0.,0.));
#64985=CARTESIAN_POINT('',(0.,-2.03719995038162E-16,1.6635));
#64986=CARTESIAN_POINT('Origin',(-0.2,-2.03719995038162E-16,1.6635));
#64987=CARTESIAN_POINT('Origin',(0.,0.,0.));
#64988=CARTESIAN_POINT('Origin',(-0.2,0.,0.));
#64989=CARTESIAN_POINT('Origin',(-17.3,0.,0.));
#64990=CARTESIAN_POINT('Origin',(0.,2.75,0.));
#64991=CARTESIAN_POINT('',(0.,-2.75,-3.36777869765522E-16));
#64992=CARTESIAN_POINT('Origin',(0.,0.,0.));
#64993=CARTESIAN_POINT('Origin',(0.3,2.77916773064255,-0.363113928340879));
#64994=CARTESIAN_POINT('',(2.6,2.72200415854531,-0.391399234621183));
#64995=CARTESIAN_POINT('',(0.3,2.72200415854531,-0.391399234621183));
#64996=CARTESIAN_POINT('',(1.35,2.72200415854531,-0.391399234621183));
#64997=CARTESIAN_POINT('',(2.6,2.59004439042211,-0.456694707264027));
#64998=CARTESIAN_POINT('',(2.6,2.77916773064255,-0.363113928340879));
#64999=CARTESIAN_POINT('',(0.3,2.59004439042211,-0.456694707264027));
#65000=CARTESIAN_POINT('',(0.3,2.59004439042211,-0.456694707264027));
#65001=CARTESIAN_POINT('',(0.3,2.77916773064255,-0.363113928340879));
#65002=CARTESIAN_POINT('Origin',(0.3,2.67375304942814,-0.471454802365716));
#65003=CARTESIAN_POINT('',(0.3,2.69171364385628,-0.563185279883955));
#65004=CARTESIAN_POINT('Origin',(0.3,0.,0.));
#65005=CARTESIAN_POINT('',(0.3,2.59004439042211,-0.456694707264027));
#65006=CARTESIAN_POINT('Origin',(0.3,2.59004439042211,-0.456694707264027));
#65007=CARTESIAN_POINT('',(2.6,2.69171364385628,-0.563185279883955));
#65008=CARTESIAN_POINT('',(1.35,2.69171364385628,-0.563185279883955));
#65009=CARTESIAN_POINT('',(2.6,2.59004439042211,-0.456694707264027));
#65010=CARTESIAN_POINT('Origin',(2.6,2.67375304942814,-0.471454802365716));
#65011=CARTESIAN_POINT('Origin',(2.6,0.,0.));
#65012=CARTESIAN_POINT('Origin',(0.3,2.67389185611625,-0.840194823713636));
#65013=CARTESIAN_POINT('',(2.6,2.61268503523469,-0.858124062511185));
#65014=CARTESIAN_POINT('',(0.3,2.61268503523469,-0.858124062511185));
#65015=CARTESIAN_POINT('',(1.35,2.61268503523469,-0.858124062511185));
#65016=CARTESIAN_POINT('',(2.6,2.47139159266694,-0.899512976946511));
#65017=CARTESIAN_POINT('',(2.6,2.67389185611625,-0.840194823713636));
#65018=CARTESIAN_POINT('',(0.3,2.47139159266694,-0.899512976946511));
#65019=CARTESIAN_POINT('',(0.3,2.47139159266694,-0.899512976946511));
#65020=CARTESIAN_POINT('',(0.3,2.67389185611625,-0.840194823713636));
#65021=CARTESIAN_POINT('Origin',(0.3,2.55126546543374,-0.928584689129192));
#65022=CARTESIAN_POINT('',(0.3,2.55302436781771,-1.02204039906893));
#65023=CARTESIAN_POINT('Origin',(0.3,0.,0.));
#65024=CARTESIAN_POINT('',(0.3,2.47139159266694,-0.899512976946511));
#65025=CARTESIAN_POINT('Origin',(0.3,2.47139159266694,-0.899512976946511));
#65026=CARTESIAN_POINT('',(2.6,2.55302436781771,-1.02204039906893));
#65027=CARTESIAN_POINT('',(1.35,2.55302436781771,-1.02204039906893));
#65028=CARTESIAN_POINT('',(2.6,2.47139159266694,-0.899512976946511));
#65029=CARTESIAN_POINT('Origin',(2.6,2.55126546543374,-0.928584689129192));
#65030=CARTESIAN_POINT('Origin',(2.6,0.,0.));
#65031=CARTESIAN_POINT('Origin',(0.3,2.48737113059643,-1.29174682452695));
#65032=CARTESIAN_POINT('',(2.6,2.42398079921089,-1.29877522499351));
#65033=CARTESIAN_POINT('',(0.3,2.42398079921089,-1.29877522499351));
#65034=CARTESIAN_POINT('',(1.35,2.42398079921089,-1.29877522499351));
#65035=CARTESIAN_POINT('',(2.6,2.27764681195307,-1.315));
#65036=CARTESIAN_POINT('',(2.6,2.48737113059643,-1.29174682452695));
#65037=CARTESIAN_POINT('',(0.3,2.27764681195307,-1.315));
#65038=CARTESIAN_POINT('',(0.3,2.27764681195307,-1.315));
#65039=CARTESIAN_POINT('',(0.3,2.48737113059643,-1.29174682452695));
#65040=CARTESIAN_POINT('Origin',(0.3,2.35125897127475,-1.3575));
#65041=CARTESIAN_POINT('',(0.3,2.33676273825567,-1.44984133790558));
#65042=CARTESIAN_POINT('Origin',(0.3,0.,0.));
#65043=CARTESIAN_POINT('',(0.3,2.27764681195307,-1.315));
#65044=CARTESIAN_POINT('Origin',(0.3,2.27764681195307,-1.315));
#65045=CARTESIAN_POINT('',(2.6,2.33676273825567,-1.44984133790558));
#65046=CARTESIAN_POINT('',(1.35,2.33676273825567,-1.44984133790558));
#65047=CARTESIAN_POINT('',(2.6,2.27764681195307,-1.315));
#65048=CARTESIAN_POINT('Origin',(2.6,2.35125897127475,-1.3575));
#65049=CARTESIAN_POINT('Origin',(2.6,0.,0.));
#65050=CARTESIAN_POINT('Origin',(0.3,2.22527289194396,-1.70404975173244));
#65051=CARTESIAN_POINT('',(2.6,2.16162513319653,-1.69996375947638));
#65052=CARTESIAN_POINT('',(0.3,2.16162513319653,-1.69996375947638));
#65053=CARTESIAN_POINT('',(1.35,2.16162513319653,-1.69996375947638));
#65054=CARTESIAN_POINT('',(2.6,2.01469688540291,-1.6905314134756));
#65055=CARTESIAN_POINT('',(2.6,2.22527289194396,-1.70404975173244));
#65056=CARTESIAN_POINT('',(0.3,2.01469688540291,-1.6905314134756));
#65057=CARTESIAN_POINT('',(0.3,2.01469688540291,-1.6905314134756));
#65058=CARTESIAN_POINT('',(0.3,2.22527289194396,-1.70404975173244));
#65059=CARTESIAN_POINT('Origin',(0.3,2.07981066306802,-1.74516836029895));
#65060=CARTESIAN_POINT('',(0.3,2.04949975535074,-1.83358958134509));
#65061=CARTESIAN_POINT('Origin',(0.3,0.,0.));
#65062=CARTESIAN_POINT('',(0.3,2.01469688540291,-1.6905314134756));
#65063=CARTESIAN_POINT('Origin',(0.3,2.01469688540291,-1.6905314134756));
#65064=CARTESIAN_POINT('',(2.6,2.04949975535074,-1.83358958134509));
#65065=CARTESIAN_POINT('',(1.35,2.04949975535074,-1.83358958134509));
#65066=CARTESIAN_POINT('',(2.6,2.01469688540291,-1.6905314134756));
#65067=CARTESIAN_POINT('Origin',(2.6,2.07981066306802,-1.74516836029895));
#65068=CARTESIAN_POINT('Origin',(2.6,0.,0.));
#65069=CARTESIAN_POINT('Origin',(0.3,1.89556086251218,-2.06457598952232));
#65070=CARTESIAN_POINT('',(2.6,1.83358958134509,-2.04949975535074));
#65071=CARTESIAN_POINT('',(0.3,1.83358958134509,-2.04949975535074));
#65072=CARTESIAN_POINT('',(1.35,1.83358958134509,-2.04949975535074));
#65073=CARTESIAN_POINT('',(2.6,1.6905314134756,-2.01469688540291));
#65074=CARTESIAN_POINT('',(2.6,1.89556086251218,-2.06457598952232));
#65075=CARTESIAN_POINT('',(0.3,1.6905314134756,-2.01469688540291));
#65076=CARTESIAN_POINT('',(0.3,1.6905314134756,-2.01469688540291));
#65077=CARTESIAN_POINT('',(0.3,1.89556086251218,-2.06457598952232));
#65078=CARTESIAN_POINT('Origin',(0.3,1.74516836029895,-2.07981066306803));
#65079=CARTESIAN_POINT('',(0.3,1.69996375947638,-2.16162513319653));
#65080=CARTESIAN_POINT('Origin',(0.3,0.,0.));
#65081=CARTESIAN_POINT('',(0.3,1.6905314134756,-2.01469688540291));
#65082=CARTESIAN_POINT('Origin',(0.3,1.6905314134756,-2.01469688540291));
#65083=CARTESIAN_POINT('',(2.6,1.69996375947638,-2.16162513319653));
#65084=CARTESIAN_POINT('',(1.35,1.69996375947638,-2.16162513319653));
#65085=CARTESIAN_POINT('',(2.6,1.6905314134756,-2.01469688540291));
#65086=CARTESIAN_POINT('Origin',(2.6,1.74516836029895,-2.07981066306803));
#65087=CARTESIAN_POINT('Origin',(2.6,0.,0.));
#65088=CARTESIAN_POINT('Origin',(0.3,1.50825317547306,-2.36237113059643));
#65089=CARTESIAN_POINT('',(2.6,1.44984133790558,-2.33676273825567));
#65090=CARTESIAN_POINT('',(0.3,1.44984133790558,-2.33676273825567));
#65091=CARTESIAN_POINT('',(1.35,1.44984133790558,-2.33676273825567));
#65092=CARTESIAN_POINT('',(2.6,1.315,-2.27764681195307));
#65093=CARTESIAN_POINT('',(2.6,1.50825317547306,-2.36237113059643));
#65094=CARTESIAN_POINT('',(0.3,1.315,-2.27764681195307));
#65095=CARTESIAN_POINT('',(0.3,1.315,-2.27764681195307));
#65096=CARTESIAN_POINT('',(0.3,1.50825317547306,-2.36237113059643));
#65097=CARTESIAN_POINT('Origin',(0.3,1.3575,-2.35125897127475));
#65098=CARTESIAN_POINT('',(0.3,1.29877522499351,-2.42398079921089));
#65099=CARTESIAN_POINT('Origin',(0.3,0.,0.));
#65100=CARTESIAN_POINT('',(0.3,1.315,-2.27764681195307));
#65101=CARTESIAN_POINT('Origin',(0.3,1.315,-2.27764681195307));
#65102=CARTESIAN_POINT('',(2.6,1.29877522499351,-2.42398079921089));
#65103=CARTESIAN_POINT('',(1.35,1.29877522499351,-2.42398079921089));
#65104=CARTESIAN_POINT('',(2.6,1.315,-2.27764681195307));
#65105=CARTESIAN_POINT('Origin',(2.6,1.3575,-2.35125897127475));
#65106=CARTESIAN_POINT('Origin',(2.6,0.,0.));
#65107=CARTESIAN_POINT('Origin',(0.3,1.07511797891011,-2.58838682028484));
#65108=CARTESIAN_POINT('',(2.6,1.02204039906892,-2.55302436781771));
#65109=CARTESIAN_POINT('',(0.3,1.02204039906892,-2.55302436781771));
#65110=CARTESIAN_POINT('',(1.35,1.02204039906892,-2.55302436781771));
#65111=CARTESIAN_POINT('',(2.6,0.899512976946507,-2.47139159266694));
#65112=CARTESIAN_POINT('',(2.6,1.07511797891011,-2.58838682028484));
#65113=CARTESIAN_POINT('',(0.3,0.899512976946507,-2.47139159266694));
#65114=CARTESIAN_POINT('',(0.3,0.899512976946507,-2.47139159266694));
#65115=CARTESIAN_POINT('',(0.3,1.07511797891011,-2.58838682028484));
#65116=CARTESIAN_POINT('Origin',(0.3,0.928584689129189,-2.55126546543374));
#65117=CARTESIAN_POINT('',(0.3,0.858124062511182,-2.61268503523469));
#65118=CARTESIAN_POINT('Origin',(0.3,0.,0.));
#65119=CARTESIAN_POINT('',(0.3,0.899512976946507,-2.47139159266694));
#65120=CARTESIAN_POINT('Origin',(0.3,0.899512976946507,-2.47139159266694));
#65121=CARTESIAN_POINT('',(2.6,0.858124062511182,-2.61268503523469));
#65122=CARTESIAN_POINT('',(1.35,0.858124062511182,-2.61268503523469));
#65123=CARTESIAN_POINT('',(2.6,0.899512976946507,-2.47139159266694));
#65124=CARTESIAN_POINT('Origin',(2.6,0.928584689129189,-2.55126546543374));
#65125=CARTESIAN_POINT('Origin',(2.6,0.,0.));
#65126=CARTESIAN_POINT('Origin',(0.3,0.60931586659393,-2.73575568622582));
#65127=CARTESIAN_POINT('',(2.6,0.563185279883954,-2.69171364385628));
#65128=CARTESIAN_POINT('',(0.3,0.563185279883954,-2.69171364385628));
#65129=CARTESIAN_POINT('',(1.35,0.563185279883954,-2.69171364385628));
#65130=CARTESIAN_POINT('',(2.6,0.456694707264026,-2.59004439042211));
#65131=CARTESIAN_POINT('',(2.6,0.60931586659393,-2.73575568622582));
#65132=CARTESIAN_POINT('',(0.3,0.456694707264026,-2.59004439042211));
#65133=CARTESIAN_POINT('',(0.3,0.456694707264026,-2.59004439042211));
#65134=CARTESIAN_POINT('',(0.3,0.60931586659393,-2.73575568622582));
#65135=CARTESIAN_POINT('Origin',(0.3,0.471454802365715,-2.67375304942814));
#65136=CARTESIAN_POINT('',(0.3,0.391399234621181,-2.72200415854531));
#65137=CARTESIAN_POINT('Origin',(0.3,0.,0.));
#65138=CARTESIAN_POINT('',(0.3,0.456694707264026,-2.59004439042211));
#65139=CARTESIAN_POINT('Origin',(0.3,0.456694707264026,-2.59004439042211));
#65140=CARTESIAN_POINT('',(2.6,0.391399234621181,-2.72200415854531));
#65141=CARTESIAN_POINT('',(1.35,0.391399234621181,-2.72200415854531));
#65142=CARTESIAN_POINT('',(2.6,0.456694707264026,-2.59004439042211));
#65143=CARTESIAN_POINT('Origin',(2.6,0.471454802365715,-2.67375304942814));
#65144=CARTESIAN_POINT('Origin',(2.6,0.,0.));
#65145=CARTESIAN_POINT('Origin',(0.3,0.124999999999999,-2.8));
#65146=CARTESIAN_POINT('',(2.6,0.0872180609552139,-2.74861656289909));
#65147=CARTESIAN_POINT('',(0.3,0.0872180609552139,-2.74861656289909));
#65148=CARTESIAN_POINT('',(1.35,0.0872180609552139,-2.74861656289909));
#65149=CARTESIAN_POINT('',(2.6,-4.83123162263631E-16,-2.63));
#65150=CARTESIAN_POINT('',(2.6,0.124999999999999,-2.8));
#65151=CARTESIAN_POINT('',(0.3,-4.83123162263631E-16,-2.63));
#65152=CARTESIAN_POINT('',(0.3,-4.83123162263631E-16,-2.63));
#65153=CARTESIAN_POINT('',(0.3,0.124999999999999,-2.8));
#65154=CARTESIAN_POINT('Origin',(0.3,-4.9873740895276E-16,-2.715));
#65155=CARTESIAN_POINT('',(0.3,-0.0872180609552148,-2.74861656289909));
#65156=CARTESIAN_POINT('Origin',(0.3,0.,0.));
#65157=CARTESIAN_POINT('',(0.3,-4.83123162263631E-16,-2.63));
#65158=CARTESIAN_POINT('Origin',(0.3,-4.83123162263631E-16,-2.63));
#65159=CARTESIAN_POINT('',(2.6,-0.0872180609552148,-2.74861656289909));
#65160=CARTESIAN_POINT('',(1.35,-0.0872180609552148,-2.74861656289909));
#65161=CARTESIAN_POINT('',(2.6,-4.83123162263631E-16,-2.63));
#65162=CARTESIAN_POINT('Origin',(2.6,-4.9873740895276E-16,-2.715));
#65163=CARTESIAN_POINT('Origin',(2.6,0.,0.));
#65164=CARTESIAN_POINT('Origin',(0.3,-0.363113928340879,-2.77916773064255));
#65165=CARTESIAN_POINT('',(2.6,-0.391399234621183,-2.72200415854531));
#65166=CARTESIAN_POINT('',(0.3,-0.391399234621183,-2.72200415854531));
#65167=CARTESIAN_POINT('',(1.35,-0.391399234621183,-2.72200415854531));
#65168=CARTESIAN_POINT('',(2.6,-0.456694707264027,-2.59004439042211));
#65169=CARTESIAN_POINT('',(2.6,-0.363113928340879,-2.77916773064255));
#65170=CARTESIAN_POINT('',(0.3,-0.456694707264027,-2.59004439042211));
#65171=CARTESIAN_POINT('',(0.3,-0.456694707264027,-2.59004439042211));
#65172=CARTESIAN_POINT('',(0.3,-0.363113928340879,-2.77916773064255));
#65173=CARTESIAN_POINT('Origin',(0.3,-0.471454802365716,-2.67375304942814));
#65174=CARTESIAN_POINT('',(0.3,-0.563185279883955,-2.69171364385628));
#65175=CARTESIAN_POINT('Origin',(0.3,0.,0.));
#65176=CARTESIAN_POINT('',(0.3,-0.456694707264027,-2.59004439042211));
#65177=CARTESIAN_POINT('Origin',(0.3,-0.456694707264027,-2.59004439042211));
#65178=CARTESIAN_POINT('',(2.6,-0.563185279883955,-2.69171364385628));
#65179=CARTESIAN_POINT('',(1.35,-0.563185279883955,-2.69171364385628));
#65180=CARTESIAN_POINT('',(2.6,-0.456694707264027,-2.59004439042211));
#65181=CARTESIAN_POINT('Origin',(2.6,-0.471454802365716,-2.67375304942814));
#65182=CARTESIAN_POINT('Origin',(2.6,0.,0.));
#65183=CARTESIAN_POINT('Origin',(0.3,-0.840194823713636,-2.67389185611625));
#65184=CARTESIAN_POINT('',(2.6,-0.858124062511185,-2.61268503523469));
#65185=CARTESIAN_POINT('',(0.3,-0.858124062511185,-2.61268503523469));
#65186=CARTESIAN_POINT('',(1.35,-0.858124062511185,-2.61268503523469));
#65187=CARTESIAN_POINT('',(2.6,-0.89951297694651,-2.47139159266694));
#65188=CARTESIAN_POINT('',(2.6,-0.840194823713636,-2.67389185611625));
#65189=CARTESIAN_POINT('',(0.3,-0.89951297694651,-2.47139159266694));
#65190=CARTESIAN_POINT('',(0.3,-0.89951297694651,-2.47139159266694));
#65191=CARTESIAN_POINT('',(0.3,-0.840194823713636,-2.67389185611625));
#65192=CARTESIAN_POINT('Origin',(0.3,-0.928584689129192,-2.55126546543374));
#65193=CARTESIAN_POINT('',(0.3,-1.02204039906893,-2.55302436781771));
#65194=CARTESIAN_POINT('Origin',(0.3,0.,0.));
#65195=CARTESIAN_POINT('',(0.3,-0.89951297694651,-2.47139159266694));
#65196=CARTESIAN_POINT('Origin',(0.3,-0.89951297694651,-2.47139159266694));
#65197=CARTESIAN_POINT('',(2.6,-1.02204039906893,-2.55302436781771));
#65198=CARTESIAN_POINT('',(1.35,-1.02204039906893,-2.55302436781771));
#65199=CARTESIAN_POINT('',(2.6,-0.89951297694651,-2.47139159266694));
#65200=CARTESIAN_POINT('Origin',(2.6,-0.928584689129192,-2.55126546543374));
#65201=CARTESIAN_POINT('Origin',(2.6,0.,0.));
#65202=CARTESIAN_POINT('Origin',(0.3,-1.29174682452695,-2.48737113059643));
#65203=CARTESIAN_POINT('',(2.6,-1.29877522499351,-2.42398079921089));
#65204=CARTESIAN_POINT('',(0.3,-1.29877522499351,-2.42398079921089));
#65205=CARTESIAN_POINT('',(1.35,-1.29877522499351,-2.42398079921089));
#65206=CARTESIAN_POINT('',(2.6,-1.315,-2.27764681195307));
#65207=CARTESIAN_POINT('',(2.6,-1.29174682452695,-2.48737113059643));
#65208=CARTESIAN_POINT('',(0.3,-1.315,-2.27764681195307));
#65209=CARTESIAN_POINT('',(0.3,-1.315,-2.27764681195307));
#65210=CARTESIAN_POINT('',(0.3,-1.29174682452695,-2.48737113059643));
#65211=CARTESIAN_POINT('Origin',(0.3,-1.3575,-2.35125897127475));
#65212=CARTESIAN_POINT('',(0.3,-1.44984133790558,-2.33676273825567));
#65213=CARTESIAN_POINT('Origin',(0.3,0.,0.));
#65214=CARTESIAN_POINT('',(0.3,-1.315,-2.27764681195307));
#65215=CARTESIAN_POINT('Origin',(0.3,-1.315,-2.27764681195307));
#65216=CARTESIAN_POINT('',(2.6,-1.44984133790558,-2.33676273825567));
#65217=CARTESIAN_POINT('',(1.35,-1.44984133790558,-2.33676273825567));
#65218=CARTESIAN_POINT('',(2.6,-1.315,-2.27764681195307));
#65219=CARTESIAN_POINT('Origin',(2.6,-1.3575,-2.35125897127475));
#65220=CARTESIAN_POINT('Origin',(2.6,0.,0.));
#65221=CARTESIAN_POINT('Origin',(0.3,-1.70404975173244,-2.22527289194396));
#65222=CARTESIAN_POINT('',(2.6,-1.69996375947638,-2.16162513319653));
#65223=CARTESIAN_POINT('',(0.3,-1.69996375947638,-2.16162513319653));
#65224=CARTESIAN_POINT('',(1.35,-1.69996375947638,-2.16162513319653));
#65225=CARTESIAN_POINT('',(2.6,-1.6905314134756,-2.01469688540291));
#65226=CARTESIAN_POINT('',(2.6,-1.70404975173244,-2.22527289194396));
#65227=CARTESIAN_POINT('',(0.3,-1.6905314134756,-2.01469688540291));
#65228=CARTESIAN_POINT('',(0.3,-1.6905314134756,-2.01469688540291));
#65229=CARTESIAN_POINT('',(0.3,-1.70404975173244,-2.22527289194396));
#65230=CARTESIAN_POINT('Origin',(0.3,-1.74516836029895,-2.07981066306802));
#65231=CARTESIAN_POINT('',(0.3,-1.83358958134509,-2.04949975535074));
#65232=CARTESIAN_POINT('Origin',(0.3,0.,0.));
#65233=CARTESIAN_POINT('',(0.3,-1.6905314134756,-2.01469688540291));
#65234=CARTESIAN_POINT('Origin',(0.3,-1.6905314134756,-2.01469688540291));
#65235=CARTESIAN_POINT('',(2.6,-1.83358958134509,-2.04949975535074));
#65236=CARTESIAN_POINT('',(1.35,-1.83358958134509,-2.04949975535074));
#65237=CARTESIAN_POINT('',(2.6,-1.6905314134756,-2.01469688540291));
#65238=CARTESIAN_POINT('Origin',(2.6,-1.74516836029895,-2.07981066306802));
#65239=CARTESIAN_POINT('Origin',(2.6,0.,0.));
#65240=CARTESIAN_POINT('Origin',(0.3,-2.06457598952232,-1.89556086251218));
#65241=CARTESIAN_POINT('',(2.6,-2.04949975535074,-1.83358958134509));
#65242=CARTESIAN_POINT('',(0.3,-2.04949975535074,-1.83358958134509));
#65243=CARTESIAN_POINT('',(1.35,-2.04949975535074,-1.83358958134509));
#65244=CARTESIAN_POINT('',(2.6,-2.01469688540291,-1.6905314134756));
#65245=CARTESIAN_POINT('',(2.6,-2.06457598952232,-1.89556086251218));
#65246=CARTESIAN_POINT('',(0.3,-2.01469688540291,-1.6905314134756));
#65247=CARTESIAN_POINT('',(0.3,-2.01469688540291,-1.6905314134756));
#65248=CARTESIAN_POINT('',(0.3,-2.06457598952232,-1.89556086251218));
#65249=CARTESIAN_POINT('Origin',(0.3,-2.07981066306803,-1.74516836029895));
#65250=CARTESIAN_POINT('',(0.3,-2.16162513319653,-1.69996375947638));
#65251=CARTESIAN_POINT('Origin',(0.3,0.,0.));
#65252=CARTESIAN_POINT('',(0.3,-2.01469688540291,-1.6905314134756));
#65253=CARTESIAN_POINT('Origin',(0.3,-2.01469688540291,-1.6905314134756));
#65254=CARTESIAN_POINT('',(2.6,-2.16162513319653,-1.69996375947638));
#65255=CARTESIAN_POINT('',(1.35,-2.16162513319653,-1.69996375947638));
#65256=CARTESIAN_POINT('',(2.6,-2.01469688540291,-1.6905314134756));
#65257=CARTESIAN_POINT('Origin',(2.6,-2.07981066306803,-1.74516836029895));
#65258=CARTESIAN_POINT('Origin',(2.6,0.,0.));
#65259=CARTESIAN_POINT('Origin',(0.3,-2.36237113059643,-1.50825317547305));
#65260=CARTESIAN_POINT('',(2.6,-2.33676273825568,-1.44984133790558));
#65261=CARTESIAN_POINT('',(0.3,-2.33676273825568,-1.44984133790558));
#65262=CARTESIAN_POINT('',(1.35,-2.33676273825567,-1.44984133790558));
#65263=CARTESIAN_POINT('',(2.6,-2.27764681195307,-1.315));
#65264=CARTESIAN_POINT('',(2.6,-2.36237113059643,-1.50825317547305));
#65265=CARTESIAN_POINT('',(0.3,-2.27764681195307,-1.315));
#65266=CARTESIAN_POINT('',(0.3,-2.27764681195307,-1.315));
#65267=CARTESIAN_POINT('',(0.3,-2.36237113059643,-1.50825317547305));
#65268=CARTESIAN_POINT('Origin',(0.3,-2.35125897127475,-1.3575));
#65269=CARTESIAN_POINT('',(0.3,-2.42398079921089,-1.29877522499351));
#65270=CARTESIAN_POINT('Origin',(0.3,0.,0.));
#65271=CARTESIAN_POINT('',(0.3,-2.27764681195307,-1.315));
#65272=CARTESIAN_POINT('Origin',(0.3,-2.27764681195307,-1.315));
#65273=CARTESIAN_POINT('',(2.6,-2.42398079921089,-1.29877522499351));
#65274=CARTESIAN_POINT('',(1.35,-2.42398079921089,-1.29877522499351));
#65275=CARTESIAN_POINT('',(2.6,-2.27764681195307,-1.315));
#65276=CARTESIAN_POINT('Origin',(2.6,-2.35125897127475,-1.3575));
#65277=CARTESIAN_POINT('Origin',(2.6,0.,0.));
#65278=CARTESIAN_POINT('Origin',(0.3,-2.58838682028483,-1.07511797891011));
#65279=CARTESIAN_POINT('',(2.6,-2.55302436781771,-1.02204039906892));
#65280=CARTESIAN_POINT('',(0.3,-2.55302436781771,-1.02204039906892));
#65281=CARTESIAN_POINT('',(1.35,-2.55302436781771,-1.02204039906892));
#65282=CARTESIAN_POINT('',(2.6,-2.47139159266694,-0.899512976946509));
#65283=CARTESIAN_POINT('',(2.6,-2.58838682028483,-1.07511797891011));
#65284=CARTESIAN_POINT('',(0.3,-2.47139159266694,-0.899512976946509));
#65285=CARTESIAN_POINT('',(0.3,-2.47139159266694,-0.899512976946509));
#65286=CARTESIAN_POINT('',(0.3,-2.58838682028483,-1.07511797891011));
#65287=CARTESIAN_POINT('Origin',(0.3,-2.55126546543374,-0.92858468912919));
#65288=CARTESIAN_POINT('',(0.3,-2.61268503523469,-0.858124062511184));
#65289=CARTESIAN_POINT('Origin',(0.3,0.,0.));
#65290=CARTESIAN_POINT('',(0.3,-2.47139159266694,-0.899512976946509));
#65291=CARTESIAN_POINT('Origin',(0.3,-2.47139159266694,-0.899512976946509));
#65292=CARTESIAN_POINT('',(2.6,-2.61268503523469,-0.858124062511184));
#65293=CARTESIAN_POINT('',(1.35,-2.61268503523469,-0.858124062511184));
#65294=CARTESIAN_POINT('',(2.6,-2.47139159266694,-0.899512976946509));
#65295=CARTESIAN_POINT('Origin',(2.6,-2.55126546543374,-0.92858468912919));
#65296=CARTESIAN_POINT('Origin',(2.6,0.,0.));
#65297=CARTESIAN_POINT('Origin',(0.3,-2.73575568622582,-0.60931586659393));
#65298=CARTESIAN_POINT('',(2.6,-2.69171364385628,-0.563185279883954));
#65299=CARTESIAN_POINT('',(0.3,-2.69171364385628,-0.563185279883954));
#65300=CARTESIAN_POINT('',(1.35,-2.69171364385628,-0.563185279883954));
#65301=CARTESIAN_POINT('',(2.6,-2.59004439042211,-0.456694707264026));
#65302=CARTESIAN_POINT('',(2.6,-2.73575568622582,-0.60931586659393));
#65303=CARTESIAN_POINT('',(0.3,-2.59004439042211,-0.456694707264026));
#65304=CARTESIAN_POINT('',(0.3,-2.59004439042211,-0.456694707264026));
#65305=CARTESIAN_POINT('',(0.3,-2.73575568622582,-0.60931586659393));
#65306=CARTESIAN_POINT('Origin',(0.3,-2.67375304942814,-0.471454802365715));
#65307=CARTESIAN_POINT('',(0.3,-2.72200415854531,-0.391399234621182));
#65308=CARTESIAN_POINT('Origin',(0.3,0.,0.));
#65309=CARTESIAN_POINT('',(0.3,-2.59004439042211,-0.456694707264026));
#65310=CARTESIAN_POINT('Origin',(0.3,-2.59004439042211,-0.456694707264026));
#65311=CARTESIAN_POINT('',(2.6,-2.72200415854531,-0.391399234621182));
#65312=CARTESIAN_POINT('',(1.35,-2.72200415854531,-0.391399234621182));
#65313=CARTESIAN_POINT('',(2.6,-2.59004439042211,-0.456694707264026));
#65314=CARTESIAN_POINT('Origin',(2.6,-2.67375304942814,-0.471454802365715));
#65315=CARTESIAN_POINT('Origin',(2.6,0.,0.));
#65316=CARTESIAN_POINT('Origin',(0.3,-2.8,-0.125));
#65317=CARTESIAN_POINT('',(2.6,-2.74861656289909,-0.0872180609552139));
#65318=CARTESIAN_POINT('',(0.3,-2.74861656289909,-0.0872180609552139));
#65319=CARTESIAN_POINT('',(1.35,-2.74861656289909,-0.0872180609552139));
#65320=CARTESIAN_POINT('',(2.6,-2.63,3.22082108175754E-16));
#65321=CARTESIAN_POINT('',(2.6,-2.8,-0.125));
#65322=CARTESIAN_POINT('',(0.3,-2.63,3.22082108175754E-16));
#65323=CARTESIAN_POINT('',(0.3,-2.63,3.22082108175754E-16));
#65324=CARTESIAN_POINT('',(0.3,-2.8,-0.125));
#65325=CARTESIAN_POINT('Origin',(0.3,-2.715,3.32491605968506E-16));
#65326=CARTESIAN_POINT('',(0.3,-2.75,-3.36777869765522E-16));
#65327=CARTESIAN_POINT('Origin',(0.3,0.,0.));
#65328=CARTESIAN_POINT('',(0.3,-2.74861656289909,0.0872180609552148));
#65329=CARTESIAN_POINT('',(0.3,-2.63,3.22082108175754E-16));
#65330=CARTESIAN_POINT('Origin',(0.3,0.,0.));
#65331=CARTESIAN_POINT('Origin',(0.3,-2.63,3.22082108175754E-16));
#65332=CARTESIAN_POINT('',(2.6,-2.74861656289909,0.0872180609552148));
#65333=CARTESIAN_POINT('',(1.35,-2.74861656289909,0.0872180609552148));
#65334=CARTESIAN_POINT('',(2.6,-2.63,3.22082108175754E-16));
#65335=CARTESIAN_POINT('Origin',(2.6,-2.715,3.32491605968506E-16));
#65336=CARTESIAN_POINT('',(2.6,-2.75,-3.36777869765522E-16));
#65337=CARTESIAN_POINT('Origin',(2.6,0.,0.));
#65338=CARTESIAN_POINT('Origin',(2.6,0.,0.));
#65339=CARTESIAN_POINT('Origin',(0.3,-2.77916773064255,0.36311392834088));
#65340=CARTESIAN_POINT('',(2.6,-2.72200415854531,0.391399234621184));
#65341=CARTESIAN_POINT('',(0.3,-2.72200415854531,0.391399234621184));
#65342=CARTESIAN_POINT('',(1.35,-2.72200415854531,0.391399234621184));
#65343=CARTESIAN_POINT('',(2.6,-2.59004439042211,0.456694707264028));
#65344=CARTESIAN_POINT('',(2.6,-2.77916773064255,0.36311392834088));
#65345=CARTESIAN_POINT('',(0.3,-2.59004439042211,0.456694707264028));
#65346=CARTESIAN_POINT('',(0.3,-2.59004439042211,0.456694707264028));
#65347=CARTESIAN_POINT('',(0.3,-2.77916773064255,0.36311392834088));
#65348=CARTESIAN_POINT('Origin',(0.3,-2.67375304942814,0.471454802365717));
#65349=CARTESIAN_POINT('',(0.3,-2.69171364385628,0.563185279883956));
#65350=CARTESIAN_POINT('Origin',(0.3,0.,0.));
#65351=CARTESIAN_POINT('',(0.3,-2.59004439042211,0.456694707264028));
#65352=CARTESIAN_POINT('Origin',(0.3,-2.59004439042211,0.456694707264028));
#65353=CARTESIAN_POINT('',(2.6,-2.69171364385628,0.563185279883956));
#65354=CARTESIAN_POINT('',(1.35,-2.69171364385628,0.563185279883956));
#65355=CARTESIAN_POINT('',(2.6,-2.59004439042211,0.456694707264028));
#65356=CARTESIAN_POINT('Origin',(2.6,-2.67375304942814,0.471454802365717));
#65357=CARTESIAN_POINT('Origin',(2.6,0.,0.));
#65358=CARTESIAN_POINT('Origin',(0.3,-2.67389185611625,0.840194823713635));
#65359=CARTESIAN_POINT('',(2.6,-2.61268503523469,0.858124062511184));
#65360=CARTESIAN_POINT('',(0.3,-2.61268503523469,0.858124062511184));
#65361=CARTESIAN_POINT('',(1.35,-2.61268503523469,0.858124062511184));
#65362=CARTESIAN_POINT('',(2.6,-2.47139159266694,0.899512976946509));
#65363=CARTESIAN_POINT('',(2.6,-2.67389185611625,0.840194823713635));
#65364=CARTESIAN_POINT('',(0.3,-2.47139159266694,0.899512976946509));
#65365=CARTESIAN_POINT('',(0.3,-2.47139159266694,0.899512976946509));
#65366=CARTESIAN_POINT('',(0.3,-2.67389185611625,0.840194823713635));
#65367=CARTESIAN_POINT('Origin',(0.3,-2.55126546543374,0.928584689129191));
#65368=CARTESIAN_POINT('',(0.3,-2.55302436781771,1.02204039906892));
#65369=CARTESIAN_POINT('Origin',(0.3,0.,0.));
#65370=CARTESIAN_POINT('',(0.3,-2.47139159266694,0.899512976946509));
#65371=CARTESIAN_POINT('Origin',(0.3,-2.47139159266694,0.899512976946509));
#65372=CARTESIAN_POINT('',(2.6,-2.55302436781771,1.02204039906892));
#65373=CARTESIAN_POINT('',(1.35,-2.55302436781771,1.02204039906893));
#65374=CARTESIAN_POINT('',(2.6,-2.47139159266694,0.899512976946509));
#65375=CARTESIAN_POINT('Origin',(2.6,-2.55126546543374,0.928584689129191));
#65376=CARTESIAN_POINT('Origin',(2.6,0.,0.));
#65377=CARTESIAN_POINT('Origin',(0.3,-2.48737113059643,1.29174682452694));
#65378=CARTESIAN_POINT('',(2.6,-2.42398079921089,1.29877522499351));
#65379=CARTESIAN_POINT('',(0.3,-2.42398079921089,1.29877522499351));
#65380=CARTESIAN_POINT('',(1.35,-2.42398079921089,1.29877522499351));
#65381=CARTESIAN_POINT('',(2.6,-2.27764681195307,1.315));
#65382=CARTESIAN_POINT('',(2.6,-2.48737113059643,1.29174682452694));
#65383=CARTESIAN_POINT('',(0.3,-2.27764681195307,1.315));
#65384=CARTESIAN_POINT('',(0.3,-2.27764681195307,1.315));
#65385=CARTESIAN_POINT('',(0.3,-2.48737113059643,1.29174682452694));
#65386=CARTESIAN_POINT('Origin',(0.3,-2.35125897127475,1.3575));
#65387=CARTESIAN_POINT('',(0.3,-2.33676273825567,1.44984133790558));
#65388=CARTESIAN_POINT('Origin',(0.3,0.,0.));
#65389=CARTESIAN_POINT('',(0.3,-2.27764681195307,1.315));
#65390=CARTESIAN_POINT('Origin',(0.3,-2.27764681195307,1.315));
#65391=CARTESIAN_POINT('',(2.6,-2.33676273825567,1.44984133790558));
#65392=CARTESIAN_POINT('',(1.35,-2.33676273825567,1.44984133790558));
#65393=CARTESIAN_POINT('',(2.6,-2.27764681195307,1.315));
#65394=CARTESIAN_POINT('Origin',(2.6,-2.35125897127475,1.3575));
#65395=CARTESIAN_POINT('Origin',(2.6,0.,0.));
#65396=CARTESIAN_POINT('Origin',(0.3,-2.22527289194396,1.70404975173244));
#65397=CARTESIAN_POINT('',(2.6,-2.16162513319653,1.69996375947638));
#65398=CARTESIAN_POINT('',(0.3,-2.16162513319653,1.69996375947638));
#65399=CARTESIAN_POINT('',(1.35,-2.16162513319653,1.69996375947638));
#65400=CARTESIAN_POINT('',(2.6,-2.01469688540291,1.6905314134756));
#65401=CARTESIAN_POINT('',(2.6,-2.22527289194396,1.70404975173244));
#65402=CARTESIAN_POINT('',(0.3,-2.01469688540291,1.6905314134756));
#65403=CARTESIAN_POINT('',(0.3,-2.01469688540291,1.6905314134756));
#65404=CARTESIAN_POINT('',(0.3,-2.22527289194396,1.70404975173244));
#65405=CARTESIAN_POINT('Origin',(0.3,-2.07981066306802,1.74516836029895));
#65406=CARTESIAN_POINT('',(0.3,-2.04949975535074,1.83358958134509));
#65407=CARTESIAN_POINT('Origin',(0.3,0.,0.));
#65408=CARTESIAN_POINT('',(0.3,-2.01469688540291,1.6905314134756));
#65409=CARTESIAN_POINT('Origin',(0.3,-2.01469688540291,1.6905314134756));
#65410=CARTESIAN_POINT('',(2.6,-2.04949975535074,1.83358958134509));
#65411=CARTESIAN_POINT('',(1.35,-2.04949975535074,1.83358958134509));
#65412=CARTESIAN_POINT('',(2.6,-2.01469688540291,1.6905314134756));
#65413=CARTESIAN_POINT('Origin',(2.6,-2.07981066306802,1.74516836029895));
#65414=CARTESIAN_POINT('Origin',(2.6,0.,0.));
#65415=CARTESIAN_POINT('Origin',(0.3,-1.89556086251218,2.06457598952232));
#65416=CARTESIAN_POINT('',(2.6,-1.83358958134509,2.04949975535074));
#65417=CARTESIAN_POINT('',(0.3,-1.83358958134509,2.04949975535074));
#65418=CARTESIAN_POINT('',(1.35,-1.83358958134509,2.04949975535074));
#65419=CARTESIAN_POINT('',(2.6,-1.6905314134756,2.01469688540291));
#65420=CARTESIAN_POINT('',(2.6,-1.89556086251218,2.06457598952232));
#65421=CARTESIAN_POINT('',(0.3,-1.6905314134756,2.01469688540291));
#65422=CARTESIAN_POINT('',(0.3,-1.6905314134756,2.01469688540291));
#65423=CARTESIAN_POINT('',(0.3,-1.89556086251218,2.06457598952232));
#65424=CARTESIAN_POINT('Origin',(0.3,-1.74516836029895,2.07981066306803));
#65425=CARTESIAN_POINT('',(0.3,-1.69996375947638,2.16162513319653));
#65426=CARTESIAN_POINT('Origin',(0.3,0.,0.));
#65427=CARTESIAN_POINT('',(0.3,-1.6905314134756,2.01469688540291));
#65428=CARTESIAN_POINT('Origin',(0.3,-1.6905314134756,2.01469688540291));
#65429=CARTESIAN_POINT('',(2.6,-1.69996375947638,2.16162513319653));
#65430=CARTESIAN_POINT('',(1.35,-1.69996375947638,2.16162513319653));
#65431=CARTESIAN_POINT('',(2.6,-1.6905314134756,2.01469688540291));
#65432=CARTESIAN_POINT('Origin',(2.6,-1.74516836029895,2.07981066306803));
#65433=CARTESIAN_POINT('Origin',(2.6,0.,0.));
#65434=CARTESIAN_POINT('Origin',(0.3,-1.50825317547305,2.36237113059643));
#65435=CARTESIAN_POINT('',(2.6,-1.44984133790558,2.33676273825568));
#65436=CARTESIAN_POINT('',(0.3,-1.44984133790558,2.33676273825568));
#65437=CARTESIAN_POINT('',(1.35,-1.44984133790558,2.33676273825568));
#65438=CARTESIAN_POINT('',(2.6,-1.315,2.27764681195307));
#65439=CARTESIAN_POINT('',(2.6,-1.50825317547305,2.36237113059643));
#65440=CARTESIAN_POINT('',(0.3,-1.315,2.27764681195307));
#65441=CARTESIAN_POINT('',(0.3,-1.315,2.27764681195307));
#65442=CARTESIAN_POINT('',(0.3,-1.50825317547305,2.36237113059643));
#65443=CARTESIAN_POINT('Origin',(0.3,-1.3575,2.35125897127475));
#65444=CARTESIAN_POINT('',(0.3,-1.29877522499351,2.42398079921089));
#65445=CARTESIAN_POINT('Origin',(0.3,0.,0.));
#65446=CARTESIAN_POINT('',(0.3,-1.315,2.27764681195307));
#65447=CARTESIAN_POINT('Origin',(0.3,-1.315,2.27764681195307));
#65448=CARTESIAN_POINT('',(2.6,-1.29877522499351,2.42398079921089));
#65449=CARTESIAN_POINT('',(1.35,-1.29877522499351,2.42398079921089));
#65450=CARTESIAN_POINT('',(2.6,-1.315,2.27764681195307));
#65451=CARTESIAN_POINT('Origin',(2.6,-1.3575,2.35125897127475));
#65452=CARTESIAN_POINT('Origin',(2.6,0.,0.));
#65453=CARTESIAN_POINT('Origin',(0.3,-1.07511797891011,2.58838682028483));
#65454=CARTESIAN_POINT('',(2.6,-1.02204039906892,2.55302436781771));
#65455=CARTESIAN_POINT('',(0.3,-1.02204039906892,2.55302436781771));
#65456=CARTESIAN_POINT('',(1.35,-1.02204039906892,2.55302436781771));
#65457=CARTESIAN_POINT('',(2.6,-0.899512976946509,2.47139159266694));
#65458=CARTESIAN_POINT('',(2.6,-1.07511797891011,2.58838682028483));
#65459=CARTESIAN_POINT('',(0.3,-0.899512976946509,2.47139159266694));
#65460=CARTESIAN_POINT('',(0.3,-0.899512976946509,2.47139159266694));
#65461=CARTESIAN_POINT('',(0.3,-1.07511797891011,2.58838682028483));
#65462=CARTESIAN_POINT('Origin',(0.3,-0.92858468912919,2.55126546543374));
#65463=CARTESIAN_POINT('',(0.3,-0.858124062511184,2.61268503523469));
#65464=CARTESIAN_POINT('Origin',(0.3,0.,0.));
#65465=CARTESIAN_POINT('',(0.3,-0.899512976946509,2.47139159266694));
#65466=CARTESIAN_POINT('Origin',(0.3,-0.899512976946509,2.47139159266694));
#65467=CARTESIAN_POINT('',(2.6,-0.858124062511184,2.61268503523469));
#65468=CARTESIAN_POINT('',(1.35,-0.858124062511184,2.61268503523469));
#65469=CARTESIAN_POINT('',(2.6,-0.899512976946509,2.47139159266694));
#65470=CARTESIAN_POINT('Origin',(2.6,-0.92858468912919,2.55126546543374));
#65471=CARTESIAN_POINT('Origin',(2.6,0.,0.));
#65472=CARTESIAN_POINT('Origin',(0.3,-0.609315866593931,2.73575568622582));
#65473=CARTESIAN_POINT('',(2.6,-0.563185279883955,2.69171364385628));
#65474=CARTESIAN_POINT('',(0.3,-0.563185279883955,2.69171364385628));
#65475=CARTESIAN_POINT('',(1.35,-0.563185279883955,2.69171364385628));
#65476=CARTESIAN_POINT('',(2.6,-0.456694707264027,2.59004439042211));
#65477=CARTESIAN_POINT('',(2.6,-0.609315866593931,2.73575568622582));
#65478=CARTESIAN_POINT('',(0.3,-0.456694707264027,2.59004439042211));
#65479=CARTESIAN_POINT('',(0.3,-0.456694707264027,2.59004439042211));
#65480=CARTESIAN_POINT('',(0.3,-0.609315866593931,2.73575568622582));
#65481=CARTESIAN_POINT('Origin',(0.3,-0.471454802365716,2.67375304942814));
#65482=CARTESIAN_POINT('',(0.3,-0.391399234621183,2.72200415854531));
#65483=CARTESIAN_POINT('Origin',(0.3,0.,0.));
#65484=CARTESIAN_POINT('',(0.3,-0.456694707264027,2.59004439042211));
#65485=CARTESIAN_POINT('Origin',(0.3,-0.456694707264027,2.59004439042211));
#65486=CARTESIAN_POINT('',(2.6,-0.391399234621183,2.72200415854531));
#65487=CARTESIAN_POINT('',(1.35,-0.391399234621183,2.72200415854531));
#65488=CARTESIAN_POINT('',(2.6,-0.456694707264027,2.59004439042211));
#65489=CARTESIAN_POINT('Origin',(2.6,-0.471454802365716,2.67375304942814));
#65490=CARTESIAN_POINT('Origin',(2.6,0.,0.));
#65491=CARTESIAN_POINT('Origin',(0.3,-0.125,2.8));
#65492=CARTESIAN_POINT('',(2.6,-0.0872180609552139,2.74861656289909));
#65493=CARTESIAN_POINT('',(0.3,-0.0872180609552139,2.74861656289909));
#65494=CARTESIAN_POINT('',(1.35,-0.0872180609552139,2.74861656289909));
#65495=CARTESIAN_POINT('',(2.6,1.61041054087877E-16,2.63));
#65496=CARTESIAN_POINT('',(2.6,-0.125,2.8));
#65497=CARTESIAN_POINT('',(0.3,1.61041054087877E-16,2.63));
#65498=CARTESIAN_POINT('',(0.3,1.61041054087877E-16,2.63));
#65499=CARTESIAN_POINT('',(0.3,-0.125,2.8));
#65500=CARTESIAN_POINT('Origin',(0.3,1.66245802984253E-16,2.715));
#65501=CARTESIAN_POINT('',(0.3,0.0872180609552142,2.74861656289909));
#65502=CARTESIAN_POINT('Origin',(0.3,0.,0.));
#65503=CARTESIAN_POINT('',(0.3,1.61041054087877E-16,2.63));
#65504=CARTESIAN_POINT('Origin',(0.3,1.61041054087877E-16,2.63));
#65505=CARTESIAN_POINT('',(2.6,0.0872180609552142,2.74861656289909));
#65506=CARTESIAN_POINT('',(1.35,0.0872180609552142,2.74861656289909));
#65507=CARTESIAN_POINT('',(2.6,1.61041054087877E-16,2.63));
#65508=CARTESIAN_POINT('Origin',(2.6,1.66245802984253E-16,2.715));
#65509=CARTESIAN_POINT('Origin',(2.6,0.,0.));
#65510=CARTESIAN_POINT('Origin',(0.3,0.363113928340879,2.77916773064255));
#65511=CARTESIAN_POINT('',(2.6,0.391399234621183,2.72200415854531));
#65512=CARTESIAN_POINT('',(0.3,0.391399234621183,2.72200415854531));
#65513=CARTESIAN_POINT('',(1.35,0.391399234621183,2.72200415854531));
#65514=CARTESIAN_POINT('',(2.6,0.456694707264027,2.59004439042211));
#65515=CARTESIAN_POINT('',(2.6,0.363113928340879,2.77916773064255));
#65516=CARTESIAN_POINT('',(0.3,0.456694707264027,2.59004439042211));
#65517=CARTESIAN_POINT('',(0.3,0.456694707264027,2.59004439042211));
#65518=CARTESIAN_POINT('',(0.3,0.363113928340879,2.77916773064255));
#65519=CARTESIAN_POINT('Origin',(0.3,0.471454802365716,2.67375304942814));
#65520=CARTESIAN_POINT('',(0.3,0.563185279883955,2.69171364385628));
#65521=CARTESIAN_POINT('Origin',(0.3,0.,0.));
#65522=CARTESIAN_POINT('',(0.3,0.456694707264027,2.59004439042211));
#65523=CARTESIAN_POINT('Origin',(0.3,0.456694707264027,2.59004439042211));
#65524=CARTESIAN_POINT('',(2.6,0.563185279883955,2.69171364385628));
#65525=CARTESIAN_POINT('',(1.35,0.563185279883955,2.69171364385628));
#65526=CARTESIAN_POINT('',(2.6,0.456694707264027,2.59004439042211));
#65527=CARTESIAN_POINT('Origin',(2.6,0.471454802365716,2.67375304942814));
#65528=CARTESIAN_POINT('Origin',(2.6,0.,0.));
#65529=CARTESIAN_POINT('Origin',(0.3,0.840194823713634,2.67389185611625));
#65530=CARTESIAN_POINT('',(2.6,0.858124062511184,2.61268503523469));
#65531=CARTESIAN_POINT('',(0.3,0.858124062511184,2.61268503523469));
#65532=CARTESIAN_POINT('',(1.35,0.858124062511184,2.61268503523469));
#65533=CARTESIAN_POINT('',(2.6,0.899512976946509,2.47139159266694));
#65534=CARTESIAN_POINT('',(2.6,0.840194823713634,2.67389185611625));
#65535=CARTESIAN_POINT('',(0.3,0.899512976946509,2.47139159266694));
#65536=CARTESIAN_POINT('',(0.3,0.899512976946509,2.47139159266694));
#65537=CARTESIAN_POINT('',(0.3,0.840194823713634,2.67389185611625));
#65538=CARTESIAN_POINT('Origin',(0.3,0.928584689129191,2.55126546543374));
#65539=CARTESIAN_POINT('',(0.3,1.02204039906892,2.55302436781771));
#65540=CARTESIAN_POINT('Origin',(0.3,0.,0.));
#65541=CARTESIAN_POINT('',(0.3,0.899512976946509,2.47139159266694));
#65542=CARTESIAN_POINT('Origin',(0.3,0.899512976946509,2.47139159266694));
#65543=CARTESIAN_POINT('',(2.6,1.02204039906892,2.55302436781771));
#65544=CARTESIAN_POINT('',(1.35,1.02204039906892,2.55302436781771));
#65545=CARTESIAN_POINT('',(2.6,0.899512976946509,2.47139159266694));
#65546=CARTESIAN_POINT('Origin',(2.6,0.928584689129191,2.55126546543374));
#65547=CARTESIAN_POINT('Origin',(2.6,0.,0.));
#65548=CARTESIAN_POINT('Origin',(0.3,1.29174682452695,2.48737113059643));
#65549=CARTESIAN_POINT('',(2.6,1.29877522499351,2.42398079921089));
#65550=CARTESIAN_POINT('',(0.3,1.29877522499351,2.42398079921089));
#65551=CARTESIAN_POINT('',(1.35,1.29877522499351,2.42398079921089));
#65552=CARTESIAN_POINT('',(2.6,1.315,2.27764681195307));
#65553=CARTESIAN_POINT('',(2.6,1.29174682452695,2.48737113059643));
#65554=CARTESIAN_POINT('',(0.3,1.315,2.27764681195307));
#65555=CARTESIAN_POINT('',(0.3,1.315,2.27764681195307));
#65556=CARTESIAN_POINT('',(0.3,1.29174682452695,2.48737113059643));
#65557=CARTESIAN_POINT('Origin',(0.3,1.3575,2.35125897127475));
#65558=CARTESIAN_POINT('',(0.3,1.44984133790558,2.33676273825567));
#65559=CARTESIAN_POINT('Origin',(0.3,0.,0.));
#65560=CARTESIAN_POINT('',(0.3,1.315,2.27764681195307));
#65561=CARTESIAN_POINT('Origin',(0.3,1.315,2.27764681195307));
#65562=CARTESIAN_POINT('',(2.6,1.44984133790558,2.33676273825567));
#65563=CARTESIAN_POINT('',(1.35,1.44984133790558,2.33676273825567));
#65564=CARTESIAN_POINT('',(2.6,1.315,2.27764681195307));
#65565=CARTESIAN_POINT('Origin',(2.6,1.3575,2.35125897127475));
#65566=CARTESIAN_POINT('Origin',(2.6,0.,0.));
#65567=CARTESIAN_POINT('Origin',(0.3,1.70404975173244,2.22527289194396));
#65568=CARTESIAN_POINT('',(2.6,1.69996375947638,2.16162513319653));
#65569=CARTESIAN_POINT('',(0.3,1.69996375947638,2.16162513319653));
#65570=CARTESIAN_POINT('',(1.35,1.69996375947638,2.16162513319653));
#65571=CARTESIAN_POINT('',(2.6,1.6905314134756,2.01469688540291));
#65572=CARTESIAN_POINT('',(2.6,1.70404975173244,2.22527289194396));
#65573=CARTESIAN_POINT('',(0.3,1.6905314134756,2.01469688540291));
#65574=CARTESIAN_POINT('',(0.3,1.6905314134756,2.01469688540291));
#65575=CARTESIAN_POINT('',(0.3,1.70404975173244,2.22527289194396));
#65576=CARTESIAN_POINT('Origin',(0.3,1.74516836029895,2.07981066306803));
#65577=CARTESIAN_POINT('',(0.3,1.83358958134509,2.04949975535074));
#65578=CARTESIAN_POINT('Origin',(0.3,0.,0.));
#65579=CARTESIAN_POINT('',(0.3,1.6905314134756,2.01469688540291));
#65580=CARTESIAN_POINT('Origin',(0.3,1.6905314134756,2.01469688540291));
#65581=CARTESIAN_POINT('',(2.6,1.83358958134509,2.04949975535074));
#65582=CARTESIAN_POINT('',(1.35,1.83358958134509,2.04949975535074));
#65583=CARTESIAN_POINT('',(2.6,1.6905314134756,2.01469688540291));
#65584=CARTESIAN_POINT('Origin',(2.6,1.74516836029895,2.07981066306803));
#65585=CARTESIAN_POINT('Origin',(2.6,0.,0.));
#65586=CARTESIAN_POINT('Origin',(0.3,2.06457598952232,1.89556086251218));
#65587=CARTESIAN_POINT('',(2.6,2.04949975535074,1.83358958134509));
#65588=CARTESIAN_POINT('',(0.3,2.04949975535074,1.83358958134509));
#65589=CARTESIAN_POINT('',(1.35,2.04949975535074,1.83358958134509));
#65590=CARTESIAN_POINT('',(2.6,2.01469688540291,1.6905314134756));
#65591=CARTESIAN_POINT('',(2.6,2.06457598952232,1.89556086251218));
#65592=CARTESIAN_POINT('',(0.3,2.01469688540291,1.6905314134756));
#65593=CARTESIAN_POINT('',(0.3,2.01469688540291,1.6905314134756));
#65594=CARTESIAN_POINT('',(0.3,2.06457598952232,1.89556086251218));
#65595=CARTESIAN_POINT('Origin',(0.3,2.07981066306803,1.74516836029895));
#65596=CARTESIAN_POINT('',(0.3,2.16162513319653,1.69996375947638));
#65597=CARTESIAN_POINT('Origin',(0.3,0.,0.));
#65598=CARTESIAN_POINT('',(0.3,2.01469688540291,1.6905314134756));
#65599=CARTESIAN_POINT('Origin',(0.3,2.01469688540291,1.6905314134756));
#65600=CARTESIAN_POINT('',(2.6,2.16162513319653,1.69996375947638));
#65601=CARTESIAN_POINT('',(1.35,2.16162513319653,1.69996375947638));
#65602=CARTESIAN_POINT('',(2.6,2.01469688540291,1.6905314134756));
#65603=CARTESIAN_POINT('Origin',(2.6,2.07981066306803,1.74516836029895));
#65604=CARTESIAN_POINT('Origin',(2.6,0.,0.));
#65605=CARTESIAN_POINT('Origin',(0.3,2.36237113059643,1.50825317547305));
#65606=CARTESIAN_POINT('',(2.6,2.33676273825567,1.44984133790558));
#65607=CARTESIAN_POINT('',(0.3,2.33676273825567,1.44984133790558));
#65608=CARTESIAN_POINT('',(1.35,2.33676273825567,1.44984133790558));
#65609=CARTESIAN_POINT('',(2.6,2.27764681195307,1.315));
#65610=CARTESIAN_POINT('',(2.6,2.36237113059643,1.50825317547305));
#65611=CARTESIAN_POINT('',(0.3,2.27764681195307,1.315));
#65612=CARTESIAN_POINT('',(0.3,2.27764681195307,1.315));
#65613=CARTESIAN_POINT('',(0.3,2.36237113059643,1.50825317547305));
#65614=CARTESIAN_POINT('Origin',(0.3,2.35125897127475,1.3575));
#65615=CARTESIAN_POINT('',(0.3,2.42398079921089,1.29877522499351));
#65616=CARTESIAN_POINT('Origin',(0.3,0.,0.));
#65617=CARTESIAN_POINT('',(0.3,2.27764681195307,1.315));
#65618=CARTESIAN_POINT('Origin',(0.3,2.27764681195307,1.315));
#65619=CARTESIAN_POINT('',(2.6,2.42398079921089,1.29877522499351));
#65620=CARTESIAN_POINT('',(1.35,2.42398079921089,1.29877522499351));
#65621=CARTESIAN_POINT('',(2.6,2.27764681195307,1.315));
#65622=CARTESIAN_POINT('Origin',(2.6,2.35125897127475,1.3575));
#65623=CARTESIAN_POINT('Origin',(2.6,0.,0.));
#65624=CARTESIAN_POINT('Origin',(0.3,2.58838682028483,1.07511797891011));
#65625=CARTESIAN_POINT('',(2.6,2.55302436781771,1.02204039906892));
#65626=CARTESIAN_POINT('',(0.3,2.55302436781771,1.02204039906892));
#65627=CARTESIAN_POINT('',(1.35,2.55302436781771,1.02204039906892));
#65628=CARTESIAN_POINT('',(2.6,2.47139159266694,0.899512976946509));
#65629=CARTESIAN_POINT('',(2.6,2.58838682028483,1.07511797891011));
#65630=CARTESIAN_POINT('',(0.3,2.47139159266694,0.899512976946509));
#65631=CARTESIAN_POINT('',(0.3,2.47139159266694,0.899512976946509));
#65632=CARTESIAN_POINT('',(0.3,2.58838682028483,1.07511797891011));
#65633=CARTESIAN_POINT('Origin',(0.3,2.55126546543374,0.92858468912919));
#65634=CARTESIAN_POINT('',(0.3,2.61268503523469,0.858124062511184));
#65635=CARTESIAN_POINT('Origin',(0.3,0.,0.));
#65636=CARTESIAN_POINT('',(0.3,2.47139159266694,0.899512976946509));
#65637=CARTESIAN_POINT('Origin',(0.3,2.47139159266694,0.899512976946509));
#65638=CARTESIAN_POINT('',(2.6,2.61268503523469,0.858124062511184));
#65639=CARTESIAN_POINT('',(1.35,2.61268503523469,0.858124062511184));
#65640=CARTESIAN_POINT('',(2.6,2.47139159266694,0.899512976946509));
#65641=CARTESIAN_POINT('Origin',(2.6,2.55126546543374,0.92858468912919));
#65642=CARTESIAN_POINT('Origin',(2.6,0.,0.));
#65643=CARTESIAN_POINT('Origin',(0.3,2.73575568622582,0.609315866593931));
#65644=CARTESIAN_POINT('',(2.6,2.69171364385628,0.563185279883955));
#65645=CARTESIAN_POINT('',(0.3,2.69171364385628,0.563185279883955));
#65646=CARTESIAN_POINT('',(1.35,2.69171364385628,0.563185279883955));
#65647=CARTESIAN_POINT('',(2.6,2.59004439042211,0.456694707264027));
#65648=CARTESIAN_POINT('',(2.6,2.73575568622582,0.609315866593931));
#65649=CARTESIAN_POINT('',(0.3,2.59004439042211,0.456694707264027));
#65650=CARTESIAN_POINT('',(0.3,2.59004439042211,0.456694707264027));
#65651=CARTESIAN_POINT('',(0.3,2.73575568622582,0.609315866593931));
#65652=CARTESIAN_POINT('Origin',(0.3,2.67375304942814,0.471454802365716));
#65653=CARTESIAN_POINT('',(0.3,2.72200415854531,0.391399234621183));
#65654=CARTESIAN_POINT('Origin',(0.3,0.,0.));
#65655=CARTESIAN_POINT('',(0.3,2.59004439042211,0.456694707264027));
#65656=CARTESIAN_POINT('Origin',(0.3,2.59004439042211,0.456694707264027));
#65657=CARTESIAN_POINT('',(2.6,2.72200415854531,0.391399234621183));
#65658=CARTESIAN_POINT('',(1.35,2.72200415854531,0.391399234621183));
#65659=CARTESIAN_POINT('',(2.6,2.59004439042211,0.456694707264027));
#65660=CARTESIAN_POINT('Origin',(2.6,2.67375304942814,0.471454802365716));
#65661=CARTESIAN_POINT('Origin',(2.6,0.,0.));
#65662=CARTESIAN_POINT('Origin',(0.3,2.8,0.125));
#65663=CARTESIAN_POINT('',(2.6,2.74861656289909,0.0872180609552145));
#65664=CARTESIAN_POINT('',(0.3,2.74861656289909,0.0872180609552145));
#65665=CARTESIAN_POINT('',(1.35,2.74861656289909,0.0872180609552145));
#65666=CARTESIAN_POINT('',(2.6,2.63,0.));
#65667=CARTESIAN_POINT('',(2.6,2.8,0.125));
#65668=CARTESIAN_POINT('',(0.3,2.63,0.));
#65669=CARTESIAN_POINT('',(0.3,2.63,0.));
#65670=CARTESIAN_POINT('',(0.3,2.8,0.125));
#65671=CARTESIAN_POINT('Origin',(0.3,2.715,0.));
#65672=CARTESIAN_POINT('',(0.3,2.74861656289909,-0.0872180609552142));
#65673=CARTESIAN_POINT('Origin',(0.3,0.,0.));
#65674=CARTESIAN_POINT('',(0.3,2.63,0.));
#65675=CARTESIAN_POINT('Origin',(0.3,2.63,0.));
#65676=CARTESIAN_POINT('',(2.6,2.74861656289909,-0.0872180609552142));
#65677=CARTESIAN_POINT('',(1.35,2.74861656289909,-0.0872180609552142));
#65678=CARTESIAN_POINT('',(2.6,2.63,0.));
#65679=CARTESIAN_POINT('Origin',(2.6,2.715,0.));
#65680=CARTESIAN_POINT('Origin',(2.6,0.,0.));
#65681=CARTESIAN_POINT('Origin',(1.32946211310777,0.,0.));
#65682=CARTESIAN_POINT('',(0.94892422621555,0.,0.));
#65683=CARTESIAN_POINT('',(1.7,-1.23357587978679,1.51069475268627E-16));
#65684=CARTESIAN_POINT('',(1.32946211310777,-0.625,-7.65404249467096E-17));
#65685=CARTESIAN_POINT('Origin',(1.7,0.,0.));
#65686=CARTESIAN_POINT('Origin',(3.,0.,1.44337567297406));
#65687=CARTESIAN_POINT('',(3.,8.83812698937422E-17,1.44337567297406));
#65688=CARTESIAN_POINT('',(3.,1.25,0.721687836487032));
#65689=CARTESIAN_POINT('',(3.,0.3125,1.26295371385231));
#65690=CARTESIAN_POINT('',(1.7,1.38777878078145E-16,1.44337567297406));
#65691=CARTESIAN_POINT('',(3.,8.83812698937422E-17,1.44337567297406));
#65692=CARTESIAN_POINT('',(1.7,1.25,0.721687836487032));
#65693=CARTESIAN_POINT('',(1.7,1.25,0.721687836487032));
#65694=CARTESIAN_POINT('',(3.,1.25,0.721687836487032));
#65695=CARTESIAN_POINT('Origin',(3.,-1.25,0.721687836487032));
#65696=CARTESIAN_POINT('',(3.,-1.25,0.721687836487032));
#65697=CARTESIAN_POINT('',(3.,-0.9375,0.90210979560879));
#65698=CARTESIAN_POINT('',(1.7,-1.25,0.721687836487032));
#65699=CARTESIAN_POINT('',(3.,-1.25,0.721687836487032));
#65700=CARTESIAN_POINT('',(1.7,8.83812698937422E-17,1.44337567297406));
#65701=CARTESIAN_POINT('Origin',(3.,-1.25,-0.721687836487032));
#65702=CARTESIAN_POINT('',(3.,-1.25,-0.721687836487032));
#65703=CARTESIAN_POINT('',(3.,-1.25,-0.360843918243516));
#65704=CARTESIAN_POINT('',(1.7,-1.25,-0.721687836487032));
#65705=CARTESIAN_POINT('',(3.,-1.25,-0.721687836487032));
#65706=CARTESIAN_POINT('',(1.7,-1.25,0.721687836487032));
#65707=CARTESIAN_POINT('Origin',(3.,-2.77555756156289E-16,-1.44337567297406));
#65708=CARTESIAN_POINT('',(3.,-2.65143809681227E-16,-1.44337567297406));
#65709=CARTESIAN_POINT('',(3.,-0.3125,-1.26295371385231));
#65710=CARTESIAN_POINT('',(1.7,-2.77555756156289E-16,-1.44337567297406));
#65711=CARTESIAN_POINT('',(3.,-2.65143809681227E-16,-1.44337567297406));
#65712=CARTESIAN_POINT('',(1.7,-1.25,-0.721687836487032));
#65713=CARTESIAN_POINT('Origin',(3.,1.25,-0.721687836487033));
#65714=CARTESIAN_POINT('',(3.,1.25,-0.721687836487033));
#65715=CARTESIAN_POINT('',(3.,0.9375,-0.902109795608791));
#65716=CARTESIAN_POINT('',(1.7,1.25,-0.721687836487033));
#65717=CARTESIAN_POINT('',(3.,1.25,-0.721687836487033));
#65718=CARTESIAN_POINT('',(1.7,-2.65143809681227E-16,-1.44337567297406));
#65719=CARTESIAN_POINT('Origin',(3.,1.25,0.721687836487032));
#65720=CARTESIAN_POINT('',(3.,1.25,0.360843918243516));
#65721=CARTESIAN_POINT('',(1.7,1.25,-0.721687836487033));
#65722=CARTESIAN_POINT('Origin',(1.7,0.,0.));
#65723=CARTESIAN_POINT('Origin',(-35.,1.1,0.));
#65724=CARTESIAN_POINT('',(-35.,-1.1,-1.34711147906209E-16));
#65725=CARTESIAN_POINT('Origin',(-35.,0.,0.));
#65726=CARTESIAN_POINT('Origin',(-34.8,0.,0.));
#65727=CARTESIAN_POINT('',(-34.8,-1.3,-1.59204083889156E-16));
#65728=CARTESIAN_POINT('Origin',(1.35,0.,0.));
#65729=CARTESIAN_POINT('',(2.7,-2.75,-3.36777869765522E-16));
#65730=CARTESIAN_POINT('Origin',(2.7,0.,0.));
#65731=CARTESIAN_POINT('',(1.35,-2.75,-3.36777869765522E-16));
#65732=CARTESIAN_POINT('',(1.35,-2.75,-3.36777869765522E-16));
#65733=CARTESIAN_POINT('Origin',(2.85,0.,0.));
#65734=CARTESIAN_POINT('',(3.,-2.45,-3.00038465791102E-16));
#65735=CARTESIAN_POINT('Origin',(3.,0.,0.));
#65736=CARTESIAN_POINT('',(2.85,-2.6,-3.18408167778312E-16));
#65737=CARTESIAN_POINT('Origin',(3.,0.,0.));
#82357=UNCERTAINTY_MEASURE_WITH_UNIT(LENGTH_MEASURE(0.01),#82385,
'DISTANCE_ACCURACY_VALUE',
'Maximum model space distance between geometric entities at asserted c
onnectivities');
#82363=UNCERTAINTY_MEASURE_WITH_UNIT(LENGTH_MEASURE(0.01),#82385,
'DISTANCE_ACCURACY_VALUE',
'Maximum model space distance between geometric entities at asserted c
onnectivities');
#82378=(
GEOMETRIC_REPRESENTATION_CONTEXT(3)
GLOBAL_UNCERTAINTY_ASSIGNED_CONTEXT((#82357))
GLOBAL_UNIT_ASSIGNED_CONTEXT((#82385,#82387,#82388))
REPRESENTATION_CONTEXT('','3D')
);
#82384=(
GEOMETRIC_REPRESENTATION_CONTEXT(3)
GLOBAL_UNCERTAINTY_ASSIGNED_CONTEXT((#82363))
GLOBAL_UNIT_ASSIGNED_CONTEXT((#82385,#82387,#82388))
REPRESENTATION_CONTEXT('','3D')
);
#82385=(
LENGTH_UNIT()
NAMED_UNIT(*)
SI_UNIT(.MILLI.,.METRE.)
);
#82387=(
NAMED_UNIT(*)
PLANE_ANGLE_UNIT()
SI_UNIT($,.RADIAN.)
);
#82388=(
NAMED_UNIT(*)
SI_UNIT($,.STERADIAN.)
SOLID_ANGLE_UNIT()
);
#82403=SHAPE_DEFINITION_REPRESENTATION(#82423,#82479);
#82423=PRODUCT_DEFINITION_SHAPE('',$,#82500);
#82479=SHAPE_REPRESENTATION('',(#32454),#82378);
#82485=PRODUCT_DEFINITION_CONTEXT('part definition',#82547,'design');
#82500=PRODUCT_DEFINITION('2026-10-20-12-38-38-109','18_DIN_912_M3x35',
#82520,#82485);
#82520=PRODUCT_DEFINITION_FORMATION('',$,#82563);
#82547=APPLICATION_CONTEXT(
'Core Data for Automotive Mechanical Design Process');
#82548=PRODUCT_CONTEXT('part definition',#82547,'mechanical');
#82563=PRODUCT('2026-10-20-12-38-38-109','18_DIN_912_M3x35',$,(#82548));
#82632=COLOUR_RGB('Black',0.12,0.14,0.17);
#82633=FILL_AREA_STYLE_COLOUR('',#82632);
#82634=FILL_AREA_STYLE('',(#82633));
#82635=SURFACE_STYLE_FILL_AREA(#82634);
#82636=SURFACE_SIDE_STYLE('',(#82635));
#82637=SURFACE_STYLE_USAGE(.BOTH.,#82636);
#82638=PRESENTATION_STYLE_ASSIGNMENT((#82637));
ENDSEC;
END-ISO-10303-21;
